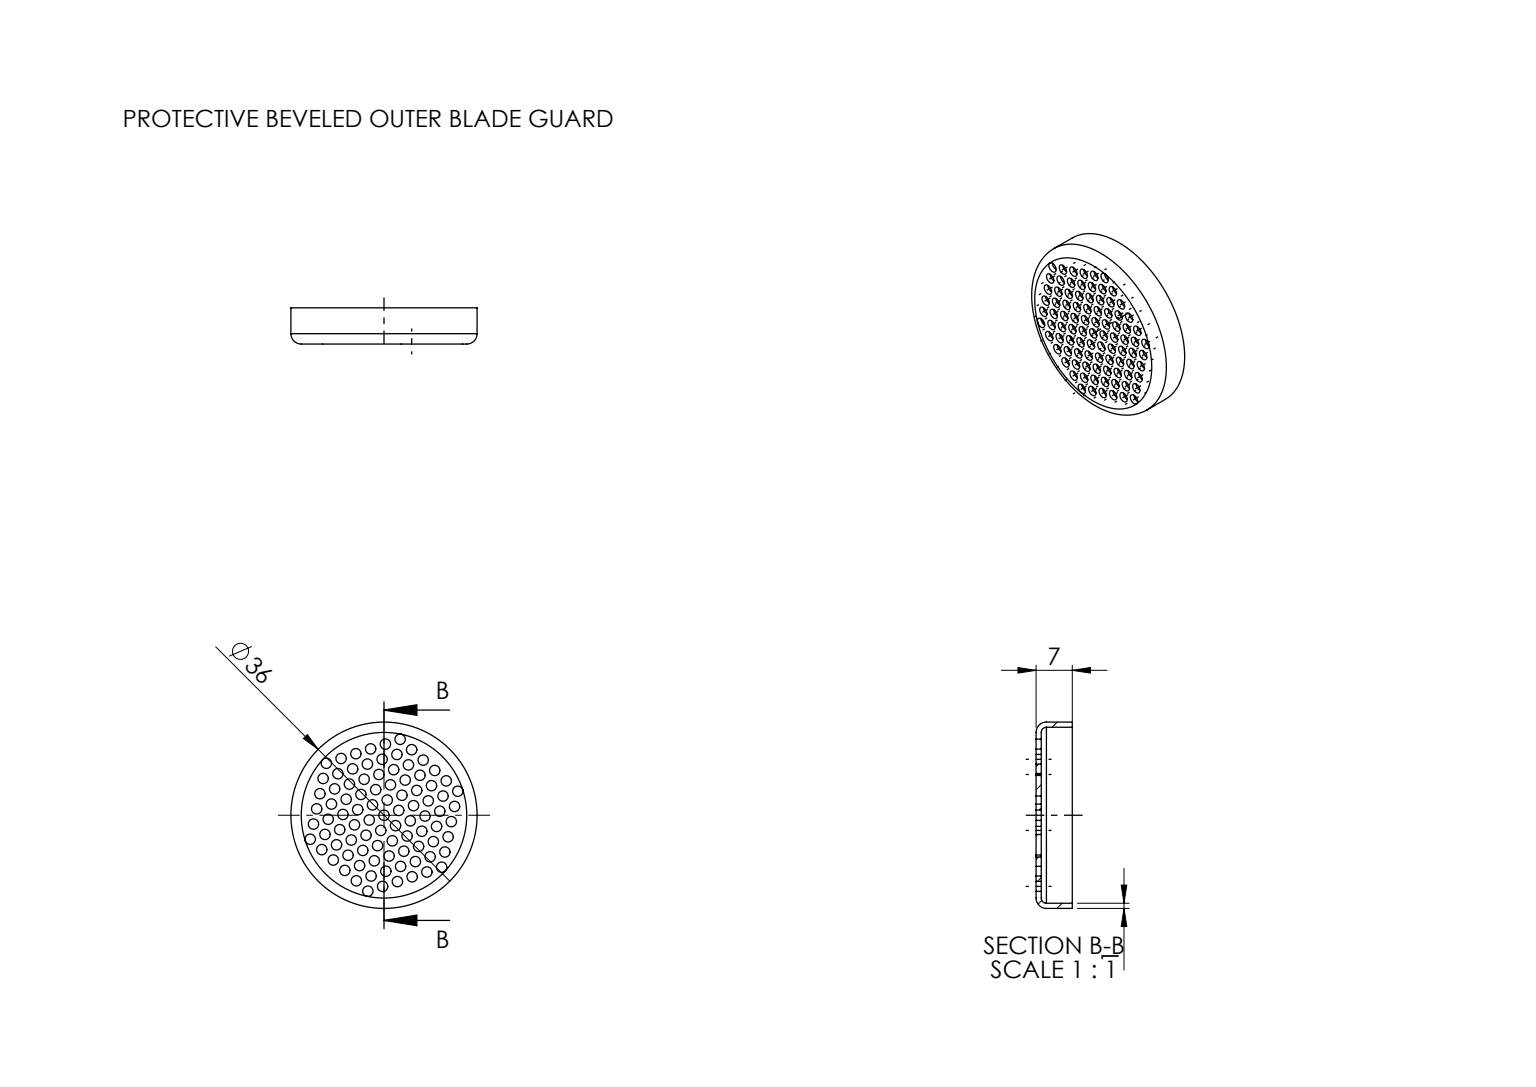
ISO-10303-21;
HEADER;
FILE_DESCRIPTION (('STEP AP214'),
    '1' );
FILE_NAME ('Protective Beveled Outer Blade Guard.step',
    '2026-10-04T08:29:30',
    ( '' ),
    ( '' ),
    'SwSTEP 2.0',
    'SolidWorks 2026',
    '' );
FILE_SCHEMA (( 'AUTOMOTIVE_DESIGN' ));
ENDSEC;

DATA;
#4=DIRECTION ( 'NONE',  ( 1.000000000000000000, 0.000000000000000000, 0.000000000000000000 ) ) ;
#5=CARTESIAN_POINT ( 'NONE',  ( 4.724371395536106633, 32.23037938972932892, 12.00000000000000000 ) ) ;
#7=VERTEX_POINT ( 'NONE', #23706 ) ;
#9=CYLINDRICAL_SURFACE ( 'NONE', #10255, 1.000000000000000000 ) ;
#10=DIRECTION ( 'NONE',  ( 1.000000000000000000, 0.000000000000000000, 0.000000000000000000 ) ) ;
#19=FACE_OUTER_BOUND ( 'NONE', #7772, .T. ) ;
#22=ORIENTED_EDGE ( 'NONE', *, *, #8423, .T. ) ;
#27=DIRECTION ( 'NONE',  ( 0.000000000000000000, 0.000000000000000000, 1.000000000000000000 ) ) ;
#33=CARTESIAN_POINT ( 'NONE',  ( -8.294006203984645609, 33.46401007850805343, 6.000000000000000000 ) ) ;
#34=ORIENTED_EDGE ( 'NONE', *, *, #3818, .T. ) ;
#39=CIRCLE ( 'NONE', #2001, 1.000000000000000000 ) ;
#40=DIRECTION ( 'NONE',  ( 1.000000000000000000, 0.000000000000000000, 0.000000000000000000 ) ) ;
#41=EDGE_LOOP ( 'NONE', ( #16818, #38380, #12394, #9835 ) ) ;
#54=DIRECTION ( 'NONE',  ( 0.000000000000000000, 0.000000000000000000, 1.000000000000000000 ) ) ;
#63=ORIENTED_EDGE ( 'NONE', *, *, #30537, .T. ) ;
#70=EDGE_CURVE ( 'NONE', #761, #15410, #872, .T. ) ;
#73=EDGE_CURVE ( 'NONE', #19744, #23095, #8006, .T. ) ;
#74=FACE_BOUND ( 'NONE', #6816, .T. ) ;
#78=DIRECTION ( 'NONE',  ( 0.000000000000000000, 0.000000000000000000, 1.000000000000000000 ) ) ;
#81=DIRECTION ( 'NONE',  ( 0.000000000000000000, 0.000000000000000000, 1.000000000000000000 ) ) ;
#83=ORIENTED_EDGE ( 'NONE', *, *, #31843, .F. ) ;
#90=ORIENTED_EDGE ( 'NONE', *, *, #14466, .T. ) ;
#91=DIRECTION ( 'NONE',  ( 1.000000000000000000, 0.000000000000000000, 0.000000000000000000 ) ) ;
#94=DIRECTION ( 'NONE',  ( 1.000000000000000000, 0.000000000000000000, 0.000000000000000000 ) ) ;
#105=CARTESIAN_POINT ( 'NONE',  ( 4.835130509701799362, 15.55077355964573904, 13.00000000000000178 ) ) ;
#107=DIRECTION ( 'NONE',  ( 1.000000000000000000, 0.000000000000000000, 0.000000000000000000 ) ) ;
#145=AXIS2_PLACEMENT_3D ( 'NONE', #32280, #11698, #11498 ) ;
#164=EDGE_CURVE ( 'NONE', #16334, #15391, #9293, .T. ) ;
#168=DIRECTION ( 'NONE',  ( 1.000000000000000000, 0.000000000000000000, 0.000000000000000000 ) ) ;
#169=EDGE_CURVE ( 'NONE', #13627, #24692, #9468, .T. ) ;
#175=DIRECTION ( 'NONE',  ( 1.000000000000000000, 0.000000000000000000, 0.000000000000000000 ) ) ;
#186=EDGE_CURVE ( 'NONE', #15751, #12988, #40137, .T. ) ;
#196=CIRCLE ( 'NONE', #16433, 1.000000000000000888 ) ;
#205=DIRECTION ( 'NONE',  ( 0.000000000000000000, 0.000000000000000000, 1.000000000000000000 ) ) ;
#206=DIRECTION ( 'NONE',  ( 0.000000000000000000, 0.000000000000000000, 1.000000000000000000 ) ) ;
#212=ORIENTED_EDGE ( 'NONE', *, *, #665, .T. ) ;
#223=ADVANCED_FACE ( 'NONE', ( #15359 ), #322, .F. ) ;
#230=DIRECTION ( 'NONE',  ( 0.000000000000000000, 0.000000000000000000, 1.000000000000000000 ) ) ;
#235=DIRECTION ( 'NONE',  ( 0.000000000000000000, 0.000000000000000000, 1.000000000000000000 ) ) ;
#237=EDGE_LOOP ( 'NONE', ( #9320, #17479 ) ) ;
#242=CARTESIAN_POINT ( 'NONE',  ( -7.559512017365658920, 19.71884705062586107, 13.00000000000000178 ) ) ;
#244=ORIENTED_EDGE ( 'NONE', *, *, #2667, .T. ) ;
#247=FACE_BOUND ( 'NONE', #237, .T. ) ;
#255=CARTESIAN_POINT ( 'NONE',  ( 5.100636323082810009, 29.29593658752792962, 6.000000000000000000 ) ) ;
#269=AXIS2_PLACEMENT_3D ( 'NONE', #36604, #30517, #27454 ) ;
#273=VECTOR ( 'NONE', #6219, 1000.000000000000000 ) ;
#274=FACE_BOUND ( 'NONE', #33600, .T. ) ;
#278=DIRECTION ( 'NONE',  ( 1.000000000000000000, 0.000000000000000000, 0.000000000000000000 ) ) ;
#292=ORIENTED_EDGE ( 'NONE', *, *, #22586, .T. ) ;
#304=DIRECTION ( 'NONE',  ( 0.000000000000000000, 0.000000000000000000, 1.000000000000000000 ) ) ;
#305=CARTESIAN_POINT ( 'NONE',  ( 9.541469607472739867, 17.40487552589537401, 13.00000000000000178 ) ) ;
#308=EDGE_LOOP ( 'NONE', ( #12738, #38655, #19382, #26352 ) ) ;
#313=ORIENTED_EDGE ( 'NONE', *, *, #4707, .F. ) ;
#314=CIRCLE ( 'NONE', #1622, 1.000000000000000888 ) ;
#317=CIRCLE ( 'NONE', #3523, 1.000000000000000000 ) ;
#318=EDGE_LOOP ( 'NONE', ( #14973, #38977, #20245, #19537 ) ) ;
#322=CYLINDRICAL_SURFACE ( 'NONE', #16452, 1.000000000000000000 ) ;
#325=CARTESIAN_POINT ( 'NONE',  ( -16.00000000000000000, 22.50000000000000711, 13.00000000000000178 ) ) ;
#327=CARTESIAN_POINT ( 'NONE',  ( 2.853166178176219425, 23.42705098312512746, 6.000000000000000000 ) ) ;
#329=DIRECTION ( 'NONE',  ( 0.000000000000000000, 0.000000000000000000, 1.000000000000000000 ) ) ;
#333=VERTEX_POINT ( 'NONE', #8869 ) ;
#337=EDGE_CURVE ( 'NONE', #7337, #4065, #33318, .T. ) ;
#342=VERTEX_POINT ( 'NONE', #31587 ) ;
#344=CARTESIAN_POINT ( 'NONE',  ( 1.247466774197339978, 28.36888560440311480, 12.00000000000000000 ) ) ;
#348=CIRCLE ( 'NONE', #38038, 1.000000000000000000 ) ;
#356=ORIENTED_EDGE ( 'NONE', *, *, #17824, .F. ) ;
#369=ORIENTED_EDGE ( 'NONE', *, *, #70, .F. ) ;
#370=EDGE_CURVE ( 'NONE', #7748, #33664, #16357, .T. ) ;
#372=CIRCLE ( 'NONE', #2976, 1.000000000000000000 ) ;
#376=FACE_OUTER_BOUND ( 'NONE', #28764, .T. ) ;
#382=CARTESIAN_POINT ( 'NONE',  ( -2.229437847141422679, 24.50739181907689712, 13.00000000000000178 ) ) ;
#389=CARTESIAN_POINT ( 'NONE',  ( 4.118671991557230072, 37.17221401100731981, 13.00000000000000178 ) ) ;
#404=CARTESIAN_POINT ( 'NONE',  ( -4.458872323573595864, 26.51478363815348160, 13.00000000000000178 ) ) ;
#405=AXIS2_PLACEMENT_3D ( 'NONE', #5623, #2190, #9079 ) ;
#406=VECTOR ( 'NONE', #32320, 1000.000000000000000 ) ;
#407=DIRECTION ( 'NONE',  ( 1.000000000000000000, 0.000000000000000000, 0.000000000000000000 ) ) ;
#418=ORIENTED_EDGE ( 'NONE', *, *, #17489, .F. ) ;
#420=DIRECTION ( 'NONE',  ( 0.000000000000000000, 0.000000000000000000, 1.000000000000000000 ) ) ;
#421=CARTESIAN_POINT ( 'NONE',  ( -7.330077540933487512, 17.71145523154927659, 6.000000000000000000 ) ) ;
#422=ADVANCED_FACE ( 'NONE', ( #9860 ), #3755, .F. ) ;
#426=CYLINDRICAL_SURFACE ( 'NONE', #11880, 1.000000000000000000 ) ;
#428=CARTESIAN_POINT ( 'NONE',  ( 4.100636323082810009, 29.29593658752792962, 12.00000000000000000 ) ) ;
#432=AXIS2_PLACEMENT_3D ( 'NONE', #3780, #28967, #7629 ) ;
#433=AXIS2_PLACEMENT_3D ( 'NONE', #15536, #27920, #20843 ) ;
#436=DIRECTION ( 'NONE',  ( 1.000000000000000000, 0.000000000000000000, 0.000000000000000000 ) ) ;
#443=FACE_OUTER_BOUND ( 'NONE', #7900, .T. ) ;
#453=DIRECTION ( 'NONE',  ( 1.000000000000000000, 0.000000000000000000, 0.000000000000000000 ) ) ;
#460=ORIENTED_EDGE ( 'NONE', *, *, #3040, .F. ) ;
#466=EDGE_CURVE ( 'NONE', #7227, #12151, #39815, .T. ) ;
#468=EDGE_CURVE ( 'NONE', #11093, #7792, #39183, .T. ) ;
#472=CYLINDRICAL_SURFACE ( 'NONE', #19490, 1.000000000000000888 ) ;
#473=FACE_BOUND ( 'NONE', #25651, .T. ) ;
#478=ADVANCED_FACE ( 'NONE', ( #13295 ), #25691, .F. ) ;
#488=VERTEX_POINT ( 'NONE', #16768 ) ;
#489=DIRECTION ( 'NONE',  ( 0.000000000000000000, 0.000000000000000000, 1.000000000000000000 ) ) ;
#495=DIRECTION ( 'NONE',  ( 0.000000000000000000, 0.000000000000000000, 1.000000000000000000 ) ) ;
#497=ORIENTED_EDGE ( 'NONE', *, *, #4457, .F. ) ;
#500=DIRECTION ( 'NONE',  ( 0.000000000000000000, 0.000000000000000000, 1.000000000000000000 ) ) ;
#502=ORIENTED_EDGE ( 'NONE', *, *, #14245, .T. ) ;
#507=ORIENTED_EDGE ( 'NONE', *, *, #21085, .T. ) ;
#516=ORIENTED_EDGE ( 'NONE', *, *, #20080, .F. ) ;
#525=DIRECTION ( 'NONE',  ( 1.000000000000000000, 0.000000000000000000, 0.000000000000000000 ) ) ;
#528=CARTESIAN_POINT ( 'NONE',  ( -6.688306800005769048, 28.52217545723006609, 12.00000000000000000 ) ) ;
#536=CYLINDRICAL_SURFACE ( 'NONE', #23712, 1.000000000000000888 ) ;
#539=ORIENTED_EDGE ( 'NONE', *, *, #1715, .F. ) ;
#548=ORIENTED_EDGE ( 'NONE', *, *, #9154, .F. ) ;
#555=AXIS2_PLACEMENT_3D ( 'NONE', #755, #4607, #4402 ) ;
#557=ORIENTED_EDGE ( 'NONE', *, *, #30997, .F. ) ;
#564=ORIENTED_EDGE ( 'NONE', *, *, #28279, .T. ) ;
#565=ORIENTED_EDGE ( 'NONE', *, *, #1592, .F. ) ;
#566=DIRECTION ( 'NONE',  ( 1.000000000000000000, 0.000000000000000000, 0.000000000000000000 ) ) ;
#567=DIRECTION ( 'NONE',  ( 0.000000000000000000, 0.000000000000000000, 1.000000000000000000 ) ) ;
#569=CYLINDRICAL_SURFACE ( 'NONE', #4551, 1.000000000000000000 ) ;
#575=EDGE_CURVE ( 'NONE', #17675, #5736, #23614, .T. ) ;
#577=LINE ( 'NONE', #40192, #36421 ) ;
#579=CARTESIAN_POINT ( 'NONE',  ( 4.100636323082810009, 29.29593658752792962, 12.00000000000000000 ) ) ;
#581=EDGE_LOOP ( 'NONE', ( #27282, #21112 ) ) ;
#600=VECTOR ( 'NONE', #21084, 1000.000000000000000 ) ;
#601=CIRCLE ( 'NONE', #23310, 1.000000000000000888 ) ;
#605=DIRECTION ( 'NONE',  ( 0.000000000000000000, 0.000000000000000000, 1.000000000000000000 ) ) ;
#607=CIRCLE ( 'NONE', #22659, 16.00000000000000000 ) ;
#609=ORIENTED_EDGE ( 'NONE', *, *, #7426, .F. ) ;
#618=EDGE_CURVE ( 'NONE', #36861, #8408, #24252, .T. ) ;
#622=DIRECTION ( 'NONE',  ( 0.000000000000000000, 0.000000000000000000, 1.000000000000000000 ) ) ;
#624=DIRECTION ( 'NONE',  ( 1.000000000000000000, 0.000000000000000000, 0.000000000000000000 ) ) ;
#625=CARTESIAN_POINT ( 'NONE',  ( 8.577540944421576441, 33.15743037285414374, 6.000000000000000000 ) ) ;
#632=VECTOR ( 'NONE', #12558, 1000.000000000000000 ) ;
#633=DIRECTION ( 'NONE',  ( 0.000000000000000000, 0.000000000000000000, 1.000000000000000000 ) ) ;
#634=VERTEX_POINT ( 'NONE', #17175 ) ;
#638=DIRECTION ( 'NONE',  ( 0.000000000000000000, 0.000000000000000000, 1.000000000000000000 ) ) ;
#641=ORIENTED_EDGE ( 'NONE', *, *, #9085, .F. ) ;
#644=FACE_BOUND ( 'NONE', #39612, .T. ) ;
#650=CARTESIAN_POINT ( 'NONE',  ( 5.064564986133971658, 13.54338174056915456, 6.000000000000000000 ) ) ;
#657=CYLINDRICAL_SURFACE ( 'NONE', #27165, 1.000000000000000888 ) ;
#664=CARTESIAN_POINT ( 'NONE',  ( 5.706335727061685681, 24.35410196624994583, 13.00000000000000178 ) ) ;
#665=EDGE_CURVE ( 'NONE', #36376, #19095, #908, .T. ) ;
#668=EDGE_CURVE ( 'NONE', #29140, #10198, #27105, .T. ) ;
#673=CARTESIAN_POINT ( 'NONE',  ( -0.01803903918367114056, 14.62372257652092422, 6.000000000000000000 ) ) ;
#682=CYLINDRICAL_SURFACE ( 'NONE', #22242, 1.000000000000000000 ) ;
#683=EDGE_CURVE ( 'NONE', #5931, #35634, #37212, .T. ) ;
#684=CIRCLE ( 'NONE', #18216, 1.000000000000000000 ) ;
#692=ORIENTED_EDGE ( 'NONE', *, *, #14157, .F. ) ;
#695=CARTESIAN_POINT ( 'NONE',  ( -3.458872323573595864, 26.51478363815348160, 13.00000000000000178 ) ) ;
#697=VERTEX_POINT ( 'NONE', #5170 ) ;
#699=CARTESIAN_POINT ( 'NONE',  ( 6.064564986133971658, 13.54338174056915456, 6.000000000000000000 ) ) ;
#708=VERTEX_POINT ( 'NONE', #2331 ) ;
#711=CARTESIAN_POINT ( 'NONE',  ( -3.118678732975735279, 7.827785988993307242, 13.00000000000000178 ) ) ;
#719=LINE ( 'NONE', #37295, #34101 ) ;
#720=ORIENTED_EDGE ( 'NONE', *, *, #23187, .T. ) ;
#730=AXIS2_PLACEMENT_3D ( 'NONE', #39640, #18124, #33167 ) ;
#732=DIRECTION ( 'NONE',  ( 1.000000000000000000, 0.000000000000000000, 0.000000000000000000 ) ) ;
#755=CARTESIAN_POINT ( 'NONE',  ( -14.26585111513660031, 17.86474508437623143, 13.00000000000000178 ) ) ;
#761=VERTEX_POINT ( 'NONE', #35848 ) ;
#775=DIRECTION ( 'NONE',  ( 0.000000000000000000, 0.000000000000000000, 1.000000000000000000 ) ) ;
#776=ORIENTED_EDGE ( 'NONE', *, *, #24265, .T. ) ;
#801=ADVANCED_FACE ( 'NONE', ( #34005 ), #24850, .F. ) ;
#808=AXIS2_PLACEMENT_3D ( 'NONE', #20811, #5557, #5361 ) ;
#810=SHAPE_DEFINITION_REPRESENTATION ( #13590, #33787 ) ;
#812=DIRECTION ( 'NONE',  ( 0.000000000000000000, 0.000000000000000000, 1.000000000000000000 ) ) ;
#820=DIRECTION ( 'NONE',  ( 0.000000000000000000, 0.000000000000000000, 1.000000000000000000 ) ) ;
#826=ORIENTED_EDGE ( 'NONE', *, *, #18908, .F. ) ;
#827=CIRCLE ( 'NONE', #29361, 1.000000000000000000 ) ;
#829=CARTESIAN_POINT ( 'NONE',  ( 8.293999462566144842, 11.53598992149257008, 12.00000000000000000 ) ) ;
#831=ORIENTED_EDGE ( 'NONE', *, *, #16332, .F. ) ;
#833=AXIS2_PLACEMENT_3D ( 'NONE', #38271, #31970, #16136 ) ;
#839=VERTEX_POINT ( 'NONE', #14916 ) ;
#843=AXIS2_PLACEMENT_3D ( 'NONE', #11726, #1991, #14371 ) ;
#844=FACE_BOUND ( 'NONE', #6698, .T. ) ;
#857=AXIS2_PLACEMENT_3D ( 'NONE', #18083, #5474, #30473 ) ;
#858=DIRECTION ( 'NONE',  ( 0.000000000000000000, 0.000000000000000000, 1.000000000000000000 ) ) ;
#867=EDGE_CURVE ( 'NONE', #37025, #33408, #28133, .T. ) ;
#869=ADVANCED_FACE ( 'NONE', ( #39494, #24256, #11671, #27502, #8821, #24652, #5564, #24058, #21208, #2722, #33618, #9020, #5768, #21014, #33423, #12264, #33812, #5960, #30362, #2529, #74, #27898, #21601, #27305, #30562, #37046, #18364, #30759, #15112, #39885, #12458, #12062, #2921, #9216, #15309, #30951, #3119, #15516, #34795, #25845, #35195, #3910, #6749, #25251, #38246, #22595, #6945, #10414, #9622, #31749, #22796, #38041, #9816, #28297, #13251, #25642, #37837, #3515, #7353, #22002, #19757, #32155, #34401, #28693, #13048, #25438, #4315, #28094, #28899, #473, #15912, #871, #31545, #274, #19352, #22392, #16310, #12659, #25051, #35004, #12856, #37646, #37445, #7153, #10210, #6552 ), #19551, .F. ) ;
#871=FACE_BOUND ( 'NONE', #16938, .T. ) ;
#872=CIRCLE ( 'NONE', #33967, 1.000000000000000000 ) ;
#880=VERTEX_POINT ( 'NONE', #4109 ) ;
#883=CARTESIAN_POINT ( 'NONE',  ( -2.229437847141422679, 24.50739181907689712, 12.00000000000000000 ) ) ;
#885=ORIENTED_EDGE ( 'NONE', *, *, #33735, .F. ) ;
#888=VERTEX_POINT ( 'NONE', #16516 ) ;
#890=CARTESIAN_POINT ( 'NONE',  ( -2.211402178667006169, 32.38366924255629442, 6.000000000000000000 ) ) ;
#893=CYLINDRICAL_SURFACE ( 'NONE', #39346, 1.000000000000000888 ) ;
#894=CIRCLE ( 'NONE', #2839, 1.000000000000000000 ) ;
#900=ORIENTED_EDGE ( 'NONE', *, *, #18324, .F. ) ;
#904=ORIENTED_EDGE ( 'NONE', *, *, #35439, .F. ) ;
#908=CIRCLE ( 'NONE', #24889, 1.000000000000000000 ) ;
#912=CIRCLE ( 'NONE', #27540, 1.000000000000000888 ) ;
#919=DIRECTION ( 'NONE',  ( 0.000000000000000000, 0.000000000000000000, 1.000000000000000000 ) ) ;
#921=EDGE_LOOP ( 'NONE', ( #7988, #20870 ) ) ;
#922=CARTESIAN_POINT ( 'NONE',  ( 5.724371395536106633, 32.23037938972932892, 13.00000000000000178 ) ) ;
#925=DIRECTION ( 'NONE',  ( 1.000000000000000000, 0.000000000000000000, 0.000000000000000000 ) ) ;
#956=VECTOR ( 'NONE', #36154, 1000.000000000000000 ) ;
#961=DIRECTION ( 'NONE',  ( 0.000000000000000000, 0.000000000000000000, 1.000000000000000000 ) ) ;
#972=ORIENTED_EDGE ( 'NONE', *, *, #34521, .F. ) ;
#974=CARTESIAN_POINT ( 'NONE',  ( -15.21736038221435727, 17.55712500267617315, 13.00000000000000178 ) ) ;
#976=STYLED_ITEM ( 'NONE', ( #32825 ), #34952 ) ;
#977=CARTESIAN_POINT ( 'NONE',  ( 13.03640989728592459, 29.14264673470096767, 13.00000000000000178 ) ) ;
#978=FACE_OUTER_BOUND ( 'NONE', #35617, .T. ) ;
#986=DIRECTION ( 'NONE',  ( 0.000000000000000000, 0.000000000000000000, 1.000000000000000000 ) ) ;
#991=LINE ( 'NONE', #7683, #5762 ) ;
#999=DIRECTION ( 'NONE',  ( 0.000000000000000000, 0.000000000000000000, 1.000000000000000000 ) ) ;
#1000=ORIENTED_EDGE ( 'NONE', *, *, #15480, .F. ) ;
#1008=ORIENTED_EDGE ( 'NONE', *, *, #2242, .F. ) ;
#1014=CIRCLE ( 'NONE', #6200, 1.000000000000000000 ) ;
#1017=PRODUCT_CONTEXT ( 'NONE', #21521, 'mechanical' ) ;
#1031=DIRECTION ( 'NONE',  ( 0.000000000000000000, 0.000000000000000000, 1.000000000000000000 ) ) ;
#1039=CIRCLE ( 'NONE', #14000, 1.000000000000000000 ) ;
#1042=AXIS2_PLACEMENT_3D ( 'NONE', #7873, #10730, #26571 ) ;
#1047=DIRECTION ( 'NONE',  ( 0.000000000000000000, 0.000000000000000000, 1.000000000000000000 ) ) ;
#1051=ORIENTED_EDGE ( 'NONE', *, *, #1452, .F. ) ;
#1053=CYLINDRICAL_SURFACE ( 'NONE', #33678, 1.000000000000000000 ) ;
#1054=CARTESIAN_POINT ( 'NONE',  ( -4.835137251120299240, 29.44922644035488446, 12.00000000000000000 ) ) ;
#1063=ORIENTED_EDGE ( 'NONE', *, *, #14261, .T. ) ;
#1066=CARTESIAN_POINT ( 'NONE',  ( -5.706342468480190000, 20.64589803375067945, 6.000000000000000000 ) ) ;
#1069=DIRECTION ( 'NONE',  ( 0.000000000000000000, 0.000000000000000000, 1.000000000000000000 ) ) ;
#1072=DIRECTION ( 'NONE',  ( 1.000000000000000000, 0.000000000000000000, 0.000000000000000000 ) ) ;
#1074=EDGE_CURVE ( 'NONE', #24243, #2749, #16921, .T. ) ;
#1076=ADVANCED_FACE ( 'NONE', ( #32767 ), #16717, .F. ) ;
#1079=ADVANCED_FACE ( 'NONE', ( #23613 ), #35403, .F. ) ;
#1081=CARTESIAN_POINT ( 'NONE',  ( 3.100636323082810009, 29.29593658752792962, 12.00000000000000000 ) ) ;
#1091=CARTESIAN_POINT ( 'NONE',  ( -3.211402178667006169, 32.38366924255629442, 13.00000000000000178 ) ) ;
#1103=ORIENTED_EDGE ( 'NONE', *, *, #25798, .F. ) ;
#1105=DIRECTION ( 'NONE',  ( 1.000000000000000000, 0.000000000000000000, 0.000000000000000000 ) ) ;
#1107=CARTESIAN_POINT ( 'NONE',  ( 0.3582258883630317636, 11.68927977431952137, 13.00000000000000178 ) ) ;
#1116=DIRECTION ( 'NONE',  ( 0.000000000000000000, 0.000000000000000000, 1.000000000000000000 ) ) ;
#1117=CYLINDRICAL_SURFACE ( 'NONE', #37924, 1.000000000000000000 ) ;
#1125=CARTESIAN_POINT ( 'NONE',  ( 0.9819609608163288872, 14.62372257652092422, 12.00000000000000000 ) ) ;
#1127=CIRCLE ( 'NONE', #32283, 1.000000000000000000 ) ;
#1149=ORIENTED_EDGE ( 'NONE', *, *, #8604, .F. ) ;
#1174=DIRECTION ( 'NONE',  ( 1.000000000000000000, 0.000000000000000000, 0.000000000000000000 ) ) ;
#1175=DIRECTION ( 'NONE',  ( 0.000000000000000000, 0.000000000000000000, 1.000000000000000000 ) ) ;
#1180=DIRECTION ( 'NONE',  ( 0.000000000000000000, 0.000000000000000000, 1.000000000000000000 ) ) ;
#1207=ORIENTED_EDGE ( 'NONE', *, *, #7249, .F. ) ;
#1213=EDGE_LOOP ( 'NONE', ( #29735, #21723 ) ) ;
#1216=AXIS2_PLACEMENT_3D ( 'NONE', #39023, #17309, #17711 ) ;
#1217=ORIENTED_EDGE ( 'NONE', *, *, #3052, .T. ) ;
#1220=CIRCLE ( 'NONE', #11606, 1.000000000000000000 ) ;
#1223=EDGE_CURVE ( 'NONE', #12698, #32913, #15840, .T. ) ;
#1226=EDGE_LOOP ( 'NONE', ( #7696, #31771 ) ) ;
#1228=DIRECTION ( 'NONE',  ( 0.000000000000000000, 0.000000000000000000, 1.000000000000000000 ) ) ;
#1229=FACE_OUTER_BOUND ( 'NONE', #33630, .T. ) ;
#1234=CARTESIAN_POINT ( 'NONE',  ( 1.494936919103933226, 34.23777120880591696, 6.000000000000000000 ) ) ;
#1240=ORIENTED_EDGE ( 'NONE', *, *, #8680, .T. ) ;
#1248=AXIS2_PLACEMENT_3D ( 'NONE', #664, #24648, #15512 ) ;
#1251=DIRECTION ( 'NONE',  ( 0.000000000000000000, 0.000000000000000000, 1.000000000000000000 ) ) ;
#1258=VERTEX_POINT ( 'NONE', #22299 ) ;
#1261=VERTEX_POINT ( 'NONE', #5321 ) ;
#1270=AXIS2_PLACEMENT_3D ( 'NONE', #37696, #19009, #9864 ) ;
#1275=DIRECTION ( 'NONE',  ( 0.000000000000000000, 0.000000000000000000, 1.000000000000000000 ) ) ;
#1287=ORIENTED_EDGE ( 'NONE', *, *, #18070, .T. ) ;
#1289=DIRECTION ( 'NONE',  ( 1.000000000000000000, 0.000000000000000000, 0.000000000000000000 ) ) ;
#1295=VECTOR ( 'NONE', #26003, 1000.000000000000000 ) ;
#1307=ORIENTED_EDGE ( 'NONE', *, *, #32309, .T. ) ;
#1310=ADVANCED_FACE ( 'NONE', ( #21162 ), #12761, .F. ) ;
#1313=EDGE_CURVE ( 'NONE', #6680, #2398, #15203, .T. ) ;
#1315=DIRECTION ( 'NONE',  ( 0.000000000000000000, 0.000000000000000000, 1.000000000000000000 ) ) ;
#1317=CARTESIAN_POINT ( 'NONE',  ( 5.458865582155095986, 18.48521636184714012, 12.00000000000000000 ) ) ;
#1324=EDGE_CURVE ( 'NONE', #26783, #13841, #26857, .T. ) ;
#1339=ORIENTED_EDGE ( 'NONE', *, *, #20945, .T. ) ;
#1350=CIRCLE ( 'NONE', #6519, 1.000000000000000888 ) ;
#1354=ORIENTED_EDGE ( 'NONE', *, *, #29827, .T. ) ;
#1356=ADVANCED_FACE ( 'NONE', ( #5514 ), #24009, .F. ) ;
#1358=EDGE_LOOP ( 'NONE', ( #33756, #22693 ) ) ;
#1361=AXIS2_PLACEMENT_3D ( 'NONE', #24804, #28254, #12412 ) ;
#1366=CARTESIAN_POINT ( 'NONE',  ( -18.00000000000000000, 22.50000000000000355, 6.000000000000000000 ) ) ;
#1367=LINE ( 'NONE', #10306, #8481 ) ;
#1376=EDGE_CURVE ( 'NONE', #18785, #40077, #26215, .T. ) ;
#1377=LINE ( 'NONE', #35710, #25357 ) ;
#1384=CARTESIAN_POINT ( 'NONE',  ( -4.118678732975735279, 7.827785988993307242, 6.000000000000000000 ) ) ;
#1396=CYLINDRICAL_SURFACE ( 'NONE', #2758, 1.000000000000000000 ) ;
#1409=ORIENTED_EDGE ( 'NONE', *, *, #22300, .F. ) ;
#1414=ORIENTED_EDGE ( 'NONE', *, *, #34847, .F. ) ;
#1419=CARTESIAN_POINT ( 'NONE',  ( 11.14716901145161643, 12.46304090461738667, 12.00000000000000000 ) ) ;
#1422=ORIENTED_EDGE ( 'NONE', *, *, #35439, .T. ) ;
#1423=LINE ( 'NONE', #23757, #26238 ) ;
#1425=EDGE_CURVE ( 'NONE', #29377, #5003, #4219, .T. ) ;
#1442=ORIENTED_EDGE ( 'NONE', *, *, #468, .T. ) ;
#1452=EDGE_CURVE ( 'NONE', #21094, #16360, #1581, .T. ) ;
#1453=DIRECTION ( 'NONE',  ( 0.000000000000000000, 0.000000000000000000, 1.000000000000000000 ) ) ;
#1454=CARTESIAN_POINT ( 'NONE',  ( 4.724371395536106633, 32.23037938972932892, 6.000000000000000000 ) ) ;
#1468=CARTESIAN_POINT ( 'NONE',  ( 16.00000000000000000, 22.50000000000000355, 12.00000000000000000 ) ) ;
#1472=CARTESIAN_POINT ( 'NONE',  ( 7.312035131040564906, 19.41226734497195849, 6.000000000000000000 ) ) ;
#1476=CIRCLE ( 'NONE', #24180, 1.000000000000000888 ) ;
#1493=DIRECTION ( 'NONE',  ( 1.000000000000000000, 0.000000000000000000, 0.000000000000000000 ) ) ;
#1495=DIRECTION ( 'NONE',  ( 0.000000000000000000, 0.000000000000000000, 1.000000000000000000 ) ) ;
#1504=ADVANCED_FACE ( 'NONE', ( #978 ), #10721, .F. ) ;
#1516=CARTESIAN_POINT ( 'NONE',  ( 0.8712018466506370462, 31.30332840660451765, 12.00000000000000000 ) ) ;
#1518=CARTESIAN_POINT ( 'NONE',  ( -7.688306800005769048, 28.52217545723006609, 12.00000000000000000 ) ) ;
#1519=CIRCLE ( 'NONE', #11910, 1.000000000000000000 ) ;
#1520=DIRECTION ( 'NONE',  ( 0.000000000000000000, 0.000000000000000000, 1.000000000000000000 ) ) ;
#1523=EDGE_CURVE ( 'NONE', #36376, #3606, #10317, .T. ) ;
#1525=CARTESIAN_POINT ( 'NONE',  ( -9.183247089818959097, 16.78440424842446532, 12.00000000000000000 ) ) ;
#1527=DIRECTION ( 'NONE',  ( 1.000000000000000000, 0.000000000000000000, 0.000000000000000000 ) ) ;
#1529=EDGE_CURVE ( 'NONE', #14246, #20723, #19724, .T. ) ;
#1531=CARTESIAN_POINT ( 'NONE',  ( 14.64210930126480115, 24.20081211342298744, 6.000000000000000000 ) ) ;
#1535=CIRCLE ( 'NONE', #24899, 1.000000000000000000 ) ;
#1553=VERTEX_POINT ( 'NONE', #25546 ) ;
#1555=CARTESIAN_POINT ( 'NONE',  ( 8.559505275947156377, 25.28115294937476065, 12.00000000000000000 ) ) ;
#1557=DIRECTION ( 'NONE',  ( 1.000000000000000000, 0.000000000000000000, 0.000000000000000000 ) ) ;
#1558=EDGE_LOOP ( 'NONE', ( #20598, #31967, #32905, #25702 ) ) ;
#1564=CARTESIAN_POINT ( 'NONE',  ( -8.577547685840080760, 11.84256962714647798, 6.000000000000000000 ) ) ;
#1573=CARTESIAN_POINT ( 'NONE',  ( 7.577540944421576441, 33.15743037285414374, 6.000000000000000000 ) ) ;
#1577=EDGE_CURVE ( 'NONE', #32176, #28480, #7460, .T. ) ;
#1581=LINE ( 'NONE', #23108, #4820 ) ;
#1582=CARTESIAN_POINT ( 'NONE',  ( -14.26585111513660031, 17.86474508437623143, 6.000000000000000000 ) ) ;
#1589=EDGE_CURVE ( 'NONE', #2436, #14685, #14573, .T. ) ;
#1590=DIRECTION ( 'NONE',  ( 0.000000000000000000, 0.000000000000000000, 1.000000000000000000 ) ) ;
#1592=EDGE_CURVE ( 'NONE', #35323, #33546, #6114, .T. ) ;
#1597=AXIS2_PLACEMENT_3D ( 'NONE', #38393, #1228, #29449 ) ;
#1602=CARTESIAN_POINT ( 'NONE',  ( -8.183247089818959097, 16.78440424842446532, 6.000000000000000000 ) ) ;
#1603=ORIENTED_EDGE ( 'NONE', *, *, #27527, .F. ) ;
#1607=ORIENTED_EDGE ( 'NONE', *, *, #31486, .F. ) ;
#1610=DIRECTION ( 'NONE',  ( 0.000000000000000000, 0.000000000000000000, 1.000000000000000000 ) ) ;
#1612=EDGE_LOOP ( 'NONE', ( #18659, #38492 ) ) ;
#1614=VERTEX_POINT ( 'NONE', #23318 ) ;
#1619=CARTESIAN_POINT ( 'NONE',  ( 6.330070799514983193, 27.28854476845134513, 13.00000000000000178 ) ) ;
#1621=DIRECTION ( 'NONE',  ( 0.000000000000000000, 0.000000000000000000, 1.000000000000000000 ) ) ;
#1622=AXIS2_PLACEMENT_3D ( 'NONE', #1740, #25900, #10676 ) ;
#1634=ORIENTED_EDGE ( 'NONE', *, *, #8604, .T. ) ;
#1640=CIRCLE ( 'NONE', #12654, 1.000000000000000000 ) ;
#1641=ORIENTED_EDGE ( 'NONE', *, *, #34748, .T. ) ;
#1646=VERTEX_POINT ( 'NONE', #32871 ) ;
#1647=ORIENTED_EDGE ( 'NONE', *, *, #28867, .T. ) ;
#1649=AXIS2_PLACEMENT_3D ( 'NONE', #3131, #12277, #15528 ) ;
#1650=CARTESIAN_POINT ( 'NONE',  ( 7.688300058587269170, 16.47782454277055564, 6.000000000000000000 ) ) ;
#1651=PLANE ( 'NONE',  #26970 ) ;
#1654=AXIS2_PLACEMENT_3D ( 'NONE', #13831, #38417, #10389 ) ;
#1665=EDGE_CURVE ( 'NONE', #12491, #1261, #14472, .T. ) ;
#1673=FACE_OUTER_BOUND ( 'NONE', #30728, .T. ) ;
#1675=CARTESIAN_POINT ( 'NONE',  ( 3.211395437248501850, 12.61633075744433796, 13.00000000000000178 ) ) ;
#1678=CIRCLE ( 'NONE', #6845, 1.000000000000000000 ) ;
#1685=DIRECTION ( 'NONE',  ( 0.000000000000000000, 0.000000000000000000, 1.000000000000000000 ) ) ;
#1690=VERTEX_POINT ( 'NONE', #18029 ) ;
#1694=DIRECTION ( 'NONE',  ( 0.000000000000000000, 0.000000000000000000, 1.000000000000000000 ) ) ;
#1708=ORIENTED_EDGE ( 'NONE', *, *, #26546, .T. ) ;
#1710=DIRECTION ( 'NONE',  ( 0.000000000000000000, 0.000000000000000000, 1.000000000000000000 ) ) ;
#1714=ORIENTED_EDGE ( 'NONE', *, *, #9208, .T. ) ;
#1715=EDGE_CURVE ( 'NONE', #40077, #18785, #11904, .T. ) ;
#1727=EDGE_CURVE ( 'NONE', #14625, #5931, #1784, .T. ) ;
#1731=DIRECTION ( 'NONE',  ( 0.000000000000000000, 0.000000000000000000, 1.000000000000000000 ) ) ;
#1735=DIRECTION ( 'NONE',  ( 0.000000000000000000, 0.000000000000000000, 1.000000000000000000 ) ) ;
#1740=CARTESIAN_POINT ( 'NONE',  ( 8.559505275947156377, 25.28115294937476065, 12.00000000000000000 ) ) ;
#1741=ORIENTED_EDGE ( 'NONE', *, *, #23042, .T. ) ;
#1750=ORIENTED_EDGE ( 'NONE', *, *, #3369, .F. ) ;
#1758=ORIENTED_EDGE ( 'NONE', *, *, #12792, .T. ) ;
#1762=DIRECTION ( 'NONE',  ( 1.000000000000000000, 0.000000000000000000, 0.000000000000000000 ) ) ;
#1768=EDGE_CURVE ( 'NONE', #8057, #24946, #11230, .T. ) ;
#1772=CIRCLE ( 'NONE', #4980, 1.000000000000000888 ) ;
#1775=DIRECTION ( 'NONE',  ( 1.000000000000000000, 0.000000000000000000, 0.000000000000000000 ) ) ;
#1776=AXIS2_PLACEMENT_3D ( 'NONE', #39774, #14803, #20706 ) ;
#1777=CIRCLE ( 'NONE', #28349, 1.000000000000000888 ) ;
#1781=CARTESIAN_POINT ( 'NONE',  ( 6.953805871968278929, 30.22298757065274444, 13.00000000000000178 ) ) ;
#1784=LINE ( 'NONE', #30215, #4083 ) ;
#1785=CARTESIAN_POINT ( 'NONE',  ( 5.348106467989403257, 35.16482219193073178, 12.00000000000000000 ) ) ;
#1798=CIRCLE ( 'NONE', #30361, 1.000000000000000000 ) ;
#1808=EDGE_LOOP ( 'NONE', ( #37828, #25664 ) ) ;
#1815=EDGE_LOOP ( 'NONE', ( #20216, #34 ) ) ;
#1821=ORIENTED_EDGE ( 'NONE', *, *, #14362, .F. ) ;
#1825=EDGE_CURVE ( 'NONE', #3811, #17784, #36546, .T. ) ;
#1826=CIRCLE ( 'NONE', #36844, 1.000000000000000000 ) ;
#1827=CARTESIAN_POINT ( 'NONE',  ( 0.7344908159097338629, 8.754836972118123839, 13.00000000000000178 ) ) ;
#1828=CARTESIAN_POINT ( 'NONE',  ( 1.853166178176219203, 23.42705098312512746, 13.00000000000000178 ) ) ;
#1833=ORIENTED_EDGE ( 'NONE', *, *, #7795, .F. ) ;
#1839=AXIS2_PLACEMENT_3D ( 'NONE', #33935, #205, #34531 ) ;
#1841=VERTEX_POINT ( 'NONE', #18819 ) ;
#1857=FACE_BOUND ( 'NONE', #16912, .T. ) ;
#1864=DIRECTION ( 'NONE',  ( 1.000000000000000000, 0.000000000000000000, 0.000000000000000000 ) ) ;
#1871=DIRECTION ( 'NONE',  ( 0.000000000000000000, 0.000000000000000000, 1.000000000000000000 ) ) ;
#1881=DIRECTION ( 'NONE',  ( 1.000000000000000000, 0.000000000000000000, 0.000000000000000000 ) ) ;
#1889=EDGE_CURVE ( 'NONE', #33038, #25337, #3370, .T. ) ;
#1892=AXIS2_PLACEMENT_3D ( 'NONE', #20958, #2671, #33765 ) ;
#1894=CARTESIAN_POINT ( 'NONE',  ( -9.183247089818959097, 16.78440424842446532, 6.000000000000000000 ) ) ;
#1900=DIRECTION ( 'NONE',  ( 0.000000000000000000, 0.000000000000000000, 1.000000000000000000 ) ) ;
#1902=EDGE_LOOP ( 'NONE', ( #18747, #37802, #33933, #21876 ) ) ;
#1916=DIRECTION ( 'NONE',  ( 0.000000000000000000, 0.000000000000000000, 1.000000000000000000 ) ) ;
#1927=AXIS2_PLACEMENT_3D ( 'NONE', #24798, #2870, #6697 ) ;
#1931=CARTESIAN_POINT ( 'NONE',  ( 0.2655024426717602637, 36.24516302788250499, 13.00000000000000178 ) ) ;
#1933=DIRECTION ( 'NONE',  ( 0.000000000000000000, 0.000000000000000000, 1.000000000000000000 ) ) ;
#1937=LINE ( 'NONE', #39095, #9264 ) ;
#1938=CARTESIAN_POINT ( 'NONE',  ( 9.293999462566146619, 11.53598992149257008, 6.000000000000000000 ) ) ;
#1940=ADVANCED_FACE ( 'NONE', ( #3569 ), #9076, .F. ) ;
#1943=DIRECTION ( 'NONE',  ( 0.000000000000000000, 0.000000000000000000, 1.000000000000000000 ) ) ;
#1944=EDGE_CURVE ( 'NONE', #30326, #6441, #36712, .T. ) ;
#1959=CYLINDRICAL_SURFACE ( 'NONE', #39979, 1.000000000000000000 ) ;
#1981=CARTESIAN_POINT ( 'NONE',  ( 4.724371395536106633, 32.23037938972932892, 6.000000000000000000 ) ) ;
#1983=AXIS2_PLACEMENT_3D ( 'NONE', #5219, #17631, #8670 ) ;
#1988=CARTESIAN_POINT ( 'NONE',  ( 3.211395437248501850, 12.61633075744433796, 6.000000000000000000 ) ) ;
#1991=DIRECTION ( 'NONE',  ( 0.000000000000000000, 0.000000000000000000, 1.000000000000000000 ) ) ;
#2001=AXIS2_PLACEMENT_3D ( 'NONE', #13298, #25694, #10874 ) ;
#2006=DIRECTION ( 'NONE',  ( 1.000000000000000000, 0.000000000000000000, 0.000000000000000000 ) ) ;
#2011=CARTESIAN_POINT ( 'NONE',  ( 3.853166178176219425, 23.42705098312512746, 6.000000000000000000 ) ) ;
#2013=AXIS2_PLACEMENT_3D ( 'NONE', #25802, #19709, #38198 ) ;
#2016=DIRECTION ( 'NONE',  ( 1.000000000000000000, 0.000000000000000000, 0.000000000000000000 ) ) ;
#2026=ORIENTED_EDGE ( 'NONE', *, *, #23863, .F. ) ;
#2030=CARTESIAN_POINT ( 'NONE',  ( 4.458865582155095986, 18.48521636184714012, 12.00000000000000000 ) ) ;
#2033=VERTEX_POINT ( 'NONE', #13103 ) ;
#2034=LINE ( 'NONE', #14414, #10664 ) ;
#2035=CARTESIAN_POINT ( 'NONE',  ( 1.358225888363031819, 11.68927977431952137, 12.00000000000000000 ) ) ;
#2036=VECTOR ( 'NONE', #34902, 1000.000000000000000 ) ;
#2037=CARTESIAN_POINT ( 'NONE',  ( -2.476907992048017260, 18.63850621467409496, 12.00000000000000000 ) ) ;
#2048=AXIS2_PLACEMENT_3D ( 'NONE', #20521, #26604, #7914 ) ;
#2051=AXIS2_PLACEMENT_3D ( 'NONE', #11019, #19958, #38239 ) ;
#2055=ORIENTED_EDGE ( 'NONE', *, *, #14868, .F. ) ;
#2060=ORIENTED_EDGE ( 'NONE', *, *, #13963, .T. ) ;
#2063=LINE ( 'NONE', #39421, #12227 ) ;
#2064=AXIS2_PLACEMENT_3D ( 'NONE', #10796, #29875, #26226 ) ;
#2066=ORIENTED_EDGE ( 'NONE', *, *, #19550, .F. ) ;
#2072=VERTEX_POINT ( 'NONE', #25493 ) ;
#2076=CARTESIAN_POINT ( 'NONE',  ( 5.953805871968278929, 30.22298757065274444, 13.00000000000000178 ) ) ;
#2082=CARTESIAN_POINT ( 'NONE',  ( 8.806975420853749625, 31.15003855377755571, 12.00000000000000000 ) ) ;
#2107=ORIENTED_EDGE ( 'NONE', *, *, #6049, .T. ) ;
#2121=VERTEX_POINT ( 'NONE', #38498 ) ;
#2125=DIRECTION ( 'NONE',  ( 1.000000000000000000, 0.000000000000000000, 0.000000000000000000 ) ) ;
#2128=DIRECTION ( 'NONE',  ( 1.000000000000000000, 0.000000000000000000, 0.000000000000000000 ) ) ;
#2137=EDGE_CURVE ( 'NONE', #24274, #12134, #28093, .T. ) ;
#2144=AXIS2_PLACEMENT_3D ( 'NONE', #27850, #9570, #15863 ) ;
#2145=DIRECTION ( 'NONE',  ( 0.000000000000000000, 0.000000000000000000, 1.000000000000000000 ) ) ;
#2151=DIRECTION ( 'NONE',  ( 1.000000000000000000, 0.000000000000000000, 0.000000000000000000 ) ) ;
#2175=MECHANICAL_DESIGN_GEOMETRIC_PRESENTATION_REPRESENTATION('',(#39801),#30067);
#2178=AXIS2_PLACEMENT_3D ( 'NONE', #34148, #25386, #25790 ) ;
#2190=DIRECTION ( 'NONE',  ( 0.000000000000000000, 0.000000000000000000, 1.000000000000000000 ) ) ;
#2191=ORIENTED_EDGE ( 'NONE', *, *, #28729, .T. ) ;
#2193=DIRECTION ( 'NONE',  ( -0.000000000000000000, -0.000000000000000000, -1.000000000000000000 ) ) ;
#2194=AXIS2_PLACEMENT_3D ( 'NONE', #5367, #11469, #14716 ) ;
#2196=EDGE_CURVE ( 'NONE', #33602, #21186, #32001, .T. ) ;
#2198=DIRECTION ( 'NONE',  ( 1.000000000000000000, 0.000000000000000000, 0.000000000000000000 ) ) ;
#2203=EDGE_CURVE ( 'NONE', #3338, #23748, #25511, .T. ) ;
#2214=ORIENTED_EDGE ( 'NONE', *, *, #1589, .T. ) ;
#2216=CARTESIAN_POINT ( 'NONE',  ( 0.3762615568374529929, 19.56555719779890978, 12.00000000000000000 ) ) ;
#2219=EDGE_CURVE ( 'NONE', #3881, #28480, #37836, .T. ) ;
#2220=EDGE_LOOP ( 'NONE', ( #38643, #904, #30878, #30669 ) ) ;
#2224=ORIENTED_EDGE ( 'NONE', *, *, #668, .F. ) ;
#2225=CARTESIAN_POINT ( 'NONE',  ( 11.03640989728592281, 29.14264673470096767, 13.00000000000000178 ) ) ;
#2242=EDGE_CURVE ( 'NONE', #634, #15741, #10881, .T. ) ;
#2244=CARTESIAN_POINT ( 'NONE',  ( -0.2474735156158440752, 16.63111439559750693, 13.00000000000000178 ) ) ;
#2271=EDGE_CURVE ( 'NONE', #14129, #36946, #30720, .T. ) ;
#2287=CYLINDRICAL_SURFACE ( 'NONE', #25446, 1.000000000000000000 ) ;
#2289=ORIENTED_EDGE ( 'NONE', *, *, #33735, .T. ) ;
#2313=LINE ( 'NONE', #29934, #33589 ) ;
#2322=VECTOR ( 'NONE', #1694, 1000.000000000000000 ) ;
#2325=CIRCLE ( 'NONE', #27599, 1.000000000000000000 ) ;
#2329=DIRECTION ( 'NONE',  ( 1.000000000000000000, 0.000000000000000000, 0.000000000000000000 ) ) ;
#2331=CARTESIAN_POINT ( 'NONE',  ( 6.440829913680675034, 10.60893893836775348, 12.00000000000000000 ) ) ;
#2339=DIRECTION ( 'NONE',  ( 0.000000000000000000, 0.000000000000000000, 1.000000000000000000 ) ) ;
#2345=EDGE_CURVE ( 'NONE', #7792, #11093, #26828, .T. ) ;
#2347=DIRECTION ( 'NONE',  ( 0.000000000000000000, 0.000000000000000000, 1.000000000000000000 ) ) ;
#2364=VECTOR ( 'NONE', #30625, 1000.000000000000000 ) ;
#2365=DIRECTION ( 'NONE',  ( 0.000000000000000000, 0.000000000000000000, 1.000000000000000000 ) ) ;
#2366=DIRECTION ( 'NONE',  ( 1.000000000000000000, 0.000000000000000000, 0.000000000000000000 ) ) ;
#2367=CARTESIAN_POINT ( 'NONE',  ( -11.39464589777670867, 26.66807349098043289, 13.00000000000000178 ) ) ;
#2378=LINE ( 'NONE', #36106, #16885 ) ;
#2384=DIRECTION ( 'NONE',  ( 1.000000000000000000, 0.000000000000000000, 0.000000000000000000 ) ) ;
#2390=VERTEX_POINT ( 'NONE', #12272 ) ;
#2392=DIRECTION ( 'NONE',  ( 1.000000000000000000, 0.000000000000000000, 0.000000000000000000 ) ) ;
#2395=EDGE_CURVE ( 'NONE', #16360, #21859, #32017, .T. ) ;
#2398=VERTEX_POINT ( 'NONE', #40095 ) ;
#2407=ORIENTED_EDGE ( 'NONE', *, *, #25596, .F. ) ;
#2408=AXIS2_PLACEMENT_3D ( 'NONE', #8042, #29380, #32027 ) ;
#2411=VERTEX_POINT ( 'NONE', #36857 ) ;
#2418=EDGE_CURVE ( 'NONE', #38453, #6898, #12465, .T. ) ;
#2419=VERTEX_POINT ( 'NONE', #22008 ) ;
#2421=FACE_OUTER_BOUND ( 'NONE', #4819, .T. ) ;
#2422=EDGE_LOOP ( 'NONE', ( #33879, #4411 ) ) ;
#2425=EDGE_CURVE ( 'NONE', #21186, #24692, #4710, .T. ) ;
#2429=CARTESIAN_POINT ( 'NONE',  ( 2.835130509701798918, 15.55077355964573904, 12.00000000000000000 ) ) ;
#2436=VERTEX_POINT ( 'NONE', #34013 ) ;
#2442=EDGE_CURVE ( 'NONE', #7574, #1553, #9426, .T. ) ;
#2443=AXIS2_PLACEMENT_3D ( 'NONE', #1981, #39536, #36496 ) ;
#2447=CIRCLE ( 'NONE', #3107, 1.000000000000000000 ) ;
#2462=AXIS2_PLACEMENT_3D ( 'NONE', #20972, #17935, #36411 ) ;
#2478=DIRECTION ( 'NONE',  ( 1.000000000000000000, 0.000000000000000000, 0.000000000000000000 ) ) ;
#2483=CARTESIAN_POINT ( 'NONE',  ( -1.247473515615844075, 16.63111439559750693, 12.00000000000000000 ) ) ;
#2494=VECTOR ( 'NONE', #31133, 1000.000000000000000 ) ;
#2498=ORIENTED_EDGE ( 'NONE', *, *, #169, .F. ) ;
#2500=VERTEX_POINT ( 'NONE', #25057 ) ;
#2501=CIRCLE ( 'NONE', #5737, 16.99999999999999645 ) ;
#2515=VERTEX_POINT ( 'NONE', #15316 ) ;
#2520=ORIENTED_EDGE ( 'NONE', *, *, #18562, .T. ) ;
#2524=AXIS2_PLACEMENT_3D ( 'NONE', #26370, #19881, #32270 ) ;
#2529=FACE_BOUND ( 'NONE', #10441, .T. ) ;
#2531=ORIENTED_EDGE ( 'NONE', *, *, #35614, .T. ) ;
#2552=AXIS2_PLACEMENT_3D ( 'NONE', #23619, #25500, #20173 ) ;
#2566=ORIENTED_EDGE ( 'NONE', *, *, #29697, .T. ) ;
#2577=CIRCLE ( 'NONE', #20095, 1.000000000000000000 ) ;
#2583=CARTESIAN_POINT ( 'NONE',  ( -12.03641663870442713, 15.85735326529964873, 6.000000000000000000 ) ) ;
#2584=AXIS2_PLACEMENT_3D ( 'NONE', #13351, #31841, #28794 ) ;
#2589=DIRECTION ( 'NONE',  ( 1.000000000000000000, 0.000000000000000000, 0.000000000000000000 ) ) ;
#2590=VERTEX_POINT ( 'NONE', #1081 ) ;
#2611=CARTESIAN_POINT ( 'NONE',  ( 16.00000000000000000, 22.50000000000000355, 11.00000000000000178 ) ) ;
#2616=EDGE_CURVE ( 'NONE', #27843, #32176, #35849, .T. ) ;
#2617=CARTESIAN_POINT ( 'NONE',  ( 3.835130509701798918, 15.55077355964573904, 13.00000000000000178 ) ) ;
#2622=AXIS2_PLACEMENT_3D ( 'NONE', #36150, #26599, #21108 ) ;
#2623=CARTESIAN_POINT ( 'NONE',  ( -3.229437847141423124, 24.50739181907689712, 6.000000000000000000 ) ) ;
#2625=DIRECTION ( 'NONE',  ( 1.000000000000000000, 0.000000000000000000, 0.000000000000000000 ) ) ;
#2634=DIRECTION ( 'NONE',  ( 0.000000000000000000, 0.000000000000000000, 1.000000000000000000 ) ) ;
#2636=CARTESIAN_POINT ( 'NONE',  ( 0.9999966292907466192, 22.50000000000031264, 12.00000000000000000 ) ) ;
#2637=CIRCLE ( 'NONE', #14959, 1.000000000000000888 ) ;
#2646=ORIENTED_EDGE ( 'NONE', *, *, #22480, .F. ) ;
#2648=CARTESIAN_POINT ( 'NONE',  ( -4.476907992048016816, 18.63850621467409496, 13.00000000000000178 ) ) ;
#2649=LINE ( 'NONE', #27428, #36051 ) ;
#2650=AXIS2_PLACEMENT_3D ( 'NONE', #7659, #38135, #7855 ) ;
#2651=LINE ( 'NONE', #9145, #3989 ) ;
#2655=DIRECTION ( 'NONE',  ( 0.000000000000000000, 0.000000000000000000, 1.000000000000000000 ) ) ;
#2667=EDGE_CURVE ( 'NONE', #12151, #36438, #3713, .T. ) ;
#2669=EDGE_CURVE ( 'NONE', #5543, #37261, #7269, .T. ) ;
#2671=DIRECTION ( 'NONE',  ( 0.000000000000000000, 0.000000000000000000, 1.000000000000000000 ) ) ;
#2673=CARTESIAN_POINT ( 'NONE',  ( 2.587660364795204782, 9.681887955242936883, 6.000000000000000000 ) ) ;
#2676=AXIS2_PLACEMENT_3D ( 'NONE', #12215, #24607, #37199 ) ;
#2681=DIRECTION ( 'NONE',  ( 0.000000000000000000, 0.000000000000000000, 1.000000000000000000 ) ) ;
#2690=DIRECTION ( 'NONE',  ( 1.000000000000000000, 0.000000000000000000, 0.000000000000000000 ) ) ;
#2691=ORIENTED_EDGE ( 'NONE', *, *, #5546, .F. ) ;
#2702=ORIENTED_EDGE ( 'NONE', *, *, #39692, .F. ) ;
#2706=ORIENTED_EDGE ( 'NONE', *, *, #17533, .T. ) ;
#2713=ORIENTED_EDGE ( 'NONE', *, *, #6496, .T. ) ;
#2716=DIRECTION ( 'NONE',  ( 1.000000000000000000, 0.000000000000000000, 0.000000000000000000 ) ) ;
#2717=EDGE_CURVE ( 'NONE', #18344, #2814, #20286, .T. ) ;
#2722=FACE_BOUND ( 'NONE', #10922, .T. ) ;
#2724=ORIENTED_EDGE ( 'NONE', *, *, #8963, .T. ) ;
#2729=CARTESIAN_POINT ( 'NONE',  ( 8.293999462566144842, 11.53598992149257008, 13.00000000000000178 ) ) ;
#2739=FACE_OUTER_BOUND ( 'NONE', #19124, .T. ) ;
#2740=ORIENTED_EDGE ( 'NONE', *, *, #36853, .F. ) ;
#2749=VERTEX_POINT ( 'NONE', #22600 ) ;
#2752=CIRCLE ( 'NONE', #18953, 1.000000000000000888 ) ;
#2753=DIRECTION ( 'NONE',  ( 1.000000000000000000, 0.000000000000000000, 0.000000000000000000 ) ) ;
#2758=AXIS2_PLACEMENT_3D ( 'NONE', #19676, #24085, #17608 ) ;
#2762=DIRECTION ( 'NONE',  ( 0.000000000000000000, 0.000000000000000000, 1.000000000000000000 ) ) ;
#2764=ORIENTED_EDGE ( 'NONE', *, *, #14758, .F. ) ;
#2766=LINE ( 'NONE', #36500, #39833 ) ;
#2769=DIRECTION ( 'NONE',  ( 0.000000000000000000, 0.000000000000000000, 1.000000000000000000 ) ) ;
#2787=CARTESIAN_POINT ( 'NONE',  ( -12.77091082532341382, 29.60251629318183575, 12.00000000000000000 ) ) ;
#2791=DIRECTION ( 'NONE',  ( 0.000000000000000000, 0.000000000000000000, 1.000000000000000000 ) ) ;
#2792=CARTESIAN_POINT ( 'NONE',  ( -6.440836655099179353, 34.39106106163288246, 6.000000000000000000 ) ) ;
#2806=CIRCLE ( 'NONE', #15759, 1.000000000000000888 ) ;
#2811=ADVANCED_FACE ( 'NONE', ( #8382 ), #2287, .F. ) ;
#2814=VERTEX_POINT ( 'NONE', #23216 ) ;
#2815=CARTESIAN_POINT ( 'NONE',  ( 11.14716901145161643, 12.46304090461738667, 12.00000000000000000 ) ) ;
#2818=AXIS2_PLACEMENT_3D ( 'NONE', #2729, #5776, #24659 ) ;
#2821=EDGE_CURVE ( 'NONE', #25235, #1258, #39735, .T. ) ;
#2823=DIRECTION ( 'NONE',  ( 0.000000000000000000, 0.000000000000000000, 1.000000000000000000 ) ) ;
#2836=DIRECTION ( 'NONE',  ( 0.000000000000000000, 0.000000000000000000, 1.000000000000000000 ) ) ;
#2839=AXIS2_PLACEMENT_3D ( 'NONE', #10969, #20310, #38790 ) ;
#2846=ORIENTED_EDGE ( 'NONE', *, *, #35816, .T. ) ;
#2849=DIRECTION ( 'NONE',  ( 0.000000000000000000, 0.000000000000000000, 1.000000000000000000 ) ) ;
#2863=ORIENTED_EDGE ( 'NONE', *, *, #8963, .F. ) ;
#2870=DIRECTION ( 'NONE',  ( 0.000000000000000000, 0.000000000000000000, 1.000000000000000000 ) ) ;
#2883=ORIENTED_EDGE ( 'NONE', *, *, #22924, .T. ) ;
#2893=EDGE_CURVE ( 'NONE', #22834, #5201, #5972, .T. ) ;
#2912=EDGE_CURVE ( 'NONE', #32554, #20514, #8595, .T. ) ;
#2914=CARTESIAN_POINT ( 'NONE',  ( -5.724378136954611840, 12.76962061027129458, 12.00000000000000000 ) ) ;
#2915=FACE_OUTER_BOUND ( 'NONE', #9754, .T. ) ;
#2918=AXIS2_PLACEMENT_3D ( 'NONE', #40147, #30817, #12322 ) ;
#2921=FACE_BOUND ( 'NONE', #19584, .T. ) ;
#2925=DIRECTION ( 'NONE',  ( 0.000000000000000000, 0.000000000000000000, 1.000000000000000000 ) ) ;
#2933=DIRECTION ( 'NONE',  ( 0.000000000000000000, 0.000000000000000000, 1.000000000000000000 ) ) ;
#2945=VECTOR ( 'NONE', #32735, 1000.000000000000000 ) ;
#2950=VERTEX_POINT ( 'NONE', #24014 ) ;
#2959=AXIS2_PLACEMENT_3D ( 'NONE', #10460, #1731, #32201 ) ;
#2960=AXIS2_PLACEMENT_3D ( 'NONE', #9346, #21726, #34132 ) ;
#2965=EDGE_CURVE ( 'NONE', #21746, #3779, #21550, .T. ) ;
#2975=DIRECTION ( 'NONE',  ( 0.000000000000000000, 0.000000000000000000, 1.000000000000000000 ) ) ;
#2976=AXIS2_PLACEMENT_3D ( 'NONE', #883, #25654, #10221 ) ;
#2977=LINE ( 'NONE', #12318, #18656 ) ;
#2983=ORIENTED_EDGE ( 'NONE', *, *, #7165, .F. ) ;
#2987=LINE ( 'NONE', #21665, #4283 ) ;
#2988=VECTOR ( 'NONE', #5876, 1000.000000000000000 ) ;
#3001=CARTESIAN_POINT ( 'NONE',  ( -18.00000000000000000, 22.50000000000000355, 13.00000000000000178 ) ) ;
#3003=ORIENTED_EDGE ( 'NONE', *, *, #7870, .T. ) ;
#3006=ORIENTED_EDGE ( 'NONE', *, *, #32881, .T. ) ;
#3013=AXIS2_PLACEMENT_3D ( 'NONE', #19573, #3337, #15932 ) ;
#3040=EDGE_CURVE ( 'NONE', #33978, #6629, #20971, .T. ) ;
#3042=ORIENTED_EDGE ( 'NONE', *, *, #18589, .T. ) ;
#3044=DIRECTION ( 'NONE',  ( 1.000000000000000000, 0.000000000000000000, 0.000000000000000000 ) ) ;
#3052=EDGE_CURVE ( 'NONE', #17743, #37305, #11845, .T. ) ;
#3056=ORIENTED_EDGE ( 'NONE', *, *, #6591, .T. ) ;
#3065=CARTESIAN_POINT ( 'NONE',  ( 2.476901250629512941, 26.36149378532653031, 13.00000000000000178 ) ) ;
#3067=LINE ( 'NONE', #6306, #19643 ) ;
#3091=FACE_BOUND ( 'NONE', #37232, .T. ) ;
#3093=VECTOR ( 'NONE', #2365, 1000.000000000000000 ) ;
#3098=ORIENTED_EDGE ( 'NONE', *, *, #3139, .F. ) ;
#3102=AXIS2_PLACEMENT_3D ( 'NONE', #15352, #6002, #15953 ) ;
#3103=EDGE_LOOP ( 'NONE', ( #12291, #25656, #14279, #8995 ) ) ;
#3107=AXIS2_PLACEMENT_3D ( 'NONE', #35785, #1453, #25282 ) ;
#3110=ORIENTED_EDGE ( 'NONE', *, *, #19798, .F. ) ;
#3119=FACE_BOUND ( 'NONE', #12939, .T. ) ;
#3123=CARTESIAN_POINT ( 'NONE',  ( -0.8712085880691411433, 13.69667159339610762, 6.000000000000000000 ) ) ;
#3131=CARTESIAN_POINT ( 'NONE',  ( -7.577547685840081648, 11.84256962714647798, 6.000000000000000000 ) ) ;
#3134=CARTESIAN_POINT ( 'NONE',  ( 1.853166178176219203, 23.42705098312512746, 12.00000000000000000 ) ) ;
#3139=EDGE_CURVE ( 'NONE', #19314, #19744, #37007, .T. ) ;
#3152=CARTESIAN_POINT ( 'NONE',  ( -5.082607396026893376, 23.58034083595207875, 12.00000000000000000 ) ) ;
#3167=DIRECTION ( 'NONE',  ( 1.000000000000000000, 0.000000000000000000, 0.000000000000000000 ) ) ;
#3173=CARTESIAN_POINT ( 'NONE',  ( -1.853172919594719970, 21.57294901687549427, 6.000000000000000000 ) ) ;
#3180=LINE ( 'NONE', #31015, #19762 ) ;
#3182=ORIENTED_EDGE ( 'NONE', *, *, #14027, .F. ) ;
#3185=CARTESIAN_POINT ( 'NONE',  ( -7.294006203984644721, 33.46401007850805343, 6.000000000000000000 ) ) ;
#3188=CARTESIAN_POINT ( 'NONE',  ( -6.953812613386785912, 14.77701242934787906, 13.00000000000000178 ) ) ;
#3220=DIRECTION ( 'NONE',  ( 0.000000000000000000, 0.000000000000000000, 1.000000000000000000 ) ) ;
#3225=ADVANCED_BREP_SHAPE_REPRESENTATION ( '', ( #34952, #24238 ), #27483 ) ;
#3245=EDGE_LOOP ( 'NONE', ( #18238, #565, #19994, #26314 ) ) ;
#3246=CIRCLE ( 'NONE', #34393, 1.000000000000000888 ) ;
#3255=EDGE_LOOP ( 'NONE', ( #22229, #30777, #5734, #23474 ) ) ;
#3257=DIRECTION ( 'NONE',  ( 1.000000000000000000, 0.000000000000000000, 0.000000000000000000 ) ) ;
#3268=EDGE_CURVE ( 'NONE', #14685, #23635, #12540, .T. ) ;
#3269=DIRECTION ( 'NONE',  ( 1.000000000000000000, 0.000000000000000000, 0.000000000000000000 ) ) ;
#3272=DIRECTION ( 'NONE',  ( 0.000000000000000000, 0.000000000000000000, 1.000000000000000000 ) ) ;
#3276=DIRECTION ( 'NONE',  ( 0.000000000000000000, 0.000000000000000000, 1.000000000000000000 ) ) ;
#3278=ORIENTED_EDGE ( 'NONE', *, *, #32069, .T. ) ;
#3283=AXIS2_PLACEMENT_3D ( 'NONE', #15758, #28149, #25101 ) ;
#3284=CARTESIAN_POINT ( 'NONE',  ( -3.853172919594720192, 21.57294901687549427, 13.00000000000000178 ) ) ;
#3285=ORIENTED_EDGE ( 'NONE', *, *, #8355, .T. ) ;
#3286=ORIENTED_EDGE ( 'NONE', *, *, #35387, .F. ) ;
#3289=FACE_BOUND ( 'NONE', #32379, .T. ) ;
#3296=CARTESIAN_POINT ( 'NONE',  ( 6.330070799514983193, 27.28854476845134513, 6.000000000000000000 ) ) ;
#3297=CARTESIAN_POINT ( 'NONE',  ( -0.6237384431625470071, 19.56555719779890978, 13.00000000000000178 ) ) ;
#3299=VECTOR ( 'NONE', #34752, 1000.000000000000000 ) ;
#3302=EDGE_LOOP ( 'NONE', ( #37285, #21030, #2107, #38367 ) ) ;
#3306=ORIENTED_EDGE ( 'NONE', *, *, #37334, .T. ) ;
#3319=CYLINDRICAL_SURFACE ( 'NONE', #23539, 1.000000000000000000 ) ;
#3320=EDGE_CURVE ( 'NONE', #16453, #32987, #8581, .T. ) ;
#3326=ORIENTED_EDGE ( 'NONE', *, *, #2667, .F. ) ;
#3337=DIRECTION ( 'NONE',  ( 0.000000000000000000, 0.000000000000000000, 1.000000000000000000 ) ) ;
#3338=VERTEX_POINT ( 'NONE', #39488 ) ;
#3343=ORIENTED_EDGE ( 'NONE', *, *, #21458, .T. ) ;
#3355=AXIS2_PLACEMENT_3D ( 'NONE', #20751, #26629, #32334 ) ;
#3363=CARTESIAN_POINT ( 'NONE',  ( -1.871208588069141143, 13.69667159339610762, 12.00000000000000000 ) ) ;
#3365=CARTESIAN_POINT ( 'NONE',  ( -7.330077540933487512, 17.71145523154927659, 12.00000000000000000 ) ) ;
#3366=DIRECTION ( 'NONE',  ( 0.000000000000000000, 0.000000000000000000, 1.000000000000000000 ) ) ;
#3369=EDGE_CURVE ( 'NONE', #35589, #19392, #32362, .T. ) ;
#3370=LINE ( 'NONE', #28153, #21600 ) ;
#3376=CARTESIAN_POINT ( 'NONE',  ( -0.7344975573282397363, 36.24516302788250499, 12.00000000000000000 ) ) ;
#3383=ORIENTED_EDGE ( 'NONE', *, *, #17215, .T. ) ;
#3384=CARTESIAN_POINT ( 'NONE',  ( 3.724371395536106188, 32.23037938972932892, 12.00000000000000000 ) ) ;
#3393=ORIENTED_EDGE ( 'NONE', *, *, #31603, .T. ) ;
#3397=VECTOR ( 'NONE', #19157, 1000.000000000000000 ) ;
#3400=CARTESIAN_POINT ( 'NONE',  ( 9.559505275947156377, 25.28115294937476065, 12.00000000000000000 ) ) ;
#3419=DIRECTION ( 'NONE',  ( 1.000000000000000000, 0.000000000000000000, 0.000000000000000000 ) ) ;
#3439=ORIENTED_EDGE ( 'NONE', *, *, #18782, .F. ) ;
#3443=DIRECTION ( 'NONE',  ( 1.000000000000000000, 0.000000000000000000, 0.000000000000000000 ) ) ;
#3445=AXIS2_PLACEMENT_3D ( 'NONE', #16456, #420, #37988 ) ;
#3446=DIRECTION ( 'NONE',  ( 0.000000000000000000, 0.000000000000000000, 1.000000000000000000 ) ) ;
#3453=DIRECTION ( 'NONE',  ( 1.000000000000000000, 0.000000000000000000, 0.000000000000000000 ) ) ;
#3455=VERTEX_POINT ( 'NONE', #25431 ) ;
#3458=EDGE_LOOP ( 'NONE', ( #36985, #9159, #21688, #29766 ) ) ;
#3466=ORIENTED_EDGE ( 'NONE', *, *, #25058, .F. ) ;
#3470=CARTESIAN_POINT ( 'NONE',  ( 1.853166178176219203, 23.42705098312512746, 6.000000000000000000 ) ) ;
#3474=AXIS2_PLACEMENT_3D ( 'NONE', #37342, #34893, #9717 ) ;
#3480=AXIS2_PLACEMENT_3D ( 'NONE', #37247, #6163, #18566 ) ;
#3488=FACE_BOUND ( 'NONE', #33804, .T. ) ;
#3489=CIRCLE ( 'NONE', #12567, 1.000000000000000000 ) ;
#3493=DIRECTION ( 'NONE',  ( 0.000000000000000000, 0.000000000000000000, 1.000000000000000000 ) ) ;
#3497=DIRECTION ( 'NONE',  ( 1.000000000000000000, 0.000000000000000000, 0.000000000000000000 ) ) ;
#3498=ADVANCED_FACE ( 'NONE', ( #28088 ), #12850, .F. ) ;
#3503=CIRCLE ( 'NONE', #4813, 1.000000000000000888 ) ;
#3506=EDGE_LOOP ( 'NONE', ( #34875, #4502, #3644, #36933 ) ) ;
#3515=FACE_BOUND ( 'NONE', #19319, .T. ) ;
#3522=ORIENTED_EDGE ( 'NONE', *, *, #9208, .F. ) ;
#3523=AXIS2_PLACEMENT_3D ( 'NONE', #30511, #31105, #18515 ) ;
#3526=CARTESIAN_POINT ( 'NONE',  ( 7.577540944421576441, 33.15743037285414374, 6.000000000000000000 ) ) ;
#3528=ORIENTED_EDGE ( 'NONE', *, *, #32151, .T. ) ;
#3529=CYLINDRICAL_SURFACE ( 'NONE', #15126, 1.000000000000000000 ) ;
#3534=LINE ( 'NONE', #12876, #36110 ) ;
#3544=DIRECTION ( 'NONE',  ( 0.000000000000000000, 0.000000000000000000, 1.000000000000000000 ) ) ;
#3545=CARTESIAN_POINT ( 'NONE',  ( 5.706335727061685681, 24.35410196624994583, 6.000000000000000000 ) ) ;
#3558=ORIENTED_EDGE ( 'NONE', *, *, #17104, .T. ) ;
#3563=CARTESIAN_POINT ( 'NONE',  ( -6.577547685840081648, 11.84256962714647798, 13.00000000000000178 ) ) ;
#3567=DIRECTION ( 'NONE',  ( 0.000000000000000000, 0.000000000000000000, 1.000000000000000000 ) ) ;
#3568=DIRECTION ( 'NONE',  ( 1.000000000000000000, 0.000000000000000000, 0.000000000000000000 ) ) ;
#3569=FACE_OUTER_BOUND ( 'NONE', #12983, .T. ) ;
#3571=CIRCLE ( 'NONE', #23681, 1.000000000000000000 ) ;
#3574=ORIENTED_EDGE ( 'NONE', *, *, #36374, .F. ) ;
#3582=ORIENTED_EDGE ( 'NONE', *, *, #16560, .F. ) ;
#3588=CIRCLE ( 'NONE', #30223, 1.000000000000000000 ) ;
#3592=ORIENTED_EDGE ( 'NONE', *, *, #38567, .F. ) ;
#3596=ORIENTED_EDGE ( 'NONE', *, *, #6124, .F. ) ;
#3606=VERTEX_POINT ( 'NONE', #28486 ) ;
#3608=DIRECTION ( 'NONE',  ( 1.000000000000000000, 0.000000000000000000, 0.000000000000000000 ) ) ;
#3610=CARTESIAN_POINT ( 'NONE',  ( 12.14716901145161643, 12.46304090461738667, 12.00000000000000000 ) ) ;
#3619=CARTESIAN_POINT ( 'NONE',  ( 9.541469607472739867, 17.40487552589537401, 13.00000000000000178 ) ) ;
#3636=DIRECTION ( 'NONE',  ( 1.000000000000000000, 0.000000000000000000, 0.000000000000000000 ) ) ;
#3637=ORIENTED_EDGE ( 'NONE', *, *, #8355, .F. ) ;
#3639=AXIS2_PLACEMENT_3D ( 'NONE', #25018, #13422, #37808 ) ;
#3644=ORIENTED_EDGE ( 'NONE', *, *, #7479, .T. ) ;
#3650=EDGE_LOOP ( 'NONE', ( #30966, #12947, #37821, #18333 ) ) ;
#3668=LINE ( 'NONE', #21750, #3299 ) ;
#3669=ADVANCED_FACE ( 'NONE', ( #28891 ), #14255, .F. ) ;
#3673=VERTEX_POINT ( 'NONE', #38440 ) ;
#3680=CARTESIAN_POINT ( 'NONE',  ( 6.688300058587269170, 16.47782454277055564, 6.000000000000000000 ) ) ;
#3684=CARTESIAN_POINT ( 'NONE',  ( -3.100643064501314328, 15.70406341247269211, 12.00000000000000000 ) ) ;
#3686=FACE_BOUND ( 'NONE', #15604, .T. ) ;
#3690=ORIENTED_EDGE ( 'NONE', *, *, #16352, .F. ) ;
#3694=DIRECTION ( 'NONE',  ( 0.000000000000000000, 0.000000000000000000, 1.000000000000000000 ) ) ;
#3703=ORIENTED_EDGE ( 'NONE', *, *, #1825, .T. ) ;
#3709=CARTESIAN_POINT ( 'NONE',  ( 0.000000000000000000, 22.50000000000000355, 12.00000000000000000 ) ) ;
#3713=LINE ( 'NONE', #673, #3397 ) ;
#3715=CIRCLE ( 'NONE', #40028, 1.000000000000000000 ) ;
#3720=CARTESIAN_POINT ( 'NONE',  ( -14.64211604268330902, 20.79918788657763429, 6.000000000000000000 ) ) ;
#3723=CARTESIAN_POINT ( 'NONE',  ( -0.2474735156158440752, 16.63111439559750693, 12.00000000000000000 ) ) ;
#3724=ORIENTED_EDGE ( 'NONE', *, *, #3369, .T. ) ;
#3729=FACE_OUTER_BOUND ( 'NONE', #38613, .T. ) ;
#3730=AXIS2_PLACEMENT_3D ( 'NONE', #3545, #34433, #11005 ) ;
#3734=CARTESIAN_POINT ( 'NONE',  ( -7.935776944912362296, 22.65328985282726393, 12.00000000000000000 ) ) ;
#3736=VERTEX_POINT ( 'NONE', #36002 ) ;
#3739=FACE_OUTER_BOUND ( 'NONE', #16500, .T. ) ;
#3740=CARTESIAN_POINT ( 'NONE',  ( -13.64211604268330724, 20.79918788657763429, 12.00000000000000000 ) ) ;
#3745=ORIENTED_EDGE ( 'NONE', *, *, #30869, .T. ) ;
#3753=CIRCLE ( 'NONE', #1839, 1.000000000000000000 ) ;
#3755=CYLINDRICAL_SURFACE ( 'NONE', #35944, 1.000000000000000888 ) ;
#3758=EDGE_CURVE ( 'NONE', #35978, #17743, #14367, .T. ) ;
#3759=ORIENTED_EDGE ( 'NONE', *, *, #15975, .T. ) ;
#3761=CARTESIAN_POINT ( 'NONE',  ( -5.724378136954611840, 12.76962061027129458, 13.00000000000000178 ) ) ;
#3764=DIRECTION ( 'NONE',  ( 0.000000000000000000, 0.000000000000000000, 1.000000000000000000 ) ) ;
#3765=CARTESIAN_POINT ( 'NONE',  ( 9.806975420853749625, 31.15003855377755571, 12.00000000000000000 ) ) ;
#3768=ORIENTED_EDGE ( 'NONE', *, *, #11787, .T. ) ;
#3779=VERTEX_POINT ( 'NONE', #1468 ) ;
#3780=CARTESIAN_POINT ( 'NONE',  ( 7.312035131040564906, 19.41226734497195849, 13.00000000000000178 ) ) ;
#3789=DIRECTION ( 'NONE',  ( -0.000000000000000000, -0.000000000000000000, -1.000000000000000000 ) ) ;
#3800=EDGE_CURVE ( 'NONE', #11948, #35485, #26012, .T. ) ;
#3805=ORIENTED_EDGE ( 'NONE', *, *, #28700, .T. ) ;
#3811=VERTEX_POINT ( 'NONE', #35798 ) ;
#3813=DIRECTION ( 'NONE',  ( 1.000000000000000000, 0.000000000000000000, 0.000000000000000000 ) ) ;
#3816=LINE ( 'NONE', #10930, #2036 ) ;
#3818=EDGE_CURVE ( 'NONE', #25818, #342, #29272, .T. ) ;
#3822=ORIENTED_EDGE ( 'NONE', *, *, #10861, .F. ) ;
#3831=DIRECTION ( 'NONE',  ( 1.000000000000000000, 0.000000000000000000, 0.000000000000000000 ) ) ;
#3841=CIRCLE ( 'NONE', #29781, 1.000000000000000000 ) ;
#3842=CARTESIAN_POINT ( 'NONE',  ( 5.440829913680675034, 10.60893893836775348, 12.00000000000000000 ) ) ;
#3851=ORIENTED_EDGE ( 'NONE', *, *, #18911, .T. ) ;
#3856=VERTEX_POINT ( 'NONE', #17919 ) ;
#3859=CARTESIAN_POINT ( 'NONE',  ( 0.6056960332696259552, 17.55816537872232530, 12.00000000000000000 ) ) ;
#3874=CIRCLE ( 'NONE', #15565, 1.000000000000000888 ) ;
#3875=CARTESIAN_POINT ( 'NONE',  ( -9.917741276437942233, 30.52956727630665057, 13.00000000000000178 ) ) ;
#3881=VERTEX_POINT ( 'NONE', #2076 ) ;
#3885=FACE_BOUND ( 'NONE', #13805, .T. ) ;
#3887=DIRECTION ( 'NONE',  ( 1.000000000000000000, 0.000000000000000000, 0.000000000000000000 ) ) ;
#3897=ADVANCED_FACE ( 'NONE', ( #14861 ), #21152, .F. ) ;
#3907=FACE_OUTER_BOUND ( 'NONE', #11561, .T. ) ;
#3910=FACE_BOUND ( 'NONE', #38784, .T. ) ;
#3942=ORIENTED_EDGE ( 'NONE', *, *, #9008, .T. ) ;
#3958=LINE ( 'NONE', #3173, #22390 ) ;
#3963=CARTESIAN_POINT ( 'NONE',  ( 9.806975420853749625, 31.15003855377755571, 13.00000000000000178 ) ) ;
#3966=DIRECTION ( 'NONE',  ( 1.000000000000000000, 0.000000000000000000, 0.000000000000000000 ) ) ;
#3968=CIRCLE ( 'NONE', #4647, 1.000000000000000000 ) ;
#3989=VECTOR ( 'NONE', #39816, 1000.000000000000000 ) ;
#3991=ORIENTED_EDGE ( 'NONE', *, *, #4938, .T. ) ;
#4003=DIRECTION ( 'NONE',  ( 0.000000000000000000, 0.000000000000000000, 1.000000000000000000 ) ) ;
#4005=DIRECTION ( 'NONE',  ( 0.000000000000000000, 0.000000000000000000, 1.000000000000000000 ) ) ;
#4009=DIRECTION ( 'NONE',  ( 0.000000000000000000, 0.000000000000000000, 1.000000000000000000 ) ) ;
#4019=CARTESIAN_POINT ( 'NONE',  ( 3.118671991557230516, 37.17221401100731981, 12.00000000000000000 ) ) ;
#4031=CARTESIAN_POINT ( 'NONE',  ( -6.330077540933487512, 17.71145523154927659, 12.00000000000000000 ) ) ;
#4038=CARTESIAN_POINT ( 'NONE',  ( 9.788939752379329562, 23.27376113029817617, 12.00000000000000000 ) ) ;
#4046=ORIENTED_EDGE ( 'NONE', *, *, #26108, .T. ) ;
#4059=CARTESIAN_POINT ( 'NONE',  ( -1.358232629781535916, 33.31072022568110924, 12.00000000000000000 ) ) ;
#4063=AXIS2_PLACEMENT_3D ( 'NONE', #33026, #24260, #20823 ) ;
#4065=VERTEX_POINT ( 'NONE', #6300 ) ;
#4068=EDGE_CURVE ( 'NONE', #21075, #29599, #23449, .T. ) ;
#4078=CYLINDRICAL_SURFACE ( 'NONE', #35400, 1.000000000000000000 ) ;
#4083=VECTOR ( 'NONE', #14776, 1000.000000000000000 ) ;
#4092=ORIENTED_EDGE ( 'NONE', *, *, #20964, .T. ) ;
#4094=ADVANCED_FACE ( 'NONE', ( #19 ), #9163, .F. ) ;
#4109=CARTESIAN_POINT ( 'NONE',  ( -3.326590493086956091, 6.849639119454676184, 13.00000000000000178 ) ) ;
#4126=ORIENTED_EDGE ( 'NONE', *, *, #23455, .T. ) ;
#4132=VERTEX_POINT ( 'NONE', #12999 ) ;
#4151=EDGE_CURVE ( 'NONE', #33408, #33800, #28245, .T. ) ;
#4153=CIRCLE ( 'NONE', #4063, 1.000000000000000888 ) ;
#4155=CIRCLE ( 'NONE', #11319, 1.000000000000000000 ) ;
#4166=CARTESIAN_POINT ( 'NONE',  ( 3.118671991557230516, 37.17221401100731981, 12.00000000000000000 ) ) ;
#4172=AXIS2_PLACEMENT_3D ( 'NONE', #25748, #13358, #13966 ) ;
#4177=EDGE_LOOP ( 'NONE', ( #17371, #16830, #29515, #18095 ) ) ;
#4182=CARTESIAN_POINT ( 'NONE',  ( -4.348113209407908464, 9.835177808069893501, 6.000000000000000000 ) ) ;
#4185=AXIS2_PLACEMENT_3D ( 'NONE', #829, #13617, #19116 ) ;
#4197=EDGE_CURVE ( 'NONE', #21746, #4655, #32473, .T. ) ;
#4200=ORIENTED_EDGE ( 'NONE', *, *, #8165, .T. ) ;
#4203=DIRECTION ( 'NONE',  ( 1.000000000000000000, 0.000000000000000000, 0.000000000000000000 ) ) ;
#4207=ORIENTED_EDGE ( 'NONE', *, *, #35998, .F. ) ;
#4217=( GEOMETRIC_REPRESENTATION_CONTEXT ( 3 ) GLOBAL_UNCERTAINTY_ASSIGNED_CONTEXT ( ( #35587 ) ) GLOBAL_UNIT_ASSIGNED_CONTEXT ( ( #35664, #19821, #20224 ) ) REPRESENTATION_CONTEXT ( 'NONE', 'WORKASPACE' ) );
#4219=LINE ( 'NONE', #29001, #24282 ) ;
#4220=DIRECTION ( 'NONE',  ( 0.000000000000000000, 0.000000000000000000, 1.000000000000000000 ) ) ;
#4230=CARTESIAN_POINT ( 'NONE',  ( -5.706342468480190000, 20.64589803375067945, 12.00000000000000000 ) ) ;
#4233=DIRECTION ( 'NONE',  ( 0.000000000000000000, 0.000000000000000000, 1.000000000000000000 ) ) ;
#4244=DIRECTION ( 'NONE',  ( 1.000000000000000000, 0.000000000000000000, 0.000000000000000000 ) ) ;
#4254=AXIS2_PLACEMENT_3D ( 'NONE', #38085, #28741, #23458 ) ;
#4263=ORIENTED_EDGE ( 'NONE', *, *, #24570, .F. ) ;
#4265=CARTESIAN_POINT ( 'NONE',  ( 9.541469607472739867, 17.40487552589537401, 12.00000000000000000 ) ) ;
#4266=CYLINDRICAL_SURFACE ( 'NONE', #34444, 1.000000000000000888 ) ;
#4269=ORIENTED_EDGE ( 'NONE', *, *, #29165, .T. ) ;
#4271=CARTESIAN_POINT ( 'NONE',  ( 6.082600654608392610, 21.41965916404854298, 12.00000000000000000 ) ) ;
#4279=CIRCLE ( 'NONE', #26998, 1.000000000000000000 ) ;
#4283=VECTOR ( 'NONE', #18036, 1000.000000000000000 ) ;
#4284=DIRECTION ( 'NONE',  ( 1.000000000000000000, 0.000000000000000000, 0.000000000000000000 ) ) ;
#4292=DIRECTION ( 'NONE',  ( 0.000000000000000000, 0.000000000000000000, 1.000000000000000000 ) ) ;
#4293=EDGE_LOOP ( 'NONE', ( #26428, #20714, #33713, #2407 ) ) ;
#4295=LINE ( 'NONE', #35176, #38851 ) ;
#4296=CARTESIAN_POINT ( 'NONE',  ( -0.9819677022348329842, 30.37627742347970283, 6.000000000000000000 ) ) ;
#4302=CARTESIAN_POINT ( 'NONE',  ( 3.724371395536106188, 32.23037938972932892, 6.000000000000000000 ) ) ;
#4315=FACE_BOUND ( 'NONE', #17062, .T. ) ;
#4320=ADVANCED_FACE ( 'NONE', ( #23357 ), #7906, .F. ) ;
#4328=VERTEX_POINT ( 'NONE', #1828 ) ;
#4330=DIRECTION ( 'NONE',  ( 0.000000000000000000, 0.000000000000000000, 1.000000000000000000 ) ) ;
#4335=CARTESIAN_POINT ( 'NONE',  ( 4.211395437248501850, 12.61633075744433796, 13.00000000000000178 ) ) ;
#4341=CARTESIAN_POINT ( 'NONE',  ( 0.9819609608163288872, 14.62372257652092422, 6.000000000000000000 ) ) ;
#4351=EDGE_LOOP ( 'NONE', ( #33099, #8110 ) ) ;
#4352=EDGE_CURVE ( 'NONE', #32176, #27843, #9842, .T. ) ;
#4354=FACE_OUTER_BOUND ( 'NONE', #13393, .T. ) ;
#4355=CARTESIAN_POINT ( 'NONE',  ( 8.293999462566144842, 11.53598992149257008, 13.00000000000000178 ) ) ;
#4360=DIRECTION ( 'NONE',  ( 1.000000000000000000, 0.000000000000000000, 0.000000000000000000 ) ) ;
#4362=EDGE_LOOP ( 'NONE', ( #29197, #32537 ) ) ;
#4374=CARTESIAN_POINT ( 'NONE',  ( -0.3582326297815359162, 33.31072022568110924, 6.000000000000000000 ) ) ;
#4378=CARTESIAN_POINT ( 'NONE',  ( 13.01837422881150452, 21.26636931122159169, 6.000000000000000000 ) ) ;
#4382=ORIENTED_EDGE ( 'NONE', *, *, #18265, .F. ) ;
#4396=EDGE_LOOP ( 'NONE', ( #24911, #28883, #14746, #4899 ) ) ;
#4401=ORIENTED_EDGE ( 'NONE', *, *, #29148, .F. ) ;
#4402=DIRECTION ( 'NONE',  ( 1.000000000000000000, 0.000000000000000000, 0.000000000000000000 ) ) ;
#4406=DIRECTION ( 'NONE',  ( 1.000000000000000000, 0.000000000000000000, 0.000000000000000000 ) ) ;
#4411=ORIENTED_EDGE ( 'NONE', *, *, #30649, .F. ) ;
#4413=CARTESIAN_POINT ( 'NONE',  ( 0.6237317017440463518, 25.43444280220171194, 6.000000000000000000 ) ) ;
#4419=CARTESIAN_POINT ( 'NONE',  ( 5.100636323082810009, 29.29593658752792962, 12.00000000000000000 ) ) ;
#4420=DIRECTION ( 'NONE',  ( 0.000000000000000000, 0.000000000000000000, 1.000000000000000000 ) ) ;
#4428=CARTESIAN_POINT ( 'NONE',  ( -2.247473515615844075, 16.63111439559750693, 12.00000000000000000 ) ) ;
#4434=CIRCLE ( 'NONE', #14819, 1.000000000000000000 ) ;
#4436=FACE_OUTER_BOUND ( 'NONE', #39055, .T. ) ;
#4437=EDGE_CURVE ( 'NONE', #2950, #7051, #18916, .T. ) ;
#4457=EDGE_CURVE ( 'NONE', #16497, #3811, #18067, .T. ) ;
#4464=DIRECTION ( 'NONE',  ( 0.000000000000000000, 0.000000000000000000, 1.000000000000000000 ) ) ;
#4468=ORIENTED_EDGE ( 'NONE', *, *, #1727, .F. ) ;
#4469=CARTESIAN_POINT ( 'NONE',  ( 0.000000000000000000, 0.000000000000000000, 0.000000000000000000 ) ) ;
#4471=CYLINDRICAL_SURFACE ( 'NONE', #17630, 1.000000000000000888 ) ;
#4472=DIRECTION ( 'NONE',  ( 1.000000000000000000, 0.000000000000000000, 0.000000000000000000 ) ) ;
#4476=CARTESIAN_POINT ( 'NONE',  ( -2.853172919594720192, 21.57294901687549427, 13.00000000000000178 ) ) ;
#4480=CARTESIAN_POINT ( 'NONE',  ( 14.01837422881150452, 21.26636931122159169, 13.00000000000000178 ) ) ;
#4482=CIRCLE ( 'NONE', #37576, 18.00000000000000000 ) ;
#4483=ORIENTED_EDGE ( 'NONE', *, *, #38781, .T. ) ;
#4497=ORIENTED_EDGE ( 'NONE', *, *, #22300, .T. ) ;
#4499=CYLINDRICAL_SURFACE ( 'NONE', #3730, 1.000000000000000000 ) ;
#4501=DIRECTION ( 'NONE',  ( 0.000000000000000000, 0.000000000000000000, 1.000000000000000000 ) ) ;
#4502=ORIENTED_EDGE ( 'NONE', *, *, #11668, .F. ) ;
#4505=ORIENTED_EDGE ( 'NONE', *, *, #6887, .F. ) ;
#4516=AXIS2_PLACEMENT_3D ( 'NONE', #1125, #13506, #10671 ) ;
#4519=EDGE_CURVE ( 'NONE', #17087, #11673, #12416, .T. ) ;
#4531=EDGE_CURVE ( 'NONE', #23343, #14560, #22073, .T. ) ;
#4540=CYLINDRICAL_SURFACE ( 'NONE', #17875, 1.000000000000000888 ) ;
#4549=FACE_OUTER_BOUND ( 'NONE', #16582, .T. ) ;
#4551=AXIS2_PLACEMENT_3D ( 'NONE', #19648, #29201, #38136 ) ;
#4569=ORIENTED_EDGE ( 'NONE', *, *, #39478, .T. ) ;
#4573=AXIS2_PLACEMENT_3D ( 'NONE', #14961, #34448, #12115 ) ;
#4575=CARTESIAN_POINT ( 'NONE',  ( -8.294006203984645609, 33.46401007850805343, 13.00000000000000178 ) ) ;
#4580=FACE_OUTER_BOUND ( 'NONE', #34181, .T. ) ;
#4583=EDGE_CURVE ( 'NONE', #8501, #27275, #27005, .T. ) ;
#4597=ORIENTED_EDGE ( 'NONE', *, *, #32250, .F. ) ;
#4606=ORIENTED_EDGE ( 'NONE', *, *, #7349, .T. ) ;
#4607=DIRECTION ( 'NONE',  ( 0.000000000000000000, 0.000000000000000000, 1.000000000000000000 ) ) ;
#4608=CARTESIAN_POINT ( 'NONE',  ( 0.6237317017440463518, 25.43444280220171194, 12.00000000000000000 ) ) ;
#4611=FACE_OUTER_BOUND ( 'NONE', #29914, .T. ) ;
#4619=DIRECTION ( 'NONE',  ( 0.000000000000000000, 0.000000000000000000, 1.000000000000000000 ) ) ;
#4626=CARTESIAN_POINT ( 'NONE',  ( 14.26584437371809777, 27.13525491562438319, 13.00000000000000178 ) ) ;
#4634=CARTESIAN_POINT ( 'NONE',  ( 0.000000000000000000, 22.50000000000000355, 12.00000000000000000 ) ) ;
#4637=CARTESIAN_POINT ( 'NONE',  ( 4.476901250629513385, 26.36149378532653031, 13.00000000000000178 ) ) ;
#4647=AXIS2_PLACEMENT_3D ( 'NONE', #20118, #29450, #10365 ) ;
#4655=VERTEX_POINT ( 'NONE', #3610 ) ;
#4658=ORIENTED_EDGE ( 'NONE', *, *, #24570, .T. ) ;
#4662=AXIS2_PLACEMENT_3D ( 'NONE', #32076, #3446, #4244 ) ;
#4668=CARTESIAN_POINT ( 'NONE',  ( -8.577547685840080760, 11.84256962714647798, 13.00000000000000178 ) ) ;
#4677=DIRECTION ( 'NONE',  ( 0.000000000000000000, 0.000000000000000000, 1.000000000000000000 ) ) ;
#4690=EDGE_LOOP ( 'NONE', ( #3098, #25683, #14065, #31716 ) ) ;
#4694=FACE_BOUND ( 'NONE', #9684, .T. ) ;
#4707=EDGE_CURVE ( 'NONE', #17253, #39380, #30611, .T. ) ;
#4708=ORIENTED_EDGE ( 'NONE', *, *, #6811, .F. ) ;
#4710=CIRCLE ( 'NONE', #32611, 1.000000000000000000 ) ;
#4722=VECTOR ( 'NONE', #20399, 1000.000000000000000 ) ;
#4736=VERTEX_POINT ( 'NONE', #12557 ) ;
#4741=CARTESIAN_POINT ( 'NONE',  ( -10.16521142134453548, 24.66068167190384841, 12.00000000000000000 ) ) ;
#4745=ORIENTED_EDGE ( 'NONE', *, *, #17376, .F. ) ;
#4752=DIRECTION ( 'NONE',  ( 0.000000000000000000, 0.000000000000000000, 1.000000000000000000 ) ) ;
#4753=AXIS2_PLACEMENT_3D ( 'NONE', #31957, #37853, #1289 ) ;
#4754=DIRECTION ( 'NONE',  ( 1.000000000000000000, 0.000000000000000000, 0.000000000000000000 ) ) ;
#4755=EDGE_LOOP ( 'NONE', ( #6573, #6456 ) ) ;
#4764=CARTESIAN_POINT ( 'NONE',  ( 10.78893975237932956, 23.27376113029817617, 12.00000000000000000 ) ) ;
#4766=AXIS2_PLACEMENT_3D ( 'NONE', #20680, #38550, #14372 ) ;
#4775=DIRECTION ( 'NONE',  ( 1.000000000000000000, 0.000000000000000000, 0.000000000000000000 ) ) ;
#4779=CIRCLE ( 'NONE', #9970, 1.000000000000000888 ) ;
#4788=ORIENTED_EDGE ( 'NONE', *, *, #11668, .T. ) ;
#4798=VERTEX_POINT ( 'NONE', #10107 ) ;
#4802=ADVANCED_FACE ( 'NONE', ( #7451 ), #38744, .F. ) ;
#4810=CARTESIAN_POINT ( 'NONE',  ( 0.9819609608163288872, 14.62372257652092422, 13.00000000000000178 ) ) ;
#4813=AXIS2_PLACEMENT_3D ( 'NONE', #22690, #16609, #20467 ) ;
#4815=ORIENTED_EDGE ( 'NONE', *, *, #39284, .F. ) ;
#4819=EDGE_LOOP ( 'NONE', ( #12199, #8147, #21082, #23738 ) ) ;
#4820=VECTOR ( 'NONE', #22495, 1000.000000000000000 ) ;
#4822=FACE_OUTER_BOUND ( 'NONE', #32447, .T. ) ;
#4823=CARTESIAN_POINT ( 'NONE',  ( 3.587660364795204782, 9.681887955242936883, 13.00000000000000178 ) ) ;
#4829=VERTEX_POINT ( 'NONE', #35499 ) ;
#4834=CARTESIAN_POINT ( 'NONE',  ( -1.623738443162547007, 19.56555719779890978, 13.00000000000000178 ) ) ;
#4848=ORIENTED_EDGE ( 'NONE', *, *, #29746, .T. ) ;
#4856=CYLINDRICAL_SURFACE ( 'NONE', #9602, 1.000000000000000000 ) ;
#4863=CIRCLE ( 'NONE', #9418, 1.000000000000000000 ) ;
#4865=ORIENTED_EDGE ( 'NONE', *, *, #2893, .T. ) ;
#4871=VERTEX_POINT ( 'NONE', #28994 ) ;
#4872=DIRECTION ( 'NONE',  ( 1.000000000000000000, 0.000000000000000000, 0.000000000000000000 ) ) ;
#4879=ADVANCED_FACE ( 'NONE', ( #38338 ), #26142, .F. ) ;
#4880=CIRCLE ( 'NONE', #10713, 16.00000000000000000 ) ;
#4881=ORIENTED_EDGE ( 'NONE', *, *, #4352, .T. ) ;
#4886=EDGE_CURVE ( 'NONE', #17473, #5105, #1367, .T. ) ;
#4889=EDGE_LOOP ( 'NONE', ( #28303, #36699 ) ) ;
#4893=FACE_BOUND ( 'NONE', #36289, .T. ) ;
#4898=CARTESIAN_POINT ( 'NONE',  ( 18.00000000000000000, 22.50000000000000711, 11.00000000000000178 ) ) ;
#4899=ORIENTED_EDGE ( 'NONE', *, *, #18324, .T. ) ;
#4904=ORIENTED_EDGE ( 'NONE', *, *, #19699, .T. ) ;
#4910=ORIENTED_EDGE ( 'NONE', *, *, #3818, .F. ) ;
#4916=EDGE_CURVE ( 'NONE', #21094, #3673, #31186, .T. ) ;
#4918=DIRECTION ( 'NONE',  ( 1.000000000000000000, 0.000000000000000000, 0.000000000000000000 ) ) ;
#4919=EDGE_LOOP ( 'NONE', ( #19898, #39272, #17299, #35275 ) ) ;
#4920=DIRECTION ( 'NONE',  ( 0.000000000000000000, 0.000000000000000000, 1.000000000000000000 ) ) ;
#4927=CIRCLE ( 'NONE', #1042, 1.000000000000000888 ) ;
#4929=CARTESIAN_POINT ( 'NONE',  ( -12.64211604268330724, 20.79918788657763429, 12.00000000000000000 ) ) ;
#4932=EDGE_LOOP ( 'NONE', ( #4910, #36188, #32120, #16272 ) ) ;
#4938=EDGE_CURVE ( 'NONE', #888, #39039, #9781, .T. ) ;
#4943=ORIENTED_EDGE ( 'NONE', *, *, #27945, .T. ) ;
#4947=DIRECTION ( 'NONE',  ( 0.000000000000000000, 0.000000000000000000, 1.000000000000000000 ) ) ;
#4953=ORIENTED_EDGE ( 'NONE', *, *, #11067, .T. ) ;
#4957=VECTOR ( 'NONE', #32535, 1000.000000000000000 ) ;
#4968=DIRECTION ( 'NONE',  ( 1.000000000000000000, 0.000000000000000000, 0.000000000000000000 ) ) ;
#4974=DIRECTION ( 'NONE',  ( 0.000000000000000000, 0.000000000000000000, 1.000000000000000000 ) ) ;
#4977=CARTESIAN_POINT ( 'NONE',  ( 7.064564986133971658, 13.54338174056915456, 12.00000000000000000 ) ) ;
#4980=AXIS2_PLACEMENT_3D ( 'NONE', #33745, #33543, #3044 ) ;
#4982=ORIENTED_EDGE ( 'NONE', *, *, #11891, .T. ) ;
#4988=VERTEX_POINT ( 'NONE', #15513 ) ;
#4992=DIRECTION ( 'NONE',  ( 0.000000000000000000, 0.000000000000000000, 1.000000000000000000 ) ) ;
#5003=VERTEX_POINT ( 'NONE', #27304 ) ;
#5014=DIRECTION ( 'NONE',  ( 0.000000000000000000, 0.000000000000000000, 1.000000000000000000 ) ) ;
#5015=CIRCLE ( 'NONE', #27714, 1.000000000000000000 ) ;
#5019=EDGE_CURVE ( 'NONE', #7705, #26791, #27896, .T. ) ;
#5039=CIRCLE ( 'NONE', #22538, 1.000000000000000888 ) ;
#5046=VERTEX_POINT ( 'NONE', #27693 ) ;
#5050=CIRCLE ( 'NONE', #18021, 16.00000000000000000 ) ;
#5055=VERTEX_POINT ( 'NONE', #24450 ) ;
#5063=CARTESIAN_POINT ( 'NONE',  ( -4.100643064501314328, 15.70406341247269211, 13.00000000000000178 ) ) ;
#5068=CYLINDRICAL_SURFACE ( 'NONE', #19444, 1.000000000000000888 ) ;
#5069=VERTEX_POINT ( 'NONE', #34002 ) ;
#5070=FILL_AREA_STYLE ('',( #39790 ) ) ;
#5079=EDGE_LOOP ( 'NONE', ( #2646, #28638, #28377, #14455 ) ) ;
#5092=ORIENTED_EDGE ( 'NONE', *, *, #9815, .F. ) ;
#5096=AXIS2_PLACEMENT_3D ( 'NONE', #7676, #13160, #38352 ) ;
#5099=ORIENTED_EDGE ( 'NONE', *, *, #31891, .T. ) ;
#5105=VERTEX_POINT ( 'NONE', #39493 ) ;
#5107=DIRECTION ( 'NONE',  ( 1.000000000000000000, 0.000000000000000000, 0.000000000000000000 ) ) ;
#5112=ORIENTED_EDGE ( 'NONE', *, *, #16329, .T. ) ;
#5116=ADVANCED_FACE ( 'NONE', ( #32660 ), #11070, .F. ) ;
#5118=CARTESIAN_POINT ( 'NONE',  ( -3.370709253380788084E-06, 22.50000000000031264, 12.00000000000000000 ) ) ;
#5124=CIRCLE ( 'NONE', #38212, 18.00000000000000000 ) ;
#5129=AXIS2_PLACEMENT_3D ( 'NONE', #32355, #20369, #4918 ) ;
#5130=DIRECTION ( 'NONE',  ( 1.000000000000000000, 0.000000000000000000, 0.000000000000000000 ) ) ;
#5134=EDGE_LOOP ( 'NONE', ( #35801, #2702 ) ) ;
#5139=ORIENTED_EDGE ( 'NONE', *, *, #27671, .T. ) ;
#5141=ORIENTED_EDGE ( 'NONE', *, *, #35796, .F. ) ;
#5143=CARTESIAN_POINT ( 'NONE',  ( -5.458872323573595864, 26.51478363815348160, 6.000000000000000000 ) ) ;
#5153=DIRECTION ( 'NONE',  ( 1.000000000000000000, 0.000000000000000000, 0.000000000000000000 ) ) ;
#5154=CARTESIAN_POINT ( 'NONE',  ( -5.348113209407908464, 9.835177808069893501, 6.000000000000000000 ) ) ;
#5155=ORIENTED_EDGE ( 'NONE', *, *, #14362, .T. ) ;
#5160=EDGE_LOOP ( 'NONE', ( #5092, #21096, #24093, #4982, #16138, #5494, #19649, #5139, #40159, #8031, #4200, #33238, #35762, #16784, #28868, #23622, #29969, #24635, #35062, #27667, #22322, #3745, #9855, #31781, #18261, #292 ) ) ;
#5170=CARTESIAN_POINT ( 'NONE',  ( -4.706342468480190000, 20.64589803375067945, 12.00000000000000000 ) ) ;
#5172=ORIENTED_EDGE ( 'NONE', *, *, #30341, .T. ) ;
#5185=CARTESIAN_POINT ( 'NONE',  ( 0.8712018466506370462, 31.30332840660451765, 6.000000000000000000 ) ) ;
#5187=EDGE_LOOP ( 'NONE', ( #17458, #27885, #1714, #16908 ) ) ;
#5192=DIRECTION ( 'NONE',  ( 0.000000000000000000, 0.000000000000000000, 1.000000000000000000 ) ) ;
#5196=ADVANCED_FACE ( 'NONE', ( #9618 ), #472, .F. ) ;
#5199=FACE_OUTER_BOUND ( 'NONE', #13457, .T. ) ;
#5201=VERTEX_POINT ( 'NONE', #28296 ) ;
#5203=DIRECTION ( 'NONE',  ( 1.000000000000000000, 0.000000000000000000, 0.000000000000000000 ) ) ;
#5204=DIRECTION ( 'NONE',  ( 0.000000000000000000, -1.000000000000000000, 0.000000000000000000 ) ) ;
#5209=CARTESIAN_POINT ( 'NONE',  ( -13.01838097023000707, 23.73363068877903359, 12.00000000000000000 ) ) ;
#5215=ADVANCED_FACE ( 'NONE', ( #3907 ), #15704, .F. ) ;
#5219=CARTESIAN_POINT ( 'NONE',  ( 14.26584437371809777, 27.13525491562438319, 12.00000000000000000 ) ) ;
#5237=CARTESIAN_POINT ( 'NONE',  ( 12.64210930126479937, 24.20081211342298744, 13.00000000000000178 ) ) ;
#5250=ORIENTED_EDGE ( 'NONE', *, *, #21062, .T. ) ;
#5257=EDGE_LOOP ( 'NONE', ( #14272, #17943, #32119, #19918 ) ) ;
#5266=CARTESIAN_POINT ( 'NONE',  ( 9.806975420853749625, 31.15003855377755571, 6.000000000000000000 ) ) ;
#5271=CIRCLE ( 'NONE', #12401, 1.000000000000000888 ) ;
#5275=EDGE_LOOP ( 'NONE', ( #11952, #31131, #17080, #33165 ) ) ;
#5289=ORIENTED_EDGE ( 'NONE', *, *, #12815, .F. ) ;
#5290=VERTEX_POINT ( 'NONE', #9814 ) ;
#5298=ADVANCED_FACE ( 'NONE', ( #34200 ), #16107, .F. ) ;
#5303=ORIENTED_EDGE ( 'NONE', *, *, #36682, .F. ) ;
#5321=CARTESIAN_POINT ( 'NONE',  ( 8.183240348400453001, 28.21559575157615996, 13.00000000000000178 ) ) ;
#5326=CARTESIAN_POINT ( 'NONE',  ( -11.41268156625113406, 18.79179606750104981, 12.00000000000000000 ) ) ;
#5328=EDGE_LOOP ( 'NONE', ( #8807, #2289, #6785, #39254 ) ) ;
#5330=EDGE_LOOP ( 'NONE', ( #14409, #26437 ) ) ;
#5344=ORIENTED_EDGE ( 'NONE', *, *, #34521, .T. ) ;
#5347=AXIS2_PLACEMENT_3D ( 'NONE', #14063, #39450, #5130 ) ;
#5361=DIRECTION ( 'NONE',  ( 1.000000000000000000, 0.000000000000000000, 0.000000000000000000 ) ) ;
#5362=DIRECTION ( 'NONE',  ( 0.000000000000000000, 0.000000000000000000, 1.000000000000000000 ) ) ;
#5367=CARTESIAN_POINT ( 'NONE',  ( -7.935776944912362296, 22.65328985282726393, 13.00000000000000178 ) ) ;
#5372=PLANE ( 'NONE',  #37636 ) ;
#5374=CARTESIAN_POINT ( 'NONE',  ( -6.688306800005769048, 28.52217545723006609, 13.00000000000000178 ) ) ;
#5377=AXIS2_PLACEMENT_3D ( 'NONE', #38600, #32106, #4872 ) ;
#5382=CIRCLE ( 'NONE', #6050, 16.00000000000000000 ) ;
#5389=CYLINDRICAL_SURFACE ( 'NONE', #23133, 1.000000000000000000 ) ;
#5402=CARTESIAN_POINT ( 'NONE',  ( -3.100643064501314328, 15.70406341247269211, 13.00000000000000178 ) ) ;
#5415=ORIENTED_EDGE ( 'NONE', *, *, #16560, .T. ) ;
#5417=CYLINDRICAL_SURFACE ( 'NONE', #15195, 1.000000000000000000 ) ;
#5418=ADVANCED_FACE ( 'NONE', ( #29303 ), #14057, .F. ) ;
#5421=CIRCLE ( 'NONE', #17795, 1.000000000000000000 ) ;
#5422=DIRECTION ( 'NONE',  ( 1.000000000000000000, 0.000000000000000000, 0.000000000000000000 ) ) ;
#5423=CARTESIAN_POINT ( 'NONE',  ( -8.559512017365658920, 19.71884705062586107, 12.00000000000000000 ) ) ;
#5428=CARTESIAN_POINT ( 'NONE',  ( 11.14716901145161643, 12.46304090461738667, 6.000000000000000000 ) ) ;
#5430=DIRECTION ( 'NONE',  ( 0.000000000000000000, 0.000000000000000000, 1.000000000000000000 ) ) ;
#5464=AXIS2_PLACEMENT_3D ( 'NONE', #29508, #1685, #11031 ) ;
#5466=ORIENTED_EDGE ( 'NONE', *, *, #8665, .T. ) ;
#5474=DIRECTION ( 'NONE',  ( 0.000000000000000000, 0.000000000000000000, 1.000000000000000000 ) ) ;
#5477=CARTESIAN_POINT ( 'NONE',  ( -6.688306800005769048, 28.52217545723006609, 13.00000000000000178 ) ) ;
#5482=DIRECTION ( 'NONE',  ( 0.000000000000000000, 0.000000000000000000, 1.000000000000000000 ) ) ;
#5490=EDGE_LOOP ( 'NONE', ( #692, #39856, #14190, #25497 ) ) ;
#5493=CARTESIAN_POINT ( 'NONE',  ( -0.01803903918367114056, 14.62372257652092422, 12.00000000000000000 ) ) ;
#5494=ORIENTED_EDGE ( 'NONE', *, *, #8705, .F. ) ;
#5495=CIRCLE ( 'NONE', #23004, 1.000000000000000888 ) ;
#5498=EDGE_LOOP ( 'NONE', ( #30727, #32701 ) ) ;
#5502=VERTEX_POINT ( 'NONE', #23408 ) ;
#5507=DIRECTION ( 'NONE',  ( 1.000000000000000000, 0.000000000000000000, 0.000000000000000000 ) ) ;
#5509=EDGE_CURVE ( 'NONE', #26584, #21822, #39643, .T. ) ;
#5511=DIRECTION ( 'NONE',  ( 0.000000000000000000, 0.000000000000000000, 1.000000000000000000 ) ) ;
#5514=FACE_OUTER_BOUND ( 'NONE', #31260, .T. ) ;
#5517=EDGE_CURVE ( 'NONE', #839, #22834, #26450, .T. ) ;
#5519=DIRECTION ( 'NONE',  ( 1.000000000000000000, 0.000000000000000000, 0.000000000000000000 ) ) ;
#5525=ORIENTED_EDGE ( 'NONE', *, *, #337, .F. ) ;
#5528=AXIS2_PLACEMENT_3D ( 'NONE', #40011, #33544, #33140 ) ;
#5532=ORIENTED_EDGE ( 'NONE', *, *, #1324, .T. ) ;
#5543=VERTEX_POINT ( 'NONE', #2082 ) ;
#5546=EDGE_CURVE ( 'NONE', #18400, #8408, #39042, .T. ) ;
#5547=CARTESIAN_POINT ( 'NONE',  ( 5.688300058587269170, 16.47782454277055564, 13.00000000000000178 ) ) ;
#5554=EDGE_LOOP ( 'NONE', ( #31328, #31703, #12353, #38632 ) ) ;
#5557=DIRECTION ( 'NONE',  ( 0.000000000000000000, 0.000000000000000000, 1.000000000000000000 ) ) ;
#5558=DIRECTION ( 'NONE',  ( 0.000000000000000000, 0.000000000000000000, 1.000000000000000000 ) ) ;
#5559=CIRCLE ( 'NONE', #8137, 1.000000000000000888 ) ;
#5564=FACE_BOUND ( 'NONE', #35416, .T. ) ;
#5581=ORIENTED_EDGE ( 'NONE', *, *, #7870, .F. ) ;
#5584=FACE_OUTER_BOUND ( 'NONE', #27287, .T. ) ;
#5586=CARTESIAN_POINT ( 'NONE',  ( -10.14717575287011542, 32.53695909538323860, 6.000000000000000000 ) ) ;
#5615=VECTOR ( 'NONE', #40109, 1000.000000000000000 ) ;
#5619=FACE_OUTER_BOUND ( 'NONE', #39417, .T. ) ;
#5623=CARTESIAN_POINT ( 'NONE',  ( 3.835130509701798918, 15.55077355964573904, 12.00000000000000000 ) ) ;
#5627=CARTESIAN_POINT ( 'NONE',  ( 4.706335727061685681, 24.35410196624994583, 13.00000000000000178 ) ) ;
#5640=ADVANCED_FACE ( 'NONE', ( #27651 ), #23806, .F. ) ;
#5644=AXIS2_PLACEMENT_3D ( 'NONE', #19369, #35213, #19168 ) ;
#5654=DIRECTION ( 'NONE',  ( 0.000000000000000000, 0.000000000000000000, 1.000000000000000000 ) ) ;
#5657=CARTESIAN_POINT ( 'NONE',  ( -16.00000000000000000, 22.50000000000000711, 11.00000000000000178 ) ) ;
#5663=CARTESIAN_POINT ( 'NONE',  ( -1.871208588069141143, 13.69667159339610762, 13.00000000000000178 ) ) ;
#5671=ADVANCED_FACE ( 'NONE', ( #33369 ), #27451, .F. ) ;
#5684=VERTEX_POINT ( 'NONE', #39837 ) ;
#5687=ADVANCED_FACE ( 'NONE', ( #24403 ), #15640, .F. ) ;
#5700=EDGE_LOOP ( 'NONE', ( #3466, #9802 ) ) ;
#5703=CIRCLE ( 'NONE', #28404, 1.000000000000000000 ) ;
#5715=DIRECTION ( 'NONE',  ( 0.000000000000000000, 0.000000000000000000, 1.000000000000000000 ) ) ;
#5716=DIRECTION ( 'NONE',  ( 0.000000000000000000, 0.000000000000000000, 1.000000000000000000 ) ) ;
#5722=CARTESIAN_POINT ( 'NONE',  ( 0.000000000000000000, 22.50000000000000355, 12.00000000000000000 ) ) ;
#5723=DIRECTION ( 'NONE',  ( 0.000000000000000000, 0.000000000000000000, 1.000000000000000000 ) ) ;
#5724=ORIENTED_EDGE ( 'NONE', *, *, #22456, .F. ) ;
#5734=ORIENTED_EDGE ( 'NONE', *, *, #34833, .T. ) ;
#5736=VERTEX_POINT ( 'NONE', #8769 ) ;
#5737=AXIS2_PLACEMENT_3D ( 'NONE', #6256, #24349, #36748 ) ;
#5752=ORIENTED_EDGE ( 'NONE', *, *, #10882, .F. ) ;
#5759=ADVANCED_FACE ( 'NONE', ( #15262 ), #33566, .F. ) ;
#5760=DIRECTION ( 'NONE',  ( -0.000000000000000000, -0.000000000000000000, -1.000000000000000000 ) ) ;
#5762=VECTOR ( 'NONE', #32063, 1000.000000000000000 ) ;
#5768=FACE_BOUND ( 'NONE', #19749, .T. ) ;
#5773=EDGE_CURVE ( 'NONE', #39686, #4328, #28648, .T. ) ;
#5776=DIRECTION ( 'NONE',  ( 0.000000000000000000, 0.000000000000000000, 1.000000000000000000 ) ) ;
#5779=ORIENTED_EDGE ( 'NONE', *, *, #15719, .F. ) ;
#5785=CARTESIAN_POINT ( 'NONE',  ( 1.871201846650637046, 31.30332840660451765, 6.000000000000000000 ) ) ;
#5791=AXIS2_PLACEMENT_3D ( 'NONE', #1894, #14271, #34861 ) ;
#5803=AXIS2_PLACEMENT_3D ( 'NONE', #18712, #24603, #22341 ) ;
#5804=ORIENTED_EDGE ( 'NONE', *, *, #16052, .F. ) ;
#5810=EDGE_CURVE ( 'NONE', #23095, #19744, #7857, .T. ) ;
#5813=ORIENTED_EDGE ( 'NONE', *, *, #35971, .F. ) ;
#5815=VECTOR ( 'NONE', #36658, 1000.000000000000000 ) ;
#5822=ADVANCED_FACE ( 'NONE', ( #31699 ), #25394, .F. ) ;
#5830=ORIENTED_EDGE ( 'NONE', *, *, #27631, .T. ) ;
#5833=CARTESIAN_POINT ( 'NONE',  ( 7.293999462566144842, 11.53598992149257008, 12.00000000000000000 ) ) ;
#5857=ORIENTED_EDGE ( 'NONE', *, *, #32366, .T. ) ;
#5858=DIRECTION ( 'NONE',  ( 0.000000000000000000, 0.000000000000000000, 1.000000000000000000 ) ) ;
#5861=DIRECTION ( 'NONE',  ( 1.000000000000000000, 0.000000000000000000, 0.000000000000000000 ) ) ;
#5862=AXIS2_PLACEMENT_3D ( 'NONE', #21011, #18564, #36843 ) ;
#5874=ORIENTED_EDGE ( 'NONE', *, *, #36728, .F. ) ;
#5876=DIRECTION ( 'NONE',  ( 0.000000000000000000, 0.000000000000000000, 1.000000000000000000 ) ) ;
#5879=VECTOR ( 'NONE', #27, 1000.000000000000000 ) ;
#5888=CARTESIAN_POINT ( 'NONE',  ( -10.78894649379783388, 21.72623886970244911, 6.000000000000000000 ) ) ;
#5910=CARTESIAN_POINT ( 'NONE',  ( -6.577547685840081648, 11.84256962714647798, 6.000000000000000000 ) ) ;
#5914=EDGE_CURVE ( 'NONE', #17958, #9757, #13691, .T. ) ;
#5916=EDGE_CURVE ( 'NONE', #29319, #2590, #24103, .T. ) ;
#5920=AXIS2_PLACEMENT_3D ( 'NONE', #28643, #6104, #30899 ) ;
#5924=DIRECTION ( 'NONE',  ( 1.000000000000000000, 0.000000000000000000, 0.000000000000000000 ) ) ;
#5930=CARTESIAN_POINT ( 'NONE',  ( -12.41268156625113406, 18.79179606750104981, 6.000000000000000000 ) ) ;
#5931=VERTEX_POINT ( 'NONE', #34550 ) ;
#5937=ORIENTED_EDGE ( 'NONE', *, *, #33881, .F. ) ;
#5940=DIRECTION ( 'NONE',  ( 0.000000000000000000, 0.000000000000000000, 1.000000000000000000 ) ) ;
#5960=FACE_BOUND ( 'NONE', #38459, .T. ) ;
#5972=CIRCLE ( 'NONE', #16358, 1.000000000000000888 ) ;
#5977=DIRECTION ( 'NONE',  ( 1.000000000000000000, 0.000000000000000000, 0.000000000000000000 ) ) ;
#5990=AXIS2_PLACEMENT_3D ( 'NONE', #38978, #23342, #19893 ) ;
#5991=CARTESIAN_POINT ( 'NONE',  ( 10.54146960747273987, 17.40487552589537401, 13.00000000000000178 ) ) ;
#5993=EDGE_LOOP ( 'NONE', ( #18579, #29785 ) ) ;
#6002=DIRECTION ( 'NONE',  ( 0.000000000000000000, 0.000000000000000000, 1.000000000000000000 ) ) ;
#6007=AXIS2_PLACEMENT_3D ( 'NONE', #33427, #27309, #30366 ) ;
#6008=CARTESIAN_POINT ( 'NONE',  ( -9.559512017365660697, 19.71884705062586107, 6.000000000000000000 ) ) ;
#6024=EDGE_CURVE ( 'NONE', #22329, #33038, #19546, .T. ) ;
#6027=EDGE_CURVE ( 'NONE', #14918, #32909, #20868, .T. ) ;
#6032=DIRECTION ( 'NONE',  ( 1.000000000000000000, 0.000000000000000000, 0.000000000000000000 ) ) ;
#6034=AXIS2_PLACEMENT_3D ( 'NONE', #31011, #34260, #30813 ) ;
#6049=EDGE_CURVE ( 'NONE', #6207, #28039, #3968, .T. ) ;
#6050=AXIS2_PLACEMENT_3D ( 'NONE', #6566, #34218, #37063 ) ;
#6057=ORIENTED_EDGE ( 'NONE', *, *, #26265, .F. ) ;
#6064=DIRECTION ( 'NONE',  ( 0.000000000000000000, 0.000000000000000000, 1.000000000000000000 ) ) ;
#6066=CARTESIAN_POINT ( 'NONE',  ( -6.706342468480190000, 20.64589803375067945, 12.00000000000000000 ) ) ;
#6074=PRODUCT_DEFINITION_FORMATION_WITH_SPECIFIED_SOURCE ( 'ANY', '', #13249, .NOT_KNOWN. ) ;
#6087=DIRECTION ( 'NONE',  ( 1.000000000000000000, 0.000000000000000000, 0.000000000000000000 ) ) ;
#6094=EDGE_CURVE ( 'NONE', #19619, #37255, #31242, .T. ) ;
#6101=ORIENTED_EDGE ( 'NONE', *, *, #14599, .T. ) ;
#6104=DIRECTION ( 'NONE',  ( 0.000000000000000000, 0.000000000000000000, 1.000000000000000000 ) ) ;
#6106=CIRCLE ( 'NONE', #28817, 1.000000000000000000 ) ;
#6108=ORIENTED_EDGE ( 'NONE', *, *, #8165, .F. ) ;
#6114=CIRCLE ( 'NONE', #6687, 1.000000000000000888 ) ;
#6118=FACE_OUTER_BOUND ( 'NONE', #22718, .T. ) ;
#6124=EDGE_CURVE ( 'NONE', #13841, #26783, #37069, .T. ) ;
#6132=FACE_BOUND ( 'NONE', #19679, .T. ) ;
#6133=AXIS2_PLACEMENT_3D ( 'NONE', #20317, #22950, #20520 ) ;
#6143=ADVANCED_FACE ( 'NONE', ( #1229 ), #10975, .F. ) ;
#6144=VERTEX_POINT ( 'NONE', #4059 ) ;
#6145=EDGE_CURVE ( 'NONE', #33348, #17668, #11118, .T. ) ;
#6154=DIRECTION ( 'NONE',  ( 0.000000000000000000, 0.000000000000000000, 1.000000000000000000 ) ) ;
#6155=VECTOR ( 'NONE', #18873, 1000.000000000000000 ) ;
#6156=CARTESIAN_POINT ( 'NONE',  ( 4.706335727061685681, 24.35410196624994583, 12.00000000000000000 ) ) ;
#6161=ADVANCED_FACE ( 'NONE', ( #35553 ), #4471, .F. ) ;
#6163=DIRECTION ( 'NONE',  ( 0.000000000000000000, 0.000000000000000000, 1.000000000000000000 ) ) ;
#6166=ORIENTED_EDGE ( 'NONE', *, *, #22769, .F. ) ;
#6168=DIRECTION ( 'NONE',  ( 0.000000000000000000, 0.000000000000000000, 1.000000000000000000 ) ) ;
#6173=ORIENTED_EDGE ( 'NONE', *, *, #6760, .F. ) ;
#6176=LINE ( 'NONE', #40101, #39919 ) ;
#6180=ORIENTED_EDGE ( 'NONE', *, *, #33279, .F. ) ;
#6184=CARTESIAN_POINT ( 'NONE',  ( -13.26585111513660031, 17.86474508437623143, 6.000000000000000000 ) ) ;
#6191=ORIENTED_EDGE ( 'NONE', *, *, #19850, .T. ) ;
#6193=LINE ( 'NONE', #18599, #12831 ) ;
#6200=AXIS2_PLACEMENT_3D ( 'NONE', #21066, #36504, #18221 ) ;
#6204=ORIENTED_EDGE ( 'NONE', *, *, #5914, .F. ) ;
#6207=VERTEX_POINT ( 'NONE', #33118 ) ;
#6208=DIRECTION ( 'NONE',  ( 0.000000000000000000, 0.000000000000000000, 1.000000000000000000 ) ) ;
#6209=APPLICATION_CONTEXT ( 'automotive_design' ) ;
#6211=CARTESIAN_POINT ( 'NONE',  ( -9.541476348891238857, 27.59512447410525127, 13.00000000000000178 ) ) ;
#6219=DIRECTION ( 'NONE',  ( 0.000000000000000000, 0.000000000000000000, 1.000000000000000000 ) ) ;
#6226=CIRCLE ( 'NONE', #20510, 1.000000000000000888 ) ;
#6228=AXIS2_PLACEMENT_3D ( 'NONE', #11133, #32477, #23521 ) ;
#6234=LINE ( 'NONE', #27968, #16615 ) ;
#6247=CARTESIAN_POINT ( 'NONE',  ( 7.917734535019441466, 14.47043272369397116, 12.00000000000000000 ) ) ;
#6249=CARTESIAN_POINT ( 'NONE',  ( 0.000000000000000000, 22.50000000000000355, 6.000000000000000000 ) ) ;
#6254=CIRCLE ( 'NONE', #14708, 1.000000000000000000 ) ;
#6256=CARTESIAN_POINT ( 'NONE',  ( 0.000000000000000000, 22.50000000000000355, 11.00000000000000178 ) ) ;
#6257=VERTEX_POINT ( 'NONE', #2035 ) ;
#6270=ORIENTED_EDGE ( 'NONE', *, *, #12514, .F. ) ;
#6272=LINE ( 'NONE', #27413, #2988 ) ;
#6275=DIRECTION ( 'NONE',  ( 0.000000000000000000, 0.000000000000000000, 1.000000000000000000 ) ) ;
#6282=ORIENTED_EDGE ( 'NONE', *, *, #22434, .F. ) ;
#6291=ORIENTED_EDGE ( 'NONE', *, *, #1589, .F. ) ;
#6293=FACE_OUTER_BOUND ( 'NONE', #25742, .T. ) ;
#6294=ORIENTED_EDGE ( 'NONE', *, *, #7647, .F. ) ;
#6300=CARTESIAN_POINT ( 'NONE',  ( -10.54147634889124063, 27.59512447410525127, 13.00000000000000178 ) ) ;
#6305=ORIENTED_EDGE ( 'NONE', *, *, #38945, .F. ) ;
#6306=CARTESIAN_POINT ( 'NONE',  ( -2.247473515615844075, 16.63111439559750693, 6.000000000000000000 ) ) ;
#6314=EDGE_CURVE ( 'NONE', #5046, #33648, #34492, .T. ) ;
#6326=FACE_BOUND ( 'NONE', #8981, .T. ) ;
#6333=VERTEX_POINT ( 'NONE', #23961 ) ;
#6351=CARTESIAN_POINT ( 'NONE',  ( -10.16521142134453548, 24.66068167190384841, 6.000000000000000000 ) ) ;
#6353=CIRCLE ( 'NONE', #10933, 1.000000000000000888 ) ;
#6355=DIRECTION ( 'NONE',  ( 0.000000000000000000, 0.000000000000000000, 1.000000000000000000 ) ) ;
#6358=FACE_OUTER_BOUND ( 'NONE', #3103, .T. ) ;
#6361=AXIS2_PLACEMENT_3D ( 'NONE', #16965, #23454, #19805 ) ;
#6366=EDGE_LOOP ( 'NONE', ( #15007, #2713 ) ) ;
#6373=EDGE_LOOP ( 'NONE', ( #21439, #39227 ) ) ;
#6378=ORIENTED_EDGE ( 'NONE', *, *, #2425, .F. ) ;
#6387=CARTESIAN_POINT ( 'NONE',  ( 2.229431105722923245, 20.49260818092372460, 13.00000000000000178 ) ) ;
#6391=VECTOR ( 'NONE', #16705, 1000.000000000000000 ) ;
#6393=AXIS2_PLACEMENT_3D ( 'NONE', #19333, #35383, #7541 ) ;
#6396=VERTEX_POINT ( 'NONE', #2429 ) ;
#6399=DIRECTION ( 'NONE',  ( 1.000000000000000000, 0.000000000000000000, 0.000000000000000000 ) ) ;
#6402=CARTESIAN_POINT ( 'NONE',  ( -11.77091082532341204, 29.60251629318183575, 6.000000000000000000 ) ) ;
#6412=FACE_OUTER_BOUND ( 'NONE', #12569, .T. ) ;
#6414=CIRCLE ( 'NONE', #34330, 1.000000000000000000 ) ;
#6418=ORIENTED_EDGE ( 'NONE', *, *, #11517, .F. ) ;
#6420=DIRECTION ( 'NONE',  ( 0.000000000000000000, 0.000000000000000000, 1.000000000000000000 ) ) ;
#6436=LINE ( 'NONE', #9703, #36160 ) ;
#6441=VERTEX_POINT ( 'NONE', #18666 ) ;
#6453=CARTESIAN_POINT ( 'NONE',  ( -2.494943660522439099, 10.76222879119470832, 13.00000000000000178 ) ) ;
#6456=ORIENTED_EDGE ( 'NONE', *, *, #9882, .T. ) ;
#6460=DIRECTION ( 'NONE',  ( 1.000000000000000000, 0.000000000000000000, 0.000000000000000000 ) ) ;
#6472=DIRECTION ( 'NONE',  ( 0.000000000000000000, 0.000000000000000000, 1.000000000000000000 ) ) ;
#6482=CYLINDRICAL_SURFACE ( 'NONE', #22483, 1.000000000000000000 ) ;
#6483=DIRECTION ( 'NONE',  ( 0.000000000000000000, 0.000000000000000000, 1.000000000000000000 ) ) ;
#6485=VERTEX_POINT ( 'NONE', #12957 ) ;
#6496=EDGE_CURVE ( 'NONE', #25213, #17512, #15666, .T. ) ;
#6504=DIRECTION ( 'NONE',  ( 1.000000000000000000, 0.000000000000000000, 0.000000000000000000 ) ) ;
#6506=DIRECTION ( 'NONE',  ( 1.000000000000000000, 0.000000000000000000, 0.000000000000000000 ) ) ;
#6512=CARTESIAN_POINT ( 'NONE',  ( -4.100643064501314328, 15.70406341247269211, 12.00000000000000000 ) ) ;
#6513=ORIENTED_EDGE ( 'NONE', *, *, #10295, .T. ) ;
#6519=AXIS2_PLACEMENT_3D ( 'NONE', #1525, #26307, #6998 ) ;
#6526=FACE_BOUND ( 'NONE', #20907, .T. ) ;
#6533=CYLINDRICAL_SURFACE ( 'NONE', #37520, 1.000000000000000000 ) ;
#6551=CARTESIAN_POINT ( 'NONE',  ( 10.78893975237932956, 23.27376113029817617, 6.000000000000000000 ) ) ;
#6552=FACE_OUTER_BOUND ( 'NONE', #5160, .T. ) ;
#6555=CYLINDRICAL_SURFACE ( 'NONE', #9904, 1.000000000000000000 ) ;
#6557=DIRECTION ( 'NONE',  ( 0.000000000000000000, 0.000000000000000000, 1.000000000000000000 ) ) ;
#6566=CARTESIAN_POINT ( 'NONE',  ( 0.000000000000000000, 22.50000000000000355, 12.00000000000000000 ) ) ;
#6569=DIRECTION ( 'NONE',  ( 1.000000000000000000, 0.000000000000000000, 0.000000000000000000 ) ) ;
#6573=ORIENTED_EDGE ( 'NONE', *, *, #17735, .T. ) ;
#6582=DIRECTION ( 'NONE',  ( 1.000000000000000000, 0.000000000000000000, 0.000000000000000000 ) ) ;
#6583=CARTESIAN_POINT ( 'NONE',  ( -12.01838097023000529, 23.73363068877903359, 13.00000000000000178 ) ) ;
#6591=EDGE_CURVE ( 'NONE', #8118, #10191, #28016, .T. ) ;
#6593=CYLINDRICAL_SURFACE ( 'NONE', #3102, 1.000000000000000000 ) ;
#6595=DIRECTION ( 'NONE',  ( 0.000000000000000000, 0.000000000000000000, 1.000000000000000000 ) ) ;
#6596=CARTESIAN_POINT ( 'NONE',  ( 12.03640989728592459, 29.14264673470096767, 12.00000000000000000 ) ) ;
#6600=CYLINDRICAL_SURFACE ( 'NONE', #1270, 1.000000000000000888 ) ;
#6603=EDGE_CURVE ( 'NONE', #342, #22756, #9324, .T. ) ;
#6604=DIRECTION ( 'NONE',  ( 1.000000000000000000, 0.000000000000000000, 0.000000000000000000 ) ) ;
#6607=EDGE_LOOP ( 'NONE', ( #27878, #30510 ) ) ;
#6610=CYLINDRICAL_SURFACE ( 'NONE', #29603, 1.000000000000000888 ) ;
#6629=VERTEX_POINT ( 'NONE', #37552 ) ;
#6632=VECTOR ( 'NONE', #40044, 1000.000000000000000 ) ;
#6649=ORIENTED_EDGE ( 'NONE', *, *, #11291, .T. ) ;
#6653=CARTESIAN_POINT ( 'NONE',  ( 6.440829913680675034, 10.60893893836775348, 6.000000000000000000 ) ) ;
#6680=VERTEX_POINT ( 'NONE', #4823 ) ;
#6684=VERTEX_POINT ( 'NONE', #17227 ) ;
#6687=AXIS2_PLACEMENT_3D ( 'NONE', #30011, #35908, #11528 ) ;
#6696=CIRCLE ( 'NONE', #35243, 1.000000000000000000 ) ;
#6697=DIRECTION ( 'NONE',  ( 1.000000000000000000, 0.000000000000000000, 0.000000000000000000 ) ) ;
#6698=EDGE_LOOP ( 'NONE', ( #641, #11607 ) ) ;
#6715=DIRECTION ( 'NONE',  ( 0.000000000000000000, 0.000000000000000000, 1.000000000000000000 ) ) ;
#6717=ORIENTED_EDGE ( 'NONE', *, *, #30221, .T. ) ;
#6720=FACE_BOUND ( 'NONE', #22288, .T. ) ;
#6731=ORIENTED_EDGE ( 'NONE', *, *, #20895, .F. ) ;
#6739=ORIENTED_EDGE ( 'NONE', *, *, #14132, .F. ) ;
#6743=CARTESIAN_POINT ( 'NONE',  ( 8.559505275947156377, 25.28115294937476065, 6.000000000000000000 ) ) ;
#6746=EDGE_CURVE ( 'NONE', #32554, #32493, #7054, .T. ) ;
#6749=FACE_BOUND ( 'NONE', #21386, .T. ) ;
#6760=EDGE_CURVE ( 'NONE', #39486, #14121, #11103, .T. ) ;
#6763=ORIENTED_EDGE ( 'NONE', *, *, #19306, .T. ) ;
#6764=DIRECTION ( 'NONE',  ( 1.000000000000000000, 0.000000000000000000, 0.000000000000000000 ) ) ;
#6765=ORIENTED_EDGE ( 'NONE', *, *, #11156, .F. ) ;
#6770=ORIENTED_EDGE ( 'NONE', *, *, #17421, .T. ) ;
#6778=CYLINDRICAL_SURFACE ( 'NONE', #34814, 18.00000000000000000 ) ;
#6785=ORIENTED_EDGE ( 'NONE', *, *, #8064, .F. ) ;
#6786=AXIS2_PLACEMENT_3D ( 'NONE', #21074, #36910, #14577 ) ;
#6790=CIRCLE ( 'NONE', #7464, 1.000000000000000000 ) ;
#6801=CARTESIAN_POINT ( 'NONE',  ( -1.623738443162547007, 19.56555719779890978, 12.00000000000000000 ) ) ;
#6811=EDGE_CURVE ( 'NONE', #14009, #7, #10416, .T. ) ;
#6816=EDGE_LOOP ( 'NONE', ( #18602, #26748 ) ) ;
#6818=LINE ( 'NONE', #4182, #9483 ) ;
#6833=VERTEX_POINT ( 'NONE', #28799 ) ;
#6834=FACE_OUTER_BOUND ( 'NONE', #3650, .T. ) ;
#6845=AXIS2_PLACEMENT_3D ( 'NONE', #18228, #27760, #11531 ) ;
#6846=CIRCLE ( 'NONE', #12717, 1.000000000000000888 ) ;
#6882=AXIS2_PLACEMENT_3D ( 'NONE', #18084, #12175, #27215 ) ;
#6884=ORIENTED_EDGE ( 'NONE', *, *, #15345, .T. ) ;
#6887=EDGE_CURVE ( 'NONE', #6898, #7015, #30560, .T. ) ;
#6888=ORIENTED_EDGE ( 'NONE', *, *, #20284, .F. ) ;
#6898=VERTEX_POINT ( 'NONE', #29806 ) ;
#6901=DIRECTION ( 'NONE',  ( 0.000000000000000000, 0.000000000000000000, 1.000000000000000000 ) ) ;
#6912=EDGE_LOOP ( 'NONE', ( #36040, #6765 ) ) ;
#6918=VERTEX_POINT ( 'NONE', #36505 ) ;
#6921=FACE_BOUND ( 'NONE', #18921, .T. ) ;
#6924=ORIENTED_EDGE ( 'NONE', *, *, #19107, .F. ) ;
#6926=LINE ( 'NONE', #650, #18727 ) ;
#6927=CARTESIAN_POINT ( 'NONE',  ( -12.03641663870442713, 15.85735326529964873, 13.00000000000000178 ) ) ;
#6935=LINE ( 'NONE', #34784, #26533 ) ;
#6938=ORIENTED_EDGE ( 'NONE', *, *, #34399, .F. ) ;
#6945=FACE_BOUND ( 'NONE', #37491, .T. ) ;
#6962=CIRCLE ( 'NONE', #25801, 1.000000000000000000 ) ;
#6971=DIRECTION ( 'NONE',  ( 0.000000000000000000, 0.000000000000000000, 1.000000000000000000 ) ) ;
#6975=CARTESIAN_POINT ( 'NONE',  ( 9.183240348400453001, 28.21559575157615996, 13.00000000000000178 ) ) ;
#6977=FACE_OUTER_BOUND ( 'NONE', #20264, .T. ) ;
#6986=AXIS2_PLACEMENT_3D ( 'NONE', #35586, #25423, #7134 ) ;
#6987=AXIS2_PLACEMENT_3D ( 'NONE', #24039, #1710, #5153 ) ;
#6998=DIRECTION ( 'NONE',  ( 1.000000000000000000, 0.000000000000000000, 0.000000000000000000 ) ) ;
#7007=ORIENTED_EDGE ( 'NONE', *, *, #17824, .T. ) ;
#7015=VERTEX_POINT ( 'NONE', #19202 ) ;
#7022=AXIS2_PLACEMENT_3D ( 'NONE', #1454, #34777, #10193 ) ;
#7026=ADVANCED_FACE ( 'NONE', ( #30810 ), #26657, .T. ) ;
#7033=ORIENTED_EDGE ( 'NONE', *, *, #15425, .T. ) ;
#7035=VECTOR ( 'NONE', #23941, 1000.000000000000000 ) ;
#7037=ORIENTED_EDGE ( 'NONE', *, *, #39171, .T. ) ;
#7046=DIRECTION ( 'NONE',  ( 1.000000000000000000, 0.000000000000000000, 0.000000000000000000 ) ) ;
#7051=VERTEX_POINT ( 'NONE', #325 ) ;
#7053=DIRECTION ( 'NONE',  ( 1.000000000000000000, 0.000000000000000000, 0.000000000000000000 ) ) ;
#7054=LINE ( 'NONE', #19867, #11735 ) ;
#7055=AXIS2_PLACEMENT_3D ( 'NONE', #21154, #27447, #11419 ) ;
#7056=CARTESIAN_POINT ( 'NONE',  ( -9.541476348891238857, 27.59512447410525127, 13.00000000000000178 ) ) ;
#7070=CARTESIAN_POINT ( 'NONE',  ( -9.559512017365660697, 19.71884705062586107, 13.00000000000000178 ) ) ;
#7077=EDGE_LOOP ( 'NONE', ( #13585, #2214, #19534, #37744 ) ) ;
#7079=CIRCLE ( 'NONE', #14225, 1.000000000000000000 ) ;
#7081=ORIENTED_EDGE ( 'NONE', *, *, #28529, .F. ) ;
#7086=VECTOR ( 'NONE', #28247, 1000.000000000000000 ) ;
#7088=ORIENTED_EDGE ( 'NONE', *, *, #35796, .T. ) ;
#7093=ORIENTED_EDGE ( 'NONE', *, *, #24528, .T. ) ;
#7107=FACE_OUTER_BOUND ( 'NONE', #7236, .T. ) ;
#7110=ORIENTED_EDGE ( 'NONE', *, *, #15720, .T. ) ;
#7124=ORIENTED_EDGE ( 'NONE', *, *, #38945, .T. ) ;
#7127=FACE_BOUND ( 'NONE', #36877, .T. ) ;
#7131=ORIENTED_EDGE ( 'NONE', *, *, #14106, .F. ) ;
#7133=CYLINDRICAL_SURFACE ( 'NONE', #6393, 1.000000000000000888 ) ;
#7134=DIRECTION ( 'NONE',  ( 1.000000000000000000, 0.000000000000000000, 0.000000000000000000 ) ) ;
#7138=VERTEX_POINT ( 'NONE', #31200 ) ;
#7146=EDGE_CURVE ( 'NONE', #22293, #2500, #36384, .T. ) ;
#7153=FACE_BOUND ( 'NONE', #8767, .T. ) ;
#7165=EDGE_CURVE ( 'NONE', #33185, #15751, #1350, .T. ) ;
#7171=CIRCLE ( 'NONE', #12375, 1.000000000000000000 ) ;
#7177=VERTEX_POINT ( 'NONE', #922 ) ;
#7180=CARTESIAN_POINT ( 'NONE',  ( 4.440829913680675034, 10.60893893836775348, 13.00000000000000178 ) ) ;
#7182=ORIENTED_EDGE ( 'NONE', *, *, #1715, .T. ) ;
#7186=ORIENTED_EDGE ( 'NONE', *, *, #20126, .F. ) ;
#7189=AXIS2_PLACEMENT_3D ( 'NONE', #31106, #6901, #6504 ) ;
#7195=CARTESIAN_POINT ( 'NONE',  ( -11.78894649379783388, 21.72623886970244911, 6.000000000000000000 ) ) ;
#7199=DIRECTION ( 'NONE',  ( 0.000000000000000000, 0.000000000000000000, 1.000000000000000000 ) ) ;
#7201=ORIENTED_EDGE ( 'NONE', *, *, #39775, .T. ) ;
#7202=CARTESIAN_POINT ( 'NONE',  ( -15.21690460405485545, 17.55572914666943873, 13.00000000000000178 ) ) ;
#7213=AXIS2_PLACEMENT_3D ( 'NONE', #39035, #19544, #32758 ) ;
#7217=ORIENTED_EDGE ( 'NONE', *, *, #11891, .F. ) ;
#7227=VERTEX_POINT ( 'NONE', #7610 ) ;
#7236=EDGE_LOOP ( 'NONE', ( #16542, #15933, #4092, #21485 ) ) ;
#7238=CYLINDRICAL_SURFACE ( 'NONE', #37519, 1.000000000000000000 ) ;
#7243=ORIENTED_EDGE ( 'NONE', *, *, #17076, .T. ) ;
#7244=ORIENTED_EDGE ( 'NONE', *, *, #17376, .T. ) ;
#7245=DIRECTION ( 'NONE',  ( 0.000000000000000000, 0.000000000000000000, 1.000000000000000000 ) ) ;
#7249=EDGE_CURVE ( 'NONE', #5684, #8671, #39, .T. ) ;
#7254=CARTESIAN_POINT ( 'NONE',  ( 15.26584437371809955, 27.13525491562438319, 12.00000000000000000 ) ) ;
#7264=CARTESIAN_POINT ( 'NONE',  ( -5.688306800005769048, 28.52217545723006609, 12.00000000000000000 ) ) ;
#7267=DIRECTION ( 'NONE',  ( 1.000000000000000000, 0.000000000000000000, 0.000000000000000000 ) ) ;
#7269=CIRCLE ( 'NONE', #18342, 1.000000000000000888 ) ;
#7274=CARTESIAN_POINT ( 'NONE',  ( -8.541476348891238857, 27.59512447410525127, 12.00000000000000000 ) ) ;
#7276=ADVANCED_FACE ( 'NONE', ( #19811 ), #16565, .F. ) ;
#7288=VERTEX_POINT ( 'NONE', #32413 ) ;
#7296=ADVANCED_FACE ( 'NONE', ( #37888 ), #32203, .F. ) ;
#7298=DIRECTION ( 'NONE',  ( 1.000000000000000000, 0.000000000000000000, 0.000000000000000000 ) ) ;
#7299=VERTEX_POINT ( 'NONE', #7202 ) ;
#7302=DIRECTION ( 'NONE',  ( 0.000000000000000000, 0.000000000000000000, 1.000000000000000000 ) ) ;
#7323=ORIENTED_EDGE ( 'NONE', *, *, #24649, .T. ) ;
#7328=CLOSED_SHELL ( 'NONE', ( #19512, #35712, #7860, #18283, #28751, #11651, #1310, #25290, #1079, #15623, #36935, #18090, #13256, #7398, #25434, #31870, #20211, #9544, #25177, #4879, #12888, #15772, #39894, #23536, #33531, #29852, #37914, #15502, #24443, #31344, #22430, #33732, #18357, #11268, #11600, #26388, #30001, #478, #36148, #6161, #19178, #10551, #34248, #28379, #21835, #19847, #32038, #22611, #21751, #26766, #4094, #13648, #5418, #26301, #16496, #37401, #16950, #16511, #13368, #8135, #30419, #9249, #27582, #35968, #801, #31741, #5215, #1076, #36303, #1356, #33494, #10879, #14546, #32951, #31359, #39927, #18457, #37809, #3897, #21256, #10858, #32666, #15987, #5640, #36239, #8876, #1504, #20165, #7296, #13105, #21528, #5687, #17074, #7026, #11290, #34196, #22166, #20157, #25646, #26236, #869, #5116, #223, #21390, #13800, #11134, #5298, #16025, #19956, #39534, #30417, #4320, #39578, #28223, #23407, #2811, #31013, #27140, #12111, #29754, #9750, #11034, #21692, #26493, #28637, #16872, #4802, #1940, #422, #33508, #35487, #7661, #10982, #5671, #5196, #23925, #32650, #11515, #33947, #36202, #37947, #26793, #26249, #19685, #27347, #26024, #39931, #6143, #40052, #29600, #36976, #7276, #35150, #17988, #17775, #32970, #12949, #33900, #31509, #19760, #39190, #24242, #8570, #7540, #18446, #5759, #20587, #15397, #24998, #24564, #3669, #16278, #31390, #28427, #27730, #39681, #3498, #24883, #39326, #27494, #22686, #11616, #34724, #5822, #23094, #20561, #31941, #39430, #14104, #16831, #31441, #27902, #14359 ) ) ;
#7337=VERTEX_POINT ( 'NONE', #7815 ) ;
#7349=EDGE_CURVE ( 'NONE', #4871, #36787, #4153, .T. ) ;
#7351=DIRECTION ( 'NONE',  ( 0.000000000000000000, 0.000000000000000000, 1.000000000000000000 ) ) ;
#7352=EDGE_CURVE ( 'NONE', #37261, #16796, #1937, .T. ) ;
#7353=FACE_BOUND ( 'NONE', #6366, .T. ) ;
#7367=ORIENTED_EDGE ( 'NONE', *, *, #27650, .F. ) ;
#7385=DIRECTION ( 'NONE',  ( 1.000000000000000000, 0.000000000000000000, 0.000000000000000000 ) ) ;
#7398=ADVANCED_FACE ( 'NONE', ( #26909 ), #14920, .F. ) ;
#7404=CARTESIAN_POINT ( 'NONE',  ( 12.03640989728592459, 29.14264673470096767, 6.000000000000000000 ) ) ;
#7418=EDGE_LOOP ( 'NONE', ( #1240, #40007 ) ) ;
#7426=EDGE_CURVE ( 'NONE', #24952, #36412, #20294, .T. ) ;
#7427=CIRCLE ( 'NONE', #12622, 1.000000000000000000 ) ;
#7431=ORIENTED_EDGE ( 'NONE', *, *, #25689, .T. ) ;
#7436=COLOUR_RGB ( '', 0.40784314, 0.44705882, 0.49803922) ;
#7440=VECTOR ( 'NONE', #35756, 1000.000000000000000 ) ;
#7450=FACE_OUTER_BOUND ( 'NONE', #37234, .T. ) ;
#7451=FACE_OUTER_BOUND ( 'NONE', #8880, .T. ) ;
#7460=LINE ( 'NONE', #11125, #30109 ) ;
#7464=AXIS2_PLACEMENT_3D ( 'NONE', #35097, #26753, #1174 ) ;
#7479=EDGE_CURVE ( 'NONE', #488, #12698, #36657, .T. ) ;
#7481=CARTESIAN_POINT ( 'NONE',  ( -5.330077540933487512, 17.71145523154927659, 12.00000000000000000 ) ) ;
#7483=EDGE_LOOP ( 'NONE', ( #14879, #33556, #36634, #2764 ) ) ;
#7495=ORIENTED_EDGE ( 'NONE', *, *, #31835, .T. ) ;
#7502=DIRECTION ( 'NONE',  ( 1.000000000000000000, 0.000000000000000000, 0.000000000000000000 ) ) ;
#7506=ORIENTED_EDGE ( 'NONE', *, *, #34223, .F. ) ;
#7508=DIRECTION ( 'NONE',  ( 1.000000000000000000, 0.000000000000000000, 0.000000000000000000 ) ) ;
#7509=EDGE_CURVE ( 'NONE', #29377, #32505, #16492, .T. ) ;
#7514=CARTESIAN_POINT ( 'NONE',  ( 13.01837422881150452, 21.26636931122159169, 12.00000000000000000 ) ) ;
#7534=DIRECTION ( 'NONE',  ( 0.000000000000000000, 0.000000000000000000, 1.000000000000000000 ) ) ;
#7537=ORIENTED_EDGE ( 'NONE', *, *, #25894, .T. ) ;
#7540=ADVANCED_FACE ( 'NONE', ( #8427 ), #3319, .F. ) ;
#7541=DIRECTION ( 'NONE',  ( 1.000000000000000000, 0.000000000000000000, 0.000000000000000000 ) ) ;
#7556=AXIS2_PLACEMENT_3D ( 'NONE', #35268, #23071, #32432 ) ;
#7557=DIRECTION ( 'NONE',  ( 0.000000000000000000, 0.000000000000000000, 1.000000000000000000 ) ) ;
#7559=EDGE_CURVE ( 'NONE', #24946, #8057, #28715, .T. ) ;
#7562=CARTESIAN_POINT ( 'NONE',  ( 5.706335727061685681, 24.35410196624994583, 6.000000000000000000 ) ) ;
#7572=CYLINDRICAL_SURFACE ( 'NONE', #12054, 1.000000000000000888 ) ;
#7574=VERTEX_POINT ( 'NONE', #27506 ) ;
#7583=AXIS2_PLACEMENT_3D ( 'NONE', #4031, #23126, #13378 ) ;
#7589=ORIENTED_EDGE ( 'NONE', *, *, #23139, .T. ) ;
#7596=AXIS2_PLACEMENT_3D ( 'NONE', #20269, #29606, #27162 ) ;
#7604=AXIS2_PLACEMENT_3D ( 'NONE', #11658, #24040, #8601 ) ;
#7609=EDGE_LOOP ( 'NONE', ( #16733, #3805 ) ) ;
#7610=CARTESIAN_POINT ( 'NONE',  ( 1.981960960816328887, 14.62372257652092422, 12.00000000000000000 ) ) ;
#7611=DIRECTION ( 'NONE',  ( 0.000000000000000000, 0.000000000000000000, 1.000000000000000000 ) ) ;
#7613=VECTOR ( 'NONE', #36894, 1000.000000000000000 ) ;
#7618=DIRECTION ( 'NONE',  ( 0.000000000000000000, 0.000000000000000000, 1.000000000000000000 ) ) ;
#7629=DIRECTION ( 'NONE',  ( 1.000000000000000000, 0.000000000000000000, 0.000000000000000000 ) ) ;
#7631=EDGE_CURVE ( 'NONE', #31950, #26852, #15519, .T. ) ;
#7637=EDGE_CURVE ( 'NONE', #7051, #32832, #11216, .T. ) ;
#7641=CARTESIAN_POINT ( 'NONE',  ( 6.577540944421576441, 33.15743037285414374, 13.00000000000000178 ) ) ;
#7646=CIRCLE ( 'NONE', #20008, 1.000000000000000000 ) ;
#7647=EDGE_CURVE ( 'NONE', #14056, #33800, #29391, .T. ) ;
#7649=ORIENTED_EDGE ( 'NONE', *, *, #7637, .T. ) ;
#7653=CARTESIAN_POINT ( 'NONE',  ( -4.440836655099179353, 34.39106106163288246, 12.00000000000000000 ) ) ;
#7657=ORIENTED_EDGE ( 'NONE', *, *, #36728, .T. ) ;
#7659=CARTESIAN_POINT ( 'NONE',  ( -5.440836655099179353, 34.39106106163288246, 6.000000000000000000 ) ) ;
#7661=ADVANCED_FACE ( 'NONE', ( #6358 ), #6555, .F. ) ;
#7668=DIRECTION ( 'NONE',  ( 0.000000000000000000, 0.000000000000000000, 1.000000000000000000 ) ) ;
#7669=DIRECTION ( 'NONE',  ( 1.000000000000000000, 0.000000000000000000, 0.000000000000000000 ) ) ;
#7674=ORIENTED_EDGE ( 'NONE', *, *, #28279, .F. ) ;
#7676=CARTESIAN_POINT ( 'NONE',  ( 7.577540944421576441, 33.15743037285414374, 12.00000000000000000 ) ) ;
#7681=VECTOR ( 'NONE', #5858, 1000.000000000000000 ) ;
#7683=CARTESIAN_POINT ( 'NONE',  ( -10.77091082532341204, 29.60251629318183575, 6.000000000000000000 ) ) ;
#7696=ORIENTED_EDGE ( 'NONE', *, *, #35695, .F. ) ;
#7697=CARTESIAN_POINT ( 'NONE',  ( -2.835137251120299684, 29.44922644035488446, 6.000000000000000000 ) ) ;
#7704=AXIS2_PLACEMENT_3D ( 'NONE', #11733, #18035, #23520 ) ;
#7705=VERTEX_POINT ( 'NONE', #24854 ) ;
#7708=AXIS2_PLACEMENT_3D ( 'NONE', #21598, #16106, #28490 ) ;
#7715=DIRECTION ( 'NONE',  ( 0.000000000000000000, 0.000000000000000000, 1.000000000000000000 ) ) ;
#7716=EDGE_CURVE ( 'NONE', #4829, #12491, #37250, .T. ) ;
#7721=DIRECTION ( 'NONE',  ( 1.000000000000000000, 0.000000000000000000, 0.000000000000000000 ) ) ;
#7722=DIRECTION ( 'NONE',  ( 0.000000000000000000, 0.000000000000000000, 1.000000000000000000 ) ) ;
#7727=ORIENTED_EDGE ( 'NONE', *, *, #9833, .T. ) ;
#7737=FACE_BOUND ( 'NONE', #6607, .T. ) ;
#7745=ORIENTED_EDGE ( 'NONE', *, *, #39800, .T. ) ;
#7748=VERTEX_POINT ( 'NONE', #38202 ) ;
#7772=EDGE_LOOP ( 'NONE', ( #30220, #7431, #10147, #1607 ) ) ;
#7774=ORIENTED_EDGE ( 'NONE', *, *, #35230, .F. ) ;
#7781=ORIENTED_EDGE ( 'NONE', *, *, #683, .F. ) ;
#7792=VERTEX_POINT ( 'NONE', #26208 ) ;
#7795=EDGE_CURVE ( 'NONE', #8150, #26803, #22883, .T. ) ;
#7807=AXIS2_PLACEMENT_3D ( 'NONE', #35347, #37989, #16867 ) ;
#7810=CYLINDRICAL_SURFACE ( 'NONE', #15599, 1.000000000000000000 ) ;
#7815=CARTESIAN_POINT ( 'NONE',  ( -8.541476348891238857, 27.59512447410525127, 13.00000000000000178 ) ) ;
#7816=DIRECTION ( 'NONE',  ( 0.000000000000000000, 0.000000000000000000, 1.000000000000000000 ) ) ;
#7825=CARTESIAN_POINT ( 'NONE',  ( 4.706335727061685681, 24.35410196624994583, 6.000000000000000000 ) ) ;
#7827=ORIENTED_EDGE ( 'NONE', *, *, #11316, .T. ) ;
#7831=DIRECTION ( 'NONE',  ( 1.000000000000000000, 0.000000000000000000, 0.000000000000000000 ) ) ;
#7840=DIRECTION ( 'NONE',  ( 0.000000000000000000, 0.000000000000000000, 1.000000000000000000 ) ) ;
#7841=DIRECTION ( 'NONE',  ( 1.000000000000000000, 0.000000000000000000, 0.000000000000000000 ) ) ;
#7843=DIRECTION ( 'NONE',  ( 0.000000000000000000, 0.000000000000000000, 1.000000000000000000 ) ) ;
#7844=ORIENTED_EDGE ( 'NONE', *, *, #19715, .T. ) ;
#7853=EDGE_LOOP ( 'NONE', ( #885, #1750, #30592, #3439 ) ) ;
#7854=CYLINDRICAL_SURFACE ( 'NONE', #35316, 1.000000000000000000 ) ;
#7855=DIRECTION ( 'NONE',  ( 1.000000000000000000, 0.000000000000000000, 0.000000000000000000 ) ) ;
#7857=CIRCLE ( 'NONE', #7189, 1.000000000000000888 ) ;
#7859=ORIENTED_EDGE ( 'NONE', *, *, #25017, .T. ) ;
#7860=ADVANCED_FACE ( 'NONE', ( #19919 ), #17486, .F. ) ;
#7862=DIRECTION ( 'NONE',  ( 1.000000000000000000, 0.000000000000000000, 0.000000000000000000 ) ) ;
#7865=DIRECTION ( 'NONE',  ( 1.000000000000000000, 0.000000000000000000, 0.000000000000000000 ) ) ;
#7870=EDGE_CURVE ( 'NONE', #2515, #7748, #33323, .T. ) ;
#7873=CARTESIAN_POINT ( 'NONE',  ( -11.41268156625113406, 18.79179606750104981, 13.00000000000000178 ) ) ;
#7887=EDGE_CURVE ( 'NONE', #19767, #36141, #31353, .T. ) ;
#7889=EDGE_CURVE ( 'NONE', #6833, #25338, #17081, .T. ) ;
#7891=CARTESIAN_POINT ( 'NONE',  ( 12.41267482483262796, 26.20820393249957192, 12.00000000000000000 ) ) ;
#7896=EDGE_LOOP ( 'NONE', ( #17922, #37279, #31913, #19416 ) ) ;
#7900=EDGE_LOOP ( 'NONE', ( #17195, #29897, #25908, #22234 ) ) ;
#7902=AXIS2_PLACEMENT_3D ( 'NONE', #3842, #9747, #38171 ) ;
#7906=CYLINDRICAL_SURFACE ( 'NONE', #26043, 1.000000000000000000 ) ;
#7914=DIRECTION ( 'NONE',  ( 1.000000000000000000, 0.000000000000000000, 0.000000000000000000 ) ) ;
#7915=DIRECTION ( 'NONE',  ( 0.000000000000000000, 0.000000000000000000, 1.000000000000000000 ) ) ;
#7932=LINE ( 'NONE', #1650, #2945 ) ;
#7933=FACE_BOUND ( 'NONE', #30692, .T. ) ;
#7939=DIRECTION ( 'NONE',  ( 1.000000000000000000, 0.000000000000000000, 0.000000000000000000 ) ) ;
#7943=ORIENTED_EDGE ( 'NONE', *, *, #17665, .F. ) ;
#7945=DIRECTION ( 'NONE',  ( 1.000000000000000000, 0.000000000000000000, 0.000000000000000000 ) ) ;
#7955=CARTESIAN_POINT ( 'NONE',  ( -12.39464589777671044, 26.66807349098043289, 6.000000000000000000 ) ) ;
#7956=EDGE_LOOP ( 'NONE', ( #19320, #23627, #10427, #10080 ) ) ;
#7966=DIRECTION ( 'NONE',  ( 0.000000000000000000, 0.000000000000000000, 1.000000000000000000 ) ) ;
#7967=VERTEX_POINT ( 'NONE', #23369 ) ;
#7983=ORIENTED_EDGE ( 'NONE', *, *, #13870, .T. ) ;
#7988=ORIENTED_EDGE ( 'NONE', *, *, #6094, .F. ) ;
#7992=CIRCLE ( 'NONE', #35225, 1.000000000000000000 ) ;
#7998=EDGE_CURVE ( 'NONE', #30397, #6485, #1519, .T. ) ;
#8006=CIRCLE ( 'NONE', #35916, 1.000000000000000888 ) ;
#8007=DIRECTION ( 'NONE',  ( 0.000000000000000000, 0.000000000000000000, 1.000000000000000000 ) ) ;
#8011=CARTESIAN_POINT ( 'NONE',  ( -6.312041872459064784, 25.58773265502866678, 12.00000000000000000 ) ) ;
#8014=CARTESIAN_POINT ( 'NONE',  ( -1.229437847141422901, 24.50739181907689712, 6.000000000000000000 ) ) ;
#8021=CARTESIAN_POINT ( 'NONE',  ( -0.2655091840902661926, 8.754836972118123839, 12.00000000000000000 ) ) ;
#8022=VERTEX_POINT ( 'NONE', #15021 ) ;
#8029=EDGE_LOOP ( 'NONE', ( #38816, #17314, #3759, #12872 ) ) ;
#8031=ORIENTED_EDGE ( 'NONE', *, *, #11316, .F. ) ;
#8039=ORIENTED_EDGE ( 'NONE', *, *, #15345, .F. ) ;
#8042=CARTESIAN_POINT ( 'NONE',  ( -6.688306800005769048, 28.52217545723006609, 6.000000000000000000 ) ) ;
#8043=DIRECTION ( 'NONE',  ( 1.000000000000000000, 0.000000000000000000, 0.000000000000000000 ) ) ;
#8044=EDGE_LOOP ( 'NONE', ( #23833, #10354 ) ) ;
#8055=CYLINDRICAL_SURFACE ( 'NONE', #2443, 1.000000000000000000 ) ;
#8057=VERTEX_POINT ( 'NONE', #21121 ) ;
#8060=DIRECTION ( 'NONE',  ( 0.000000000000000000, 0.000000000000000000, 1.000000000000000000 ) ) ;
#8063=CARTESIAN_POINT ( 'NONE',  ( -11.14717575287011542, 32.53695909538323860, 6.000000000000000000 ) ) ;
#8064=EDGE_CURVE ( 'NONE', #25619, #20347, #23566, .T. ) ;
#8069=DIRECTION ( 'NONE',  ( 0.000000000000000000, 0.000000000000000000, 1.000000000000000000 ) ) ;
#8070=AXIS2_PLACEMENT_3D ( 'NONE', #14221, #17694, #17491 ) ;
#8073=EDGE_LOOP ( 'NONE', ( #3596, #35127 ) ) ;
#8082=AXIS2_PLACEMENT_3D ( 'NONE', #19806, #13293, #35042 ) ;
#8087=CARTESIAN_POINT ( 'NONE',  ( 9.541469607472739867, 17.40487552589537401, 6.000000000000000000 ) ) ;
#8090=VERTEX_POINT ( 'NONE', #27214 ) ;
#8091=EDGE_CURVE ( 'NONE', #28113, #12049, #25482, .T. ) ;
#8096=ORIENTED_EDGE ( 'NONE', *, *, #24041, .F. ) ;
#8098=VERTEX_POINT ( 'NONE', #39337 ) ;
#8102=DIRECTION ( 'NONE',  ( 0.000000000000000000, 0.000000000000000000, 1.000000000000000000 ) ) ;
#8110=ORIENTED_EDGE ( 'NONE', *, *, #30287, .F. ) ;
#8112=CARTESIAN_POINT ( 'NONE',  ( -13.39464589777671044, 26.66807349098043289, 6.000000000000000000 ) ) ;
#8113=DIRECTION ( 'NONE',  ( 0.000000000000000000, 0.000000000000000000, 1.000000000000000000 ) ) ;
#8118=VERTEX_POINT ( 'NONE', #33063 ) ;
#8135=ADVANCED_FACE ( 'NONE', ( #4611 ), #14557, .F. ) ;
#8136=DIRECTION ( 'NONE',  ( 0.000000000000000000, 0.000000000000000000, 1.000000000000000000 ) ) ;
#8137=AXIS2_PLACEMENT_3D ( 'NONE', #30809, #9862, #19006 ) ;
#8140=CARTESIAN_POINT ( 'NONE',  ( -8.559512017365658920, 19.71884705062586107, 12.00000000000000000 ) ) ;
#8143=EDGE_CURVE ( 'NONE', #1258, #25235, #6696, .T. ) ;
#8147=ORIENTED_EDGE ( 'NONE', *, *, #36682, .T. ) ;
#8150=VERTEX_POINT ( 'NONE', #7653 ) ;
#8154=ORIENTED_EDGE ( 'NONE', *, *, #1889, .F. ) ;
#8165=EDGE_CURVE ( 'NONE', #33425, #3338, #17113, .T. ) ;
#8168=VECTOR ( 'NONE', #31025, 1000.000000000000000 ) ;
#8171=AXIS2_PLACEMENT_3D ( 'NONE', #18871, #10324, #31262 ) ;
#8175=CARTESIAN_POINT ( 'NONE',  ( 1.623731701744046241, 25.43444280220171194, 13.00000000000000178 ) ) ;
#8176=EDGE_LOOP ( 'NONE', ( #17345, #7124 ) ) ;
#8181=CARTESIAN_POINT ( 'NONE',  ( -3.458872323573595864, 26.51478363815348160, 6.000000000000000000 ) ) ;
#8183=EDGE_LOOP ( 'NONE', ( #26587, #4815, #12559, #31094 ) ) ;
#8190=DIRECTION ( 'NONE',  ( 0.000000000000000000, 0.000000000000000000, 1.000000000000000000 ) ) ;
#8191=EDGE_LOOP ( 'NONE', ( #4468, #34993, #2724, #28577 ) ) ;
#8200=AXIS2_PLACEMENT_3D ( 'NONE', #37412, #37618, #12823 ) ;
#8214=DIRECTION ( 'NONE',  ( 1.000000000000000000, 0.000000000000000000, 0.000000000000000000 ) ) ;
#8218=DIRECTION ( 'NONE',  ( 1.000000000000000000, 0.000000000000000000, 0.000000000000000000 ) ) ;
#8235=EDGE_LOOP ( 'NONE', ( #12441, #18947 ) ) ;
#8244=ORIENTED_EDGE ( 'NONE', *, *, #24642, .F. ) ;
#8263=VECTOR ( 'NONE', #32000, 1000.000000000000000 ) ;
#8271=DIRECTION ( 'NONE',  ( 0.000000000000000000, 0.000000000000000000, 1.000000000000000000 ) ) ;
#8274=CARTESIAN_POINT ( 'NONE',  ( 3.118671991557230516, 37.17221401100731981, 13.00000000000000178 ) ) ;
#8277=ORIENTED_EDGE ( 'NONE', *, *, #2242, .T. ) ;
#8279=DIRECTION ( 'NONE',  ( 1.000000000000000000, 0.000000000000000000, 0.000000000000000000 ) ) ;
#8294=CARTESIAN_POINT ( 'NONE',  ( 6.330070799514983193, 27.28854476845134513, 6.000000000000000000 ) ) ;
#8303=CARTESIAN_POINT ( 'NONE',  ( -11.14717575287011542, 32.53695909538323860, 12.00000000000000000 ) ) ;
#8306=FACE_OUTER_BOUND ( 'NONE', #3245, .T. ) ;
#8312=ORIENTED_EDGE ( 'NONE', *, *, #13832, .F. ) ;
#8315=DIRECTION ( 'NONE',  ( 0.000000000000000000, 0.000000000000000000, 1.000000000000000000 ) ) ;
#8316=ORIENTED_EDGE ( 'NONE', *, *, #22087, .T. ) ;
#8317=DIRECTION ( 'NONE',  ( 0.000000000000000000, 0.000000000000000000, 1.000000000000000000 ) ) ;
#8320=AXIS2_PLACEMENT_3D ( 'NONE', #20197, #4752, #27880 ) ;
#8321=DIRECTION ( 'NONE',  ( 0.000000000000000000, 0.000000000000000000, 1.000000000000000000 ) ) ;
#8323=DIRECTION ( 'NONE',  ( 0.000000000000000000, 0.000000000000000000, 1.000000000000000000 ) ) ;
#8336=FACE_OUTER_BOUND ( 'NONE', #3458, .T. ) ;
#8343=ORIENTED_EDGE ( 'NONE', *, *, #20256, .F. ) ;
#8348=VECTOR ( 'NONE', #32056, 1000.000000000000000 ) ;
#8355=EDGE_CURVE ( 'NONE', #2590, #29319, #26168, .T. ) ;
#8357=ORIENTED_EDGE ( 'NONE', *, *, #19332, .T. ) ;
#8363=ORIENTED_EDGE ( 'NONE', *, *, #17331, .T. ) ;
#8366=DIRECTION ( 'NONE',  ( 0.000000000000000000, 0.000000000000000000, 1.000000000000000000 ) ) ;
#8368=DIRECTION ( 'NONE',  ( 0.000000000000000000, 0.000000000000000000, 1.000000000000000000 ) ) ;
#8369=ORIENTED_EDGE ( 'NONE', *, *, #28043, .F. ) ;
#8370=CARTESIAN_POINT ( 'NONE',  ( -3.476907992048017260, 18.63850621467409496, 6.000000000000000000 ) ) ;
#8380=DIRECTION ( 'NONE',  ( 1.000000000000000000, 0.000000000000000000, 0.000000000000000000 ) ) ;
#8381=CIRCLE ( 'NONE', #7055, 1.000000000000000000 ) ;
#8382=FACE_OUTER_BOUND ( 'NONE', #9118, .T. ) ;
#8384=ORIENTED_EDGE ( 'NONE', *, *, #16329, .F. ) ;
#8396=FACE_OUTER_BOUND ( 'NONE', #33033, .T. ) ;
#8398=CARTESIAN_POINT ( 'NONE',  ( 8.577540944421576441, 33.15743037285414374, 12.00000000000000000 ) ) ;
#8406=CARTESIAN_POINT ( 'NONE',  ( -6.330077540933487512, 17.71145523154927659, 6.000000000000000000 ) ) ;
#8408=VERTEX_POINT ( 'NONE', #34309 ) ;
#8411=ORIENTED_EDGE ( 'NONE', *, *, #36100, .T. ) ;
#8415=ORIENTED_EDGE ( 'NONE', *, *, #1529, .T. ) ;
#8419=CARTESIAN_POINT ( 'NONE',  ( -0.2655091840902661926, 8.754836972118123839, 6.000000000000000000 ) ) ;
#8423=EDGE_CURVE ( 'NONE', #19485, #10298, #9921, .T. ) ;
#8427=FACE_OUTER_BOUND ( 'NONE', #23439, .T. ) ;
#8430=DIRECTION ( 'NONE',  ( 0.000000000000000000, 0.000000000000000000, 1.000000000000000000 ) ) ;
#8434=AXIS2_PLACEMENT_3D ( 'NONE', #15711, #27903, #18767 ) ;
#8443=ORIENTED_EDGE ( 'NONE', *, *, #37334, .F. ) ;
#8452=EDGE_LOOP ( 'NONE', ( #24578, #37470 ) ) ;
#8454=CARTESIAN_POINT ( 'NONE',  ( -3.724378136954612284, 12.76962061027129458, 12.00000000000000000 ) ) ;
#8455=CYLINDRICAL_SURFACE ( 'NONE', #19915, 1.000000000000000888 ) ;
#8457=EDGE_LOOP ( 'NONE', ( #8343, #33467, #35337, #17984 ) ) ;
#8470=EDGE_LOOP ( 'NONE', ( #35385, #21278, #37935, #8363 ) ) ;
#8473=DIRECTION ( 'NONE',  ( 1.000000000000000000, 0.000000000000000000, 0.000000000000000000 ) ) ;
#8475=DIRECTION ( 'NONE',  ( 0.000000000000000000, 0.000000000000000000, 1.000000000000000000 ) ) ;
#8481=VECTOR ( 'NONE', #13146, 1000.000000000000000 ) ;
#8483=DIRECTION ( 'NONE',  ( 0.000000000000000000, 0.000000000000000000, 1.000000000000000000 ) ) ;
#8490=CARTESIAN_POINT ( 'NONE',  ( 2.587660364795204782, 9.681887955242936883, 13.00000000000000178 ) ) ;
#8495=DIRECTION ( 'NONE',  ( 0.000000000000000000, 0.000000000000000000, 1.000000000000000000 ) ) ;
#8497=CIRCLE ( 'NONE', #31194, 1.000000000000000000 ) ;
#8501=VERTEX_POINT ( 'NONE', #31851 ) ;
#8502=CYLINDRICAL_SURFACE ( 'NONE', #1776, 1.000000000000000888 ) ;
#8508=EDGE_CURVE ( 'NONE', #24105, #26292, #36588, .T. ) ;
#8542=CARTESIAN_POINT ( 'NONE',  ( 12.39463915635820612, 18.33192650902018883, 6.000000000000000000 ) ) ;
#8552=EDGE_CURVE ( 'NONE', #33546, #16724, #39148, .T. ) ;
#8559=DIRECTION ( 'NONE',  ( 1.224646799147353207E-16, 1.000000000000000000, -0.000000000000000000 ) ) ;
#8562=DIRECTION ( 'NONE',  ( 1.000000000000000000, 0.000000000000000000, 0.000000000000000000 ) ) ;
#8567=DIRECTION ( 'NONE',  ( 0.000000000000000000, 0.000000000000000000, 1.000000000000000000 ) ) ;
#8569=CIRCLE ( 'NONE', #5990, 1.000000000000000000 ) ;
#8570=ADVANCED_FACE ( 'NONE', ( #32672 ), #29810, .F. ) ;
#8581=CIRCLE ( 'NONE', #808, 1.000000000000000000 ) ;
#8591=ORIENTED_EDGE ( 'NONE', *, *, #38128, .F. ) ;
#8593=UNCERTAINTY_MEASURE_WITH_UNIT (LENGTH_MEASURE( 1.000000000000000082E-05 ), #11767, 'distance_accuracy_value', 'NONE');
#8595=CIRCLE ( 'NONE', #26747, 1.000000000000000888 ) ;
#8601=DIRECTION ( 'NONE',  ( 1.000000000000000000, 0.000000000000000000, 0.000000000000000000 ) ) ;
#8604=EDGE_CURVE ( 'NONE', #31324, #15244, #27475, .T. ) ;
#8608=ORIENTED_EDGE ( 'NONE', *, *, #32251, .T. ) ;
#8610=EDGE_CURVE ( 'NONE', #22293, #19810, #22302, .T. ) ;
#8615=AXIS2_PLACEMENT_3D ( 'NONE', #18741, #18542, #39671 ) ;
#8616=CARTESIAN_POINT ( 'NONE',  ( 3.835130509701798918, 15.55077355964573904, 12.00000000000000000 ) ) ;
#8620=FACE_OUTER_BOUND ( 'NONE', #22417, .T. ) ;
#8635=DIRECTION ( 'NONE',  ( 1.000000000000000000, 0.000000000000000000, 0.000000000000000000 ) ) ;
#8637=ORIENTED_EDGE ( 'NONE', *, *, #18062, .F. ) ;
#8652=FACE_OUTER_BOUND ( 'NONE', #308, .T. ) ;
#8654=ORIENTED_EDGE ( 'NONE', *, *, #7559, .F. ) ;
#8661=EDGE_CURVE ( 'NONE', #12475, #9569, #3489, .T. ) ;
#8665=EDGE_CURVE ( 'NONE', #5003, #4736, #23599, .T. ) ;
#8669=AXIS2_PLACEMENT_3D ( 'NONE', #6453, #19051, #7046 ) ;
#8670=DIRECTION ( 'NONE',  ( 1.000000000000000000, 0.000000000000000000, 0.000000000000000000 ) ) ;
#8671=VERTEX_POINT ( 'NONE', #20271 ) ;
#8675=CARTESIAN_POINT ( 'NONE',  ( -14.01838097023000707, 23.73363068877903359, 12.00000000000000000 ) ) ;
#8677=DIRECTION ( 'NONE',  ( 1.000000000000000000, 0.000000000000000000, 0.000000000000000000 ) ) ;
#8678=DIRECTION ( 'NONE',  ( 1.000000000000000000, 0.000000000000000000, 0.000000000000000000 ) ) ;
#8680=EDGE_CURVE ( 'NONE', #16522, #24243, #14510, .T. ) ;
#8685=DIRECTION ( 'NONE',  ( 0.000000000000000000, 0.000000000000000000, 1.000000000000000000 ) ) ;
#8687=CARTESIAN_POINT ( 'NONE',  ( -9.183247089818959097, 16.78440424842446532, 12.00000000000000000 ) ) ;
#8705=EDGE_CURVE ( 'NONE', #1690, #12341, #37222, .T. ) ;
#8711=AXIS2_PLACEMENT_3D ( 'NONE', #18866, #33371, #30313 ) ;
#8713=DIRECTION ( 'NONE',  ( 1.000000000000000000, 0.000000000000000000, 0.000000000000000000 ) ) ;
#8734=DIRECTION ( 'NONE',  ( 0.000000000000000000, 0.000000000000000000, 1.000000000000000000 ) ) ;
#8743=EDGE_LOOP ( 'NONE', ( #32696, #15311 ) ) ;
#8747=VECTOR ( 'NONE', #20529, 1000.000000000000000 ) ;
#8752=DIRECTION ( 'NONE',  ( 0.000000000000000000, 0.000000000000000000, 1.000000000000000000 ) ) ;
#8754=VECTOR ( 'NONE', #7618, 1000.000000000000000 ) ;
#8767=EDGE_LOOP ( 'NONE', ( #212, #35777 ) ) ;
#8769=CARTESIAN_POINT ( 'NONE',  ( 6.312035131040564906, 19.41226734497195849, 12.00000000000000000 ) ) ;
#8782=ORIENTED_EDGE ( 'NONE', *, *, #14308, .F. ) ;
#8785=AXIS2_PLACEMENT_3D ( 'NONE', #36978, #6483, #6087 ) ;
#8789=DIRECTION ( 'NONE',  ( 0.000000000000000000, 0.000000000000000000, 1.000000000000000000 ) ) ;
#8794=ORIENTED_EDGE ( 'NONE', *, *, #13451, .F. ) ;
#8799=EDGE_LOOP ( 'NONE', ( #3690, #16153, #13797, #17464 ) ) ;
#8805=DIRECTION ( 'NONE',  ( 0.000000000000000000, 0.000000000000000000, 1.000000000000000000 ) ) ;
#8807=ORIENTED_EDGE ( 'NONE', *, *, #25637, .F. ) ;
#8821=FACE_BOUND ( 'NONE', #9879, .T. ) ;
#8822=DIRECTION ( 'NONE',  ( 0.000000000000000000, 0.000000000000000000, 1.000000000000000000 ) ) ;
#8823=ORIENTED_EDGE ( 'NONE', *, *, #19192, .T. ) ;
#8827=FACE_OUTER_BOUND ( 'NONE', #33325, .T. ) ;
#8836=DIRECTION ( 'NONE',  ( 1.000000000000000000, 0.000000000000000000, 0.000000000000000000 ) ) ;
#8839=CYLINDRICAL_SURFACE ( 'NONE', #36535, 1.000000000000000000 ) ;
#8854=LINE ( 'NONE', #39723, #10219 ) ;
#8857=VERTEX_POINT ( 'NONE', #6801 ) ;
#8863=EDGE_CURVE ( 'NONE', #37261, #5543, #13196, .T. ) ;
#8864=CARTESIAN_POINT ( 'NONE',  ( 12.03640989728592459, 29.14264673470096767, 13.00000000000000178 ) ) ;
#8865=EDGE_LOOP ( 'NONE', ( #18999, #10452, #7093, #7037 ) ) ;
#8866=DIRECTION ( 'NONE',  ( 0.000000000000000000, 0.000000000000000000, 1.000000000000000000 ) ) ;
#8867=AXIS2_PLACEMENT_3D ( 'NONE', #38058, #37856, #13269 ) ;
#8868=CARTESIAN_POINT ( 'NONE',  ( -10.77091082532341204, 29.60251629318183575, 12.00000000000000000 ) ) ;
#8869=CARTESIAN_POINT ( 'NONE',  ( -6.082607396026893376, 23.58034083595207875, 13.00000000000000178 ) ) ;
#8876=ADVANCED_FACE ( 'NONE', ( #6412 ), #16926, .F. ) ;
#8880=EDGE_LOOP ( 'NONE', ( #3182, #1833, #5250, #22618 ) ) ;
#8892=EDGE_CURVE ( 'NONE', #25752, #10001, #31421, .T. ) ;
#8901=CIRCLE ( 'NONE', #19266, 16.00000000000000000 ) ;
#8913=CIRCLE ( 'NONE', #36799, 1.000000000000000000 ) ;
#8917=CARTESIAN_POINT ( 'NONE',  ( -5.082607396026893376, 23.58034083595207875, 12.00000000000000000 ) ) ;
#8943=EDGE_LOOP ( 'NONE', ( #18200, #23996 ) ) ;
#8946=FACE_OUTER_BOUND ( 'NONE', #10028, .T. ) ;
#8951=CYLINDRICAL_SURFACE ( 'NONE', #10921, 1.000000000000000000 ) ;
#8956=CARTESIAN_POINT ( 'NONE',  ( -6.330077540933487512, 17.71145523154927659, 6.000000000000000000 ) ) ;
#8960=VECTOR ( 'NONE', #24090, 1000.000000000000000 ) ;
#8963=EDGE_CURVE ( 'NONE', #26936, #35634, #38653, .T. ) ;
#8973=DIRECTION ( 'NONE',  ( 1.000000000000000000, 0.000000000000000000, 0.000000000000000000 ) ) ;
#8975=CARTESIAN_POINT ( 'NONE',  ( 0.7344908159097338629, 8.754836972118123839, 12.00000000000000000 ) ) ;
#8979=CARTESIAN_POINT ( 'NONE',  ( -12.03641663870442713, 15.85735326529964873, 6.000000000000000000 ) ) ;
#8981=EDGE_LOOP ( 'NONE', ( #37968, #25711 ) ) ;
#8986=DIRECTION ( 'NONE',  ( 0.000000000000000000, 0.000000000000000000, 1.000000000000000000 ) ) ;
#8991=CYLINDRICAL_SURFACE ( 'NONE', #23802, 1.000000000000000000 ) ;
#8993=DIRECTION ( 'NONE',  ( 0.000000000000000000, 0.000000000000000000, 1.000000000000000000 ) ) ;
#8995=ORIENTED_EDGE ( 'NONE', *, *, #14619, .T. ) ;
#9008=EDGE_CURVE ( 'NONE', #3338, #19810, #24908, .T. ) ;
#9015=EDGE_CURVE ( 'NONE', #38676, #2411, #34261, .T. ) ;
#9016=CARTESIAN_POINT ( 'NONE',  ( 10.77090408390491127, 15.39748370681878775, 6.000000000000000000 ) ) ;
#9018=VECTOR ( 'NONE', #7557, 1000.000000000000000 ) ;
#9020=FACE_BOUND ( 'NONE', #26337, .T. ) ;
#9027=DIRECTION ( 'NONE',  ( 1.000000000000000000, 0.000000000000000000, 0.000000000000000000 ) ) ;
#9034=EDGE_CURVE ( 'NONE', #10554, #25424, #37878, .T. ) ;
#9035=CARTESIAN_POINT ( 'NONE',  ( -2.835137251120299684, 29.44922644035488446, 12.00000000000000000 ) ) ;
#9038=CARTESIAN_POINT ( 'NONE',  ( -1.605702774688126722, 27.44183462127829642, 6.000000000000000000 ) ) ;
#9039=EDGE_LOOP ( 'NONE', ( #1634, #25978 ) ) ;
#9044=CIRCLE ( 'NONE', #31743, 1.000000000000000000 ) ;
#9053=CARTESIAN_POINT ( 'NONE',  ( -5.082607396026893376, 23.58034083595207875, 13.00000000000000178 ) ) ;
#9059=CARTESIAN_POINT ( 'NONE',  ( -10.16521142134453548, 24.66068167190384841, 13.00000000000000178 ) ) ;
#9066=DIRECTION ( 'NONE',  ( 0.000000000000000000, 0.000000000000000000, 1.000000000000000000 ) ) ;
#9069=DIRECTION ( 'NONE',  ( 1.000000000000000000, 0.000000000000000000, 0.000000000000000000 ) ) ;
#9076=CYLINDRICAL_SURFACE ( 'NONE', #30695, 1.000000000000000888 ) ;
#9079=DIRECTION ( 'NONE',  ( 1.000000000000000000, 0.000000000000000000, 0.000000000000000000 ) ) ;
#9082=DIRECTION ( 'NONE',  ( 1.000000000000000000, 0.000000000000000000, 0.000000000000000000 ) ) ;
#9083=LINE ( 'NONE', #21468, #26355 ) ;
#9085=EDGE_CURVE ( 'NONE', #37515, #4328, #39849, .T. ) ;
#9090=DIRECTION ( 'NONE',  ( 0.000000000000000000, 0.000000000000000000, 1.000000000000000000 ) ) ;
#9099=EDGE_LOOP ( 'NONE', ( #30483, #7131 ) ) ;
#9102=ORIENTED_EDGE ( 'NONE', *, *, #21885, .F. ) ;
#9103=DIRECTION ( 'NONE',  ( 1.000000000000000000, 0.000000000000000000, 0.000000000000000000 ) ) ;
#9117=LINE ( 'NONE', #18662, #632 ) ;
#9118=EDGE_LOOP ( 'NONE', ( #5289, #31981, #22, #34575 ) ) ;
#9130=DIRECTION ( 'NONE',  ( 0.000000000000000000, 0.000000000000000000, 1.000000000000000000 ) ) ;
#9132=EDGE_CURVE ( 'NONE', #36141, #19767, #34669, .T. ) ;
#9140=VERTEX_POINT ( 'NONE', #4929 ) ;
#9145=CARTESIAN_POINT ( 'NONE',  ( 0.6056960332696259552, 17.55816537872232530, 6.000000000000000000 ) ) ;
#9154=EDGE_CURVE ( 'NONE', #36335, #7574, #912, .T. ) ;
#9159=ORIENTED_EDGE ( 'NONE', *, *, #35436, .T. ) ;
#9163=CYLINDRICAL_SURFACE ( 'NONE', #31243, 1.000000000000000888 ) ;
#9165=CARTESIAN_POINT ( 'NONE',  ( -14.26585111513660031, 17.86474508437623143, 13.00000000000000178 ) ) ;
#9184=AXIS2_PLACEMENT_3D ( 'NONE', #12786, #31875, #19087 ) ;
#9198=DIRECTION ( 'NONE',  ( 0.000000000000000000, 0.000000000000000000, 1.000000000000000000 ) ) ;
#9208=EDGE_CURVE ( 'NONE', #26791, #30382, #21050, .T. ) ;
#9216=FACE_BOUND ( 'NONE', #34566, .T. ) ;
#9221=CARTESIAN_POINT ( 'NONE',  ( 0.6417673702184640838, 33.31072022568110924, 6.000000000000000000 ) ) ;
#9227=AXIS2_PLACEMENT_3D ( 'NONE', #5722, #27660, #27862 ) ;
#9230=CARTESIAN_POINT ( 'NONE',  ( -10.16521142134453548, 24.66068167190384841, 13.00000000000000178 ) ) ;
#9236=CARTESIAN_POINT ( 'NONE',  ( -4.706342468480190000, 20.64589803375067945, 6.000000000000000000 ) ) ;
#9247=AXIS2_PLACEMENT_3D ( 'NONE', #19690, #37979, #9950 ) ;
#9249=ADVANCED_FACE ( 'NONE', ( #6118 ), #9579, .F. ) ;
#9262=CARTESIAN_POINT ( 'NONE',  ( 6.688300058587269170, 16.47782454277055564, 13.00000000000000178 ) ) ;
#9264=VECTOR ( 'NONE', #4974, 1000.000000000000000 ) ;
#9280=CARTESIAN_POINT ( 'NONE',  ( 11.41267482483262619, 26.20820393249957192, 13.00000000000000178 ) ) ;
#9287=CARTESIAN_POINT ( 'NONE',  ( -1.247473515615844075, 16.63111439559750693, 13.00000000000000178 ) ) ;
#9293=CIRCLE ( 'NONE', #30055, 1.000000000000000000 ) ;
#9305=EDGE_LOOP ( 'NONE', ( #20390, #27864, #26888, #2883 ) ) ;
#9307=FACE_OUTER_BOUND ( 'NONE', #28594, .T. ) ;
#9310=CIRCLE ( 'NONE', #32005, 1.000000000000000000 ) ;
#9311=EDGE_LOOP ( 'NONE', ( #34775, #17167, #38553, #29028, #33776, #23985, #35306 ) ) ;
#9318=AXIS2_PLACEMENT_3D ( 'NONE', #33228, #1943, #27114 ) ;
#9320=ORIENTED_EDGE ( 'NONE', *, *, #22924, .F. ) ;
#9321=AXIS2_PLACEMENT_3D ( 'NONE', #35044, #19598, #31993 ) ;
#9324=LINE ( 'NONE', #34108, #14396 ) ;
#9330=ORIENTED_EDGE ( 'NONE', *, *, #30869, .F. ) ;
#9335=CARTESIAN_POINT ( 'NONE',  ( -2.587667106213709101, 35.31811204475769728, 12.00000000000000000 ) ) ;
#9346=CARTESIAN_POINT ( 'NONE',  ( -0.2655091840902661926, 8.754836972118123839, 6.000000000000000000 ) ) ;
#9369=CARTESIAN_POINT ( 'NONE',  ( 10.77090408390491127, 15.39748370681878775, 13.00000000000000178 ) ) ;
#9374=DIRECTION ( 'NONE',  ( 1.000000000000000000, 0.000000000000000000, 0.000000000000000000 ) ) ;
#9379=AXIS2_PLACEMENT_3D ( 'NONE', #39998, #39606, #11978 ) ;
#9387=VERTEX_POINT ( 'NONE', #4480 ) ;
#9389=CIRCLE ( 'NONE', #405, 1.000000000000000000 ) ;
#9391=FACE_BOUND ( 'NONE', #24982, .T. ) ;
#9400=DIRECTION ( 'NONE',  ( 1.000000000000000000, 0.000000000000000000, 0.000000000000000000 ) ) ;
#9401=DIRECTION ( 'NONE',  ( 1.000000000000000000, 0.000000000000000000, 0.000000000000000000 ) ) ;
#9410=EDGE_CURVE ( 'NONE', #3673, #21094, #36646, .T. ) ;
#9416=DIRECTION ( 'NONE',  ( 1.000000000000000000, 0.000000000000000000, 0.000000000000000000 ) ) ;
#9418=AXIS2_PLACEMENT_3D ( 'NONE', #40190, #2823, #17682 ) ;
#9421=FACE_OUTER_BOUND ( 'NONE', #8457, .T. ) ;
#9424=DIRECTION ( 'NONE',  ( 0.000000000000000000, 0.000000000000000000, 1.000000000000000000 ) ) ;
#9426=LINE ( 'NONE', #27509, #14420 ) ;
#9450=CARTESIAN_POINT ( 'NONE',  ( -8.917741276437942233, 30.52956727630665057, 12.00000000000000000 ) ) ;
#9452=DIRECTION ( 'NONE',  ( 0.000000000000000000, 0.000000000000000000, 1.000000000000000000 ) ) ;
#9453=AXIS2_PLACEMENT_3D ( 'NONE', #32830, #2347, #23472 ) ;
#9461=EDGE_LOOP ( 'NONE', ( #6938, #26733, #12735, #21537 ) ) ;
#9463=DIRECTION ( 'NONE',  ( 1.000000000000000000, 0.000000000000000000, 0.000000000000000000 ) ) ;
#9468=LINE ( 'NONE', #28145, #9954 ) ;
#9472=CYLINDRICAL_SURFACE ( 'NONE', #22649, 1.000000000000000888 ) ;
#9474=CARTESIAN_POINT ( 'NONE',  ( -1.623738443162547007, 19.56555719779890978, 6.000000000000000000 ) ) ;
#9476=CARTESIAN_POINT ( 'NONE',  ( 2.118671991557230516, 37.17221401100731981, 6.000000000000000000 ) ) ;
#9482=CARTESIAN_POINT ( 'NONE',  ( 13.01837422881150452, 21.26636931122159169, 6.000000000000000000 ) ) ;
#9483=VECTOR ( 'NONE', #10280, 1000.000000000000000 ) ;
#9491=DIRECTION ( 'NONE',  ( 0.000000000000000000, 0.000000000000000000, 1.000000000000000000 ) ) ;
#9514=LINE ( 'NONE', #24945, #7681 ) ;
#9537=CYLINDRICAL_SURFACE ( 'NONE', #27829, 1.000000000000000888 ) ;
#9538=AXIS2_PLACEMENT_3D ( 'NONE', #37478, #40117, #24683 ) ;
#9544=ADVANCED_FACE ( 'NONE', ( #8336 ), #23164, .F. ) ;
#9549=FACE_OUTER_BOUND ( 'NONE', #19529, .T. ) ;
#9551=CARTESIAN_POINT ( 'NONE',  ( -5.082607396026893376, 23.58034083595207875, 13.00000000000000178 ) ) ;
#9554=LINE ( 'NONE', #12985, #38160 ) ;
#9555=DIRECTION ( 'NONE',  ( 1.000000000000000000, 0.000000000000000000, 0.000000000000000000 ) ) ;
#9556=EDGE_LOOP ( 'NONE', ( #21139, #6770, #30253, #34296 ) ) ;
#9565=EDGE_CURVE ( 'NONE', #12651, #13548, #38583, .T. ) ;
#9567=AXIS2_PLACEMENT_3D ( 'NONE', #8087, #20496, #20699 ) ;
#9568=CARTESIAN_POINT ( 'NONE',  ( 9.183240348400453001, 28.21559575157615996, 6.000000000000000000 ) ) ;
#9569=VERTEX_POINT ( 'NONE', #2244 ) ;
#9570=DIRECTION ( 'NONE',  ( 0.000000000000000000, 0.000000000000000000, 1.000000000000000000 ) ) ;
#9573=CIRCLE ( 'NONE', #36200, 1.000000000000000000 ) ;
#9579=CYLINDRICAL_SURFACE ( 'NONE', #32711, 1.000000000000000000 ) ;
#9585=CYLINDRICAL_SURFACE ( 'NONE', #3639, 1.000000000000000000 ) ;
#9587=ORIENTED_EDGE ( 'NONE', *, *, #9882, .F. ) ;
#9591=FACE_BOUND ( 'NONE', #35840, .T. ) ;
#9594=ORIENTED_EDGE ( 'NONE', *, *, #10139, .T. ) ;
#9602=AXIS2_PLACEMENT_3D ( 'NONE', #35948, #8315, #8713 ) ;
#9607=CIRCLE ( 'NONE', #40073, 1.000000000000000000 ) ;
#9618=FACE_OUTER_BOUND ( 'NONE', #20340, .T. ) ;
#9621=EDGE_CURVE ( 'NONE', #40046, #15493, #29459, .T. ) ;
#9622=FACE_BOUND ( 'NONE', #1815, .T. ) ;
#9631=ORIENTED_EDGE ( 'NONE', *, *, #21441, .F. ) ;
#9639=VERTEX_POINT ( 'NONE', #33129 ) ;
#9642=EDGE_CURVE ( 'NONE', #2072, #13470, #28193, .T. ) ;
#9654=CARTESIAN_POINT ( 'NONE',  ( 0.000000000000000000, 22.50000000000000355, 13.00000000000000178 ) ) ;
#9657=ORIENTED_EDGE ( 'NONE', *, *, #27246, .T. ) ;
#9661=AXIS2_PLACEMENT_3D ( 'NONE', #22501, #34911, #35513 ) ;
#9663=EDGE_LOOP ( 'NONE', ( #38524, #7589 ) ) ;
#9676=CARTESIAN_POINT ( 'NONE',  ( 8.183240348400453001, 28.21559575157615996, 6.000000000000000000 ) ) ;
#9679=CARTESIAN_POINT ( 'NONE',  ( -5.953812613386785912, 14.77701242934787906, 6.000000000000000000 ) ) ;
#9684=EDGE_LOOP ( 'NONE', ( #1207, #28331 ) ) ;
#9703=CARTESIAN_POINT ( 'NONE',  ( 2.476901250629512941, 26.36149378532653031, 6.000000000000000000 ) ) ;
#9707=EDGE_LOOP ( 'NONE', ( #26526, #30380, #26386, #17885 ) ) ;
#9716=ORIENTED_EDGE ( 'NONE', *, *, #26517, .T. ) ;
#9717=DIRECTION ( 'NONE',  ( 1.000000000000000000, 0.000000000000000000, 0.000000000000000000 ) ) ;
#9722=CARTESIAN_POINT ( 'NONE',  ( -12.77091082532341382, 29.60251629318183575, 13.00000000000000178 ) ) ;
#9724=LINE ( 'NONE', #6653, #28611 ) ;
#9725=CARTESIAN_POINT ( 'NONE',  ( -12.39464589777671044, 26.66807349098043289, 6.000000000000000000 ) ) ;
#9728=ORIENTED_EDGE ( 'NONE', *, *, #38799, .T. ) ;
#9735=CARTESIAN_POINT ( 'NONE',  ( -8.312041872459065672, 25.58773265502866678, 12.00000000000000000 ) ) ;
#9747=DIRECTION ( 'NONE',  ( 0.000000000000000000, 0.000000000000000000, 1.000000000000000000 ) ) ;
#9750=ADVANCED_FACE ( 'NONE', ( #17891 ), #30871, .F. ) ;
#9752=CARTESIAN_POINT ( 'NONE',  ( -16.00000000000000000, 22.50000000000000711, 12.00000000000000000 ) ) ;
#9754=EDGE_LOOP ( 'NONE', ( #1603, #1414, #16253, #35134 ) ) ;
#9756=CARTESIAN_POINT ( 'NONE',  ( -2.118678732975735279, 7.827785988993307242, 12.00000000000000000 ) ) ;
#9757=VERTEX_POINT ( 'NONE', #2636 ) ;
#9759=VECTOR ( 'NONE', #11165, 1000.000000000000000 ) ;
#9771=EDGE_CURVE ( 'NONE', #8098, #34344, #15212, .T. ) ;
#9773=CYLINDRICAL_SURFACE ( 'NONE', #39633, 1.000000000000000000 ) ;
#9781=CIRCLE ( 'NONE', #37680, 1.000000000000000000 ) ;
#9784=AXIS2_PLACEMENT_3D ( 'NONE', #10261, #29154, #22642 ) ;
#9791=FACE_BOUND ( 'NONE', #16095, .T. ) ;
#9797=DIRECTION ( 'NONE',  ( 0.000000000000000000, 0.000000000000000000, 1.000000000000000000 ) ) ;
#9798=DIRECTION ( 'NONE',  ( 1.000000000000000000, 0.000000000000000000, 0.000000000000000000 ) ) ;
#9800=ORIENTED_EDGE ( 'NONE', *, *, #22586, .F. ) ;
#9802=ORIENTED_EDGE ( 'NONE', *, *, #6314, .F. ) ;
#9804=CARTESIAN_POINT ( 'NONE',  ( 10.78893975237932956, 23.27376113029817617, 6.000000000000000000 ) ) ;
#9814=CARTESIAN_POINT ( 'NONE',  ( 3.458865582155095986, 18.48521636184714012, 12.00000000000000000 ) ) ;
#9815=EDGE_CURVE ( 'NONE', #17253, #4988, #26897, .T. ) ;
#9816=FACE_BOUND ( 'NONE', #24433, .T. ) ;
#9820=DIRECTION ( 'NONE',  ( 1.000000000000000000, 0.000000000000000000, 0.000000000000000000 ) ) ;
#9831=LINE ( 'NONE', #890, #16674 ) ;
#9833=EDGE_CURVE ( 'NONE', #2411, #37016, #32088, .T. ) ;
#9835=ORIENTED_EDGE ( 'NONE', *, *, #25365, .T. ) ;
#9838=CARTESIAN_POINT ( 'NONE',  ( 10.14716901145161465, 12.46304090461738667, 13.00000000000000178 ) ) ;
#9842=CIRCLE ( 'NONE', #7807, 1.000000000000000888 ) ;
#9847=ORIENTED_EDGE ( 'NONE', *, *, #18062, .T. ) ;
#9855=ORIENTED_EDGE ( 'NONE', *, *, #39775, .F. ) ;
#9858=EDGE_CURVE ( 'NONE', #32934, #16598, #24950, .T. ) ;
#9860=FACE_OUTER_BOUND ( 'NONE', #15537, .T. ) ;
#9862=DIRECTION ( 'NONE',  ( 0.000000000000000000, 0.000000000000000000, 1.000000000000000000 ) ) ;
#9864=DIRECTION ( 'NONE',  ( 1.000000000000000000, 0.000000000000000000, 0.000000000000000000 ) ) ;
#9868=DIRECTION ( 'NONE',  ( 0.000000000000000000, 0.000000000000000000, 1.000000000000000000 ) ) ;
#9879=EDGE_LOOP ( 'NONE', ( #19015, #23541 ) ) ;
#9880=CARTESIAN_POINT ( 'NONE',  ( 0.000000000000000000, 22.50000000000000355, 12.00000000000000000 ) ) ;
#9882=EDGE_CURVE ( 'NONE', #25824, #8022, #7427, .T. ) ;
#9900=CARTESIAN_POINT ( 'NONE',  ( 7.559505275947156377, 25.28115294937476065, 13.00000000000000178 ) ) ;
#9904=AXIS2_PLACEMENT_3D ( 'NONE', #10374, #6168, #15915 ) ;
#9906=ORIENTED_EDGE ( 'NONE', *, *, #13876, .T. ) ;
#9908=ORIENTED_EDGE ( 'NONE', *, *, #36332, .F. ) ;
#9911=EDGE_CURVE ( 'NONE', #2500, #5105, #10690, .T. ) ;
#9913=CIRCLE ( 'NONE', #26119, 1.000000000000000000 ) ;
#9920=DIRECTION ( 'NONE',  ( 0.000000000000000000, 0.000000000000000000, 1.000000000000000000 ) ) ;
#9921=LINE ( 'NONE', #22301, #17781 ) ;
#9924=VERTEX_POINT ( 'NONE', #389 ) ;
#9941=ORIENTED_EDGE ( 'NONE', *, *, #11540, .T. ) ;
#9948=VERTEX_POINT ( 'NONE', #19262 ) ;
#9950=DIRECTION ( 'NONE',  ( 1.000000000000000000, 0.000000000000000000, 0.000000000000000000 ) ) ;
#9952=ORIENTED_EDGE ( 'NONE', *, *, #34721, .T. ) ;
#9954=VECTOR ( 'NONE', #27751, 1000.000000000000000 ) ;
#9961=DIRECTION ( 'NONE',  ( 1.000000000000000000, 0.000000000000000000, 0.000000000000000000 ) ) ;
#9967=CARTESIAN_POINT ( 'NONE',  ( -9.541476348891238857, 27.59512447410525127, 12.00000000000000000 ) ) ;
#9970=AXIS2_PLACEMENT_3D ( 'NONE', #15607, #24948, #3608 ) ;
#9971=EDGE_LOOP ( 'NONE', ( #3286, #4263, #21759, #1641 ) ) ;
#9974=DIRECTION ( 'NONE',  ( 1.000000000000000000, 0.000000000000000000, 0.000000000000000000 ) ) ;
#9975=EDGE_LOOP ( 'NONE', ( #14329, #13582 ) ) ;
#9977=AXIS2_PLACEMENT_3D ( 'NONE', #16157, #15959, #26090 ) ;
#9980=CARTESIAN_POINT ( 'NONE',  ( 1.605696033269625955, 17.55816537872232530, 13.00000000000000178 ) ) ;
#9984=LINE ( 'NONE', #19731, #26931 ) ;
#9988=CYLINDRICAL_SURFACE ( 'NONE', #39751, 1.000000000000000000 ) ;
#9991=CARTESIAN_POINT ( 'NONE',  ( -2.229437847141422679, 24.50739181907689712, 6.000000000000000000 ) ) ;
#9993=EDGE_CURVE ( 'NONE', #22329, #11380, #22113, .T. ) ;
#9998=AXIS2_PLACEMENT_3D ( 'NONE', #11117, #4003, #17015 ) ;
#10001=VERTEX_POINT ( 'NONE', #7264 ) ;
#10011=DIRECTION ( 'NONE',  ( 1.000000000000000000, 0.000000000000000000, -0.000000000000000000 ) ) ;
#10012=EDGE_CURVE ( 'NONE', #29252, #697, #32802, .T. ) ;
#10017=DIRECTION ( 'NONE',  ( 0.000000000000000000, 0.000000000000000000, 1.000000000000000000 ) ) ;
#10027=CARTESIAN_POINT ( 'NONE',  ( 2.587660364795204782, 9.681887955242936883, 6.000000000000000000 ) ) ;
#10028=EDGE_LOOP ( 'NONE', ( #10422, #32834, #19828, #20633 ) ) ;
#10032=DIRECTION ( 'NONE',  ( 0.000000000000000000, 0.000000000000000000, 1.000000000000000000 ) ) ;
#10033=ORIENTED_EDGE ( 'NONE', *, *, #20080, .T. ) ;
#10051=CIRCLE ( 'NONE', #36651, 1.000000000000000000 ) ;
#10053=DIRECTION ( 'NONE',  ( 1.000000000000000000, 0.000000000000000000, 0.000000000000000000 ) ) ;
#10062=CARTESIAN_POINT ( 'NONE',  ( 0.2655024426717602637, 36.24516302788250499, 6.000000000000000000 ) ) ;
#10076=DIRECTION ( 'NONE',  ( 0.000000000000000000, 0.000000000000000000, 1.000000000000000000 ) ) ;
#10080=ORIENTED_EDGE ( 'NONE', *, *, #20930, .F. ) ;
#10099=CYLINDRICAL_SURFACE ( 'NONE', #22603, 1.000000000000000888 ) ;
#10103=ORIENTED_EDGE ( 'NONE', *, *, #18716, .F. ) ;
#10106=AXIS2_PLACEMENT_3D ( 'NONE', #24421, #11641, #40 ) ;
#10107=CARTESIAN_POINT ( 'NONE',  ( 0.6056960332696259552, 17.55816537872232530, 13.00000000000000178 ) ) ;
#10129=CARTESIAN_POINT ( 'NONE',  ( -11.14717575287011542, 32.53695909538323860, 13.00000000000000178 ) ) ;
#10139=EDGE_CURVE ( 'NONE', #22765, #19611, #21101, .T. ) ;
#10142=CIRCLE ( 'NONE', #39976, 1.000000000000000000 ) ;
#10143=EDGE_CURVE ( 'NONE', #32505, #33425, #4880, .T. ) ;
#10147=ORIENTED_EDGE ( 'NONE', *, *, #26670, .T. ) ;
#10175=ORIENTED_EDGE ( 'NONE', *, *, #12408, .F. ) ;
#10178=DIRECTION ( 'NONE',  ( 1.000000000000000000, 0.000000000000000000, 0.000000000000000000 ) ) ;
#10185=EDGE_LOOP ( 'NONE', ( #2026, #21465 ) ) ;
#10191=VERTEX_POINT ( 'NONE', #4834 ) ;
#10193=DIRECTION ( 'NONE',  ( 1.000000000000000000, 0.000000000000000000, 0.000000000000000000 ) ) ;
#10198=VERTEX_POINT ( 'NONE', #5237 ) ;
#10200=AXIS2_PLACEMENT_3D ( 'NONE', #36131, #14991, #27378 ) ;
#10208=CYLINDRICAL_SURFACE ( 'NONE', #35611, 1.000000000000000000 ) ;
#10209=CARTESIAN_POINT ( 'NONE',  ( -5.440836655099179353, 34.39106106163288246, 6.000000000000000000 ) ) ;
#10210=FACE_BOUND ( 'NONE', #30267, .T. ) ;
#10217=EDGE_LOOP ( 'NONE', ( #9330, #25774, #2520, #14074, #36247, #16003 ) ) ;
#10219=VECTOR ( 'NONE', #29982, 1000.000000000000000 ) ;
#10221=DIRECTION ( 'NONE',  ( 1.000000000000000000, 0.000000000000000000, 0.000000000000000000 ) ) ;
#10225=CARTESIAN_POINT ( 'NONE',  ( 8.293999462566144842, 11.53598992149257008, 6.000000000000000000 ) ) ;
#10241=CARTESIAN_POINT ( 'NONE',  ( 0.9819609608163288872, 14.62372257652092422, 6.000000000000000000 ) ) ;
#10242=ORIENTED_EDGE ( 'NONE', *, *, #20795, .F. ) ;
#10255=AXIS2_PLACEMENT_3D ( 'NONE', #24780, #12789, #18695 ) ;
#10257=DIRECTION ( 'NONE',  ( 1.000000000000000000, 0.000000000000000000, 0.000000000000000000 ) ) ;
#10260=EDGE_CURVE ( 'NONE', #24757, #27796, #30182, .T. ) ;
#10261=CARTESIAN_POINT ( 'NONE',  ( 12.39463915635820612, 18.33192650902018883, 6.000000000000000000 ) ) ;
#10271=CARTESIAN_POINT ( 'NONE',  ( 0.000000000000000000, 22.50000000000000355, 6.000000000000000000 ) ) ;
#10280=DIRECTION ( 'NONE',  ( 0.000000000000000000, 0.000000000000000000, 1.000000000000000000 ) ) ;
#10287=ORIENTED_EDGE ( 'NONE', *, *, #14868, .T. ) ;
#10292=CIRCLE ( 'NONE', #26503, 1.000000000000000888 ) ;
#10295=EDGE_CURVE ( 'NONE', #5543, #5069, #13976, .T. ) ;
#10298=VERTEX_POINT ( 'NONE', #38760 ) ;
#10306=CARTESIAN_POINT ( 'NONE',  ( -12.14717575287011719, 32.53695909538323860, 6.000000000000000000 ) ) ;
#10309=CARTESIAN_POINT ( 'NONE',  ( 18.00000000000000000, 22.50000000000000711, 13.00000000000000178 ) ) ;
#10310=ORIENTED_EDGE ( 'NONE', *, *, #7349, .F. ) ;
#10317=LINE ( 'NONE', #13154, #37243 ) ;
#10318=DIRECTION ( 'NONE',  ( 1.000000000000000000, 0.000000000000000000, 0.000000000000000000 ) ) ;
#10324=DIRECTION ( 'NONE',  ( 0.000000000000000000, 0.000000000000000000, 1.000000000000000000 ) ) ;
#10341=CIRCLE ( 'NONE', #33067, 1.000000000000000000 ) ;
#10349=AXIS2_PLACEMENT_3D ( 'NONE', #9568, #37788, #9961 ) ;
#10351=ORIENTED_EDGE ( 'NONE', *, *, #10476, .F. ) ;
#10354=ORIENTED_EDGE ( 'NONE', *, *, #34499, .T. ) ;
#10357=VERTEX_POINT ( 'NONE', #2787 ) ;
#10362=FACE_OUTER_BOUND ( 'NONE', #8191, .T. ) ;
#10365=DIRECTION ( 'NONE',  ( 1.000000000000000000, 0.000000000000000000, 0.000000000000000000 ) ) ;
#10368=CARTESIAN_POINT ( 'NONE',  ( -9.183247089818959097, 16.78440424842446532, 6.000000000000000000 ) ) ;
#10372=VECTOR ( 'NONE', #9424, 1000.000000000000000 ) ;
#10373=ORIENTED_EDGE ( 'NONE', *, *, #29443, .T. ) ;
#10374=CARTESIAN_POINT ( 'NONE',  ( -4.724378136954611840, 12.76962061027129458, 6.000000000000000000 ) ) ;
#10387=DIRECTION ( 'NONE',  ( 1.000000000000000000, 0.000000000000000000, 0.000000000000000000 ) ) ;
#10388=EDGE_CURVE ( 'NONE', #19790, #28635, #36008, .T. ) ;
#10389=DIRECTION ( 'NONE',  ( 1.000000000000000000, 0.000000000000000000, 0.000000000000000000 ) ) ;
#10390=EDGE_CURVE ( 'NONE', #37016, #2411, #3571, .T. ) ;
#10397=DIRECTION ( 'NONE',  ( 1.000000000000000000, 0.000000000000000000, 0.000000000000000000 ) ) ;
#10407=EDGE_LOOP ( 'NONE', ( #25265, #39680, #30251, #9941 ) ) ;
#10413=EDGE_CURVE ( 'NONE', #25213, #19790, #37813, .T. ) ;
#10414=FACE_BOUND ( 'NONE', #11853, .T. ) ;
#10416=CIRCLE ( 'NONE', #35075, 1.000000000000000000 ) ;
#10422=ORIENTED_EDGE ( 'NONE', *, *, #2271, .F. ) ;
#10425=FACE_OUTER_BOUND ( 'NONE', #17393, .T. ) ;
#10427=ORIENTED_EDGE ( 'NONE', *, *, #4068, .T. ) ;
#10441=EDGE_LOOP ( 'NONE', ( #18860, #26067 ) ) ;
#10452=ORIENTED_EDGE ( 'NONE', *, *, #4938, .F. ) ;
#10454=DIRECTION ( 'NONE',  ( 0.000000000000000000, 0.000000000000000000, 1.000000000000000000 ) ) ;
#10460=CARTESIAN_POINT ( 'NONE',  ( 2.229431105722923245, 20.49260818092372460, 6.000000000000000000 ) ) ;
#10462=ORIENTED_EDGE ( 'NONE', *, *, #39478, .F. ) ;
#10469=FILL_AREA_STYLE_COLOUR ( '', #7436 ) ;
#10476=EDGE_CURVE ( 'NONE', #5055, #36861, #9984, .T. ) ;
#10481=ORIENTED_EDGE ( 'NONE', *, *, #8665, .F. ) ;
#10492=AXIS2_PLACEMENT_3D ( 'NONE', #20295, #38777, #17256 ) ;
#10495=VERTEX_POINT ( 'NONE', #3684 ) ;
#10510=ORIENTED_EDGE ( 'NONE', *, *, #618, .T. ) ;
#10517=DIRECTION ( 'NONE',  ( 1.000000000000000000, 0.000000000000000000, 0.000000000000000000 ) ) ;
#10542=ORIENTED_EDGE ( 'NONE', *, *, #25872, .T. ) ;
#10548=EDGE_CURVE ( 'NONE', #27371, #15493, #1640, .T. ) ;
#10551=ADVANCED_FACE ( 'NONE', ( #35169 ), #35575, .F. ) ;
#10554=VERTEX_POINT ( 'NONE', #11397 ) ;
#10585=CARTESIAN_POINT ( 'NONE',  ( -0.01803903918367114056, 14.62372257652092422, 13.00000000000000178 ) ) ;
#10591=CARTESIAN_POINT ( 'NONE',  ( 14.01837422881150452, 21.26636931122159169, 6.000000000000000000 ) ) ;
#10608=ORIENTED_EDGE ( 'NONE', *, *, #25798, .T. ) ;
#10616=EDGE_CURVE ( 'NONE', #3736, #17087, #7932, .T. ) ;
#10617=CARTESIAN_POINT ( 'NONE',  ( 4.348106467989403257, 35.16482219193073178, 6.000000000000000000 ) ) ;
#10618=AXIS2_PLACEMENT_3D ( 'NONE', #17973, #6355, #18170 ) ;
#10664=VECTOR ( 'NONE', #38995, 1000.000000000000000 ) ;
#10668=CARTESIAN_POINT ( 'NONE',  ( 9.165204679926031162, 20.33931832809677331, 12.00000000000000000 ) ) ;
#10671=DIRECTION ( 'NONE',  ( 1.000000000000000000, 0.000000000000000000, 0.000000000000000000 ) ) ;
#10676=DIRECTION ( 'NONE',  ( 1.000000000000000000, 0.000000000000000000, 0.000000000000000000 ) ) ;
#10677=ORIENTED_EDGE ( 'NONE', *, *, #33881, .T. ) ;
#10690=CIRCLE ( 'NONE', #13932, 1.000000000000000888 ) ;
#10705=DIRECTION ( 'NONE',  ( 0.000000000000000000, 0.000000000000000000, 1.000000000000000000 ) ) ;
#10707=DIRECTION ( 'NONE',  ( 0.000000000000000000, 0.000000000000000000, 1.000000000000000000 ) ) ;
#10713=AXIS2_PLACEMENT_3D ( 'NONE', #4634, #26164, #2198 ) ;
#10720=DIRECTION ( 'NONE',  ( 0.000000000000000000, 0.000000000000000000, 1.000000000000000000 ) ) ;
#10721=CYLINDRICAL_SURFACE ( 'NONE', #4172, 1.000000000000000888 ) ;
#10722=CARTESIAN_POINT ( 'NONE',  ( -1.247473515615844075, 16.63111439559750693, 13.00000000000000178 ) ) ;
#10724=CARTESIAN_POINT ( 'NONE',  ( 0.000000000000000000, 22.50000000000000355, 13.00000000000000178 ) ) ;
#10730=DIRECTION ( 'NONE',  ( 0.000000000000000000, 0.000000000000000000, 1.000000000000000000 ) ) ;
#10732=DIRECTION ( 'NONE',  ( 0.000000000000000000, 0.000000000000000000, 1.000000000000000000 ) ) ;
#10740=DIRECTION ( 'NONE',  ( 1.000000000000000000, 0.000000000000000000, 0.000000000000000000 ) ) ;
#10748=CARTESIAN_POINT ( 'NONE',  ( 4.118671991557230072, 37.17221401100731981, 12.00000000000000000 ) ) ;
#10751=ORIENTED_EDGE ( 'NONE', *, *, #2717, .T. ) ;
#10759=ORIENTED_EDGE ( 'NONE', *, *, #20330, .F. ) ;
#10766=ORIENTED_EDGE ( 'NONE', *, *, #18060, .F. ) ;
#10767=DIRECTION ( 'NONE',  ( 0.000000000000000000, 0.000000000000000000, 1.000000000000000000 ) ) ;
#10770=DIRECTION ( 'NONE',  ( 1.000000000000000000, 0.000000000000000000, 0.000000000000000000 ) ) ;
#10773=EDGE_LOOP ( 'NONE', ( #25581, #18890, #34965, #24286 ) ) ;
#10775=CARTESIAN_POINT ( 'NONE',  ( 3.494936919103933448, 34.23777120880591696, 13.00000000000000178 ) ) ;
#10780=CIRCLE ( 'NONE', #15327, 1.000000000000000000 ) ;
#10782=VERTEX_POINT ( 'NONE', #38617 ) ;
#10788=AXIS2_PLACEMENT_3D ( 'NONE', #26365, #1590, #38758 ) ;
#10791=ORIENTED_EDGE ( 'NONE', *, *, #26108, .F. ) ;
#10796=CARTESIAN_POINT ( 'NONE',  ( 7.312035131040564906, 19.41226734497195849, 6.000000000000000000 ) ) ;
#10803=ORIENTED_EDGE ( 'NONE', *, *, #31583, .F. ) ;
#10818=VERTEX_POINT ( 'NONE', #18689 ) ;
#10821=DIRECTION ( 'NONE',  ( 0.000000000000000000, 0.000000000000000000, 1.000000000000000000 ) ) ;
#10827=DIRECTION ( 'NONE',  ( 0.000000000000000000, 0.000000000000000000, 1.000000000000000000 ) ) ;
#10828=ORIENTED_EDGE ( 'NONE', *, *, #8705, .T. ) ;
#10833=CARTESIAN_POINT ( 'NONE',  ( -4.100643064501314328, 15.70406341247269211, 12.00000000000000000 ) ) ;
#10837=EDGE_LOOP ( 'NONE', ( #557, #35903, #21776, #18731 ) ) ;
#10843=CIRCLE ( 'NONE', #20568, 1.000000000000000888 ) ;
#10851=DIRECTION ( 'NONE',  ( 0.000000000000000000, 0.000000000000000000, 1.000000000000000000 ) ) ;
#10852=LINE ( 'NONE', #23244, #27081 ) ;
#10858=ADVANCED_FACE ( 'NONE', ( #8946 ), #14840, .F. ) ;
#10861=EDGE_CURVE ( 'NONE', #32505, #32004, #17323, .T. ) ;
#10868=VECTOR ( 'NONE', #32890, 1000.000000000000000 ) ;
#10872=VERTEX_POINT ( 'NONE', #2648 ) ;
#10874=DIRECTION ( 'NONE',  ( 1.000000000000000000, 0.000000000000000000, 0.000000000000000000 ) ) ;
#10879=ADVANCED_FACE ( 'NONE', ( #9549 ), #6482, .F. ) ;
#10881=LINE ( 'NONE', #1531, #28768 ) ;
#10882=EDGE_CURVE ( 'NONE', #37740, #26271, #1772, .T. ) ;
#10884=CIRCLE ( 'NONE', #35532, 1.000000000000000888 ) ;
#10886=ORIENTED_EDGE ( 'NONE', *, *, #36374, .T. ) ;
#10892=EDGE_LOOP ( 'NONE', ( #83, #30543, #39994, #38398 ) ) ;
#10905=CARTESIAN_POINT ( 'NONE',  ( 0.000000000000000000, 22.50000000000000355, 13.00000000000000178 ) ) ;
#10906=DIRECTION ( 'NONE',  ( 0.000000000000000000, 0.000000000000000000, 1.000000000000000000 ) ) ;
#10910=VECTOR ( 'NONE', #206, 1000.000000000000000 ) ;
#10917=AXIS2_PLACEMENT_3D ( 'NONE', #23453, #5558, #32809 ) ;
#10921=AXIS2_PLACEMENT_3D ( 'NONE', #17308, #29682, #1864 ) ;
#10922=EDGE_LOOP ( 'NONE', ( #17116, #8357 ) ) ;
#10923=DIRECTION ( 'NONE',  ( 0.000000000000000000, 0.000000000000000000, 1.000000000000000000 ) ) ;
#10926=ORIENTED_EDGE ( 'NONE', *, *, #20727, .F. ) ;
#10928=CARTESIAN_POINT ( 'NONE',  ( -10.54147634889124063, 27.59512447410525127, 12.00000000000000000 ) ) ;
#10930=CARTESIAN_POINT ( 'NONE',  ( 7.917734535019441466, 14.47043272369397116, 6.000000000000000000 ) ) ;
#10931=DIRECTION ( 'NONE',  ( 1.000000000000000000, 0.000000000000000000, 0.000000000000000000 ) ) ;
#10932=DIRECTION ( 'NONE',  ( 1.000000000000000000, 0.000000000000000000, 0.000000000000000000 ) ) ;
#10933=AXIS2_PLACEMENT_3D ( 'NONE', #17667, #38981, #23544 ) ;
#10943=AXIS2_PLACEMENT_3D ( 'NONE', #29549, #26502, #20415 ) ;
#10954=EDGE_LOOP ( 'NONE', ( #17716, #16368 ) ) ;
#10961=ORIENTED_EDGE ( 'NONE', *, *, #7479, .F. ) ;
#10964=AXIS2_PLACEMENT_3D ( 'NONE', #24250, #5760, #12055 ) ;
#10968=CIRCLE ( 'NONE', #30435, 1.000000000000000888 ) ;
#10969=CARTESIAN_POINT ( 'NONE',  ( -7.935776944912362296, 22.65328985282726393, 12.00000000000000000 ) ) ;
#10974=LINE ( 'NONE', #8112, #956 ) ;
#10975=CYLINDRICAL_SURFACE ( 'NONE', #26691, 1.000000000000000000 ) ;
#10982=ADVANCED_FACE ( 'NONE', ( #20046 ), #14142, .F. ) ;
#10985=CARTESIAN_POINT ( 'NONE',  ( -1.000003370709253492, 22.50000000000031264, 13.00000000000000178 ) ) ;
#10999=DIRECTION ( 'NONE',  ( 0.000000000000000000, 0.000000000000000000, 1.000000000000000000 ) ) ;
#11000=FACE_BOUND ( 'NONE', #5700, .T. ) ;
#11003=EDGE_LOOP ( 'NONE', ( #33057, #36990 ) ) ;
#11005=DIRECTION ( 'NONE',  ( 1.000000000000000000, 0.000000000000000000, 0.000000000000000000 ) ) ;
#11015=ORIENTED_EDGE ( 'NONE', *, *, #24715, .F. ) ;
#11019=CARTESIAN_POINT ( 'NONE',  ( 11.14716901145161643, 12.46304090461738667, 13.00000000000000178 ) ) ;
#11031=DIRECTION ( 'NONE',  ( 1.000000000000000000, 0.000000000000000000, 0.000000000000000000 ) ) ;
#11033=DIRECTION ( 'NONE',  ( 1.000000000000000000, 0.000000000000000000, 0.000000000000000000 ) ) ;
#11034=ADVANCED_FACE ( 'NONE', ( #17001 ), #15838, .F. ) ;
#11040=DIRECTION ( 'NONE',  ( 0.000000000000000000, 0.000000000000000000, 1.000000000000000000 ) ) ;
#11045=ORIENTED_EDGE ( 'NONE', *, *, #35695, .T. ) ;
#11057=DIRECTION ( 'NONE',  ( 1.000000000000000000, 0.000000000000000000, 0.000000000000000000 ) ) ;
#11058=FACE_OUTER_BOUND ( 'NONE', #26880, .T. ) ;
#11059=AXIS2_PLACEMENT_3D ( 'NONE', #1573, #30003, #33269 ) ;
#11067=EDGE_CURVE ( 'NONE', #35978, #21042, #8901, .T. ) ;
#11069=FACE_OUTER_BOUND ( 'NONE', #9305, .T. ) ;
#11070=TOROIDAL_SURFACE ( 'NONE', #25341, 16.00000000000000000, 1.000000000000000000 ) ;
#11072=DIRECTION ( 'NONE',  ( 1.000000000000000000, 0.000000000000000000, 0.000000000000000000 ) ) ;
#11075=EDGE_LOOP ( 'NONE', ( #25737, #16681 ) ) ;
#11078=CYLINDRICAL_SURFACE ( 'NONE', #21395, 1.000000000000000000 ) ;
#11081=CARTESIAN_POINT ( 'NONE',  ( 9.917734535019443243, 14.47043272369397116, 6.000000000000000000 ) ) ;
#11083=EDGE_CURVE ( 'NONE', #37992, #21042, #17982, .T. ) ;
#11089=DIRECTION ( 'NONE',  ( 0.000000000000000000, 0.000000000000000000, 1.000000000000000000 ) ) ;
#11093=VERTEX_POINT ( 'NONE', #18203 ) ;
#11103=CIRCLE ( 'NONE', #22102, 1.000000000000000000 ) ;
#11107=ORIENTED_EDGE ( 'NONE', *, *, #30341, .F. ) ;
#11115=FACE_OUTER_BOUND ( 'NONE', #5079, .T. ) ;
#11116=ORIENTED_EDGE ( 'NONE', *, *, #38589, .T. ) ;
#11117=CARTESIAN_POINT ( 'NONE',  ( 5.348106467989403257, 35.16482219193073178, 6.000000000000000000 ) ) ;
#11118=CIRCLE ( 'NONE', #28652, 1.000000000000000000 ) ;
#11125=CARTESIAN_POINT ( 'NONE',  ( 7.953805871968279817, 30.22298757065274444, 6.000000000000000000 ) ) ;
#11127=CARTESIAN_POINT ( 'NONE',  ( 9.165204679926031162, 20.33931832809677331, 6.000000000000000000 ) ) ;
#11130=EDGE_LOOP ( 'NONE', ( #7367, #20396 ) ) ;
#11133=CARTESIAN_POINT ( 'NONE',  ( 2.229431105722923245, 20.49260818092372460, 12.00000000000000000 ) ) ;
#11134=ADVANCED_FACE ( 'NONE', ( #20854 ), #8455, .F. ) ;
#11141=EDGE_CURVE ( 'NONE', #13470, #5684, #20653, .T. ) ;
#11154=ORIENTED_EDGE ( 'NONE', *, *, #668, .T. ) ;
#11156=EDGE_CURVE ( 'NONE', #333, #10298, #23801, .T. ) ;
#11157=VERTEX_POINT ( 'NONE', #5402 ) ;
#11162=CYLINDRICAL_SURFACE ( 'NONE', #19335, 1.000000000000000000 ) ;
#11165=DIRECTION ( 'NONE',  ( 0.000000000000000000, 0.000000000000000000, 1.000000000000000000 ) ) ;
#11168=ORIENTED_EDGE ( 'NONE', *, *, #29443, .F. ) ;
#11194=FACE_BOUND ( 'NONE', #38576, .T. ) ;
#11197=DIRECTION ( 'NONE',  ( 1.000000000000000000, 0.000000000000000000, 0.000000000000000000 ) ) ;
#11198=ORIENTED_EDGE ( 'NONE', *, *, #39945, .F. ) ;
#11203=ORIENTED_EDGE ( 'NONE', *, *, #14245, .F. ) ;
#11206=FACE_OUTER_BOUND ( 'NONE', #22661, .T. ) ;
#11216=CIRCLE ( 'NONE', #37163, 16.00000000000000000 ) ;
#11226=DIRECTION ( 'NONE',  ( 0.000000000000000000, 0.000000000000000000, 1.000000000000000000 ) ) ;
#11229=VERTEX_POINT ( 'NONE', #39122 ) ;
#11230=CIRCLE ( 'NONE', #843, 1.000000000000000000 ) ;
#11236=LINE ( 'NONE', #8181, #19858 ) ;
#11242=DIRECTION ( 'NONE',  ( 1.000000000000000000, 0.000000000000000000, 0.000000000000000000 ) ) ;
#11244=CARTESIAN_POINT ( 'NONE',  ( 9.293999462566146619, 11.53598992149257008, 13.00000000000000178 ) ) ;
#11246=ORIENTED_EDGE ( 'NONE', *, *, #32881, .F. ) ;
#11249=CARTESIAN_POINT ( 'NONE',  ( 12.14716901145161643, 12.46304090461738667, 6.000000000000000000 ) ) ;
#11253=AXIS2_PLACEMENT_3D ( 'NONE', #9038, #21422, #5977 ) ;
#11261=ORIENTED_EDGE ( 'NONE', *, *, #575, .T. ) ;
#11267=DIRECTION ( 'NONE',  ( 0.000000000000000000, 0.000000000000000000, 1.000000000000000000 ) ) ;
#11268=ADVANCED_FACE ( 'NONE', ( #8652 ), #23688, .F. ) ;
#11278=DIRECTION ( 'NONE',  ( 1.000000000000000000, 0.000000000000000000, 0.000000000000000000 ) ) ;
#11281=DIRECTION ( 'NONE',  ( 1.000000000000000000, 0.000000000000000000, 0.000000000000000000 ) ) ;
#11290=ADVANCED_FACE ( 'NONE', ( #3739 ), #6778, .T. ) ;
#11291=EDGE_CURVE ( 'NONE', #25337, #11380, #12148, .T. ) ;
#11292=CARTESIAN_POINT ( 'NONE',  ( -7.064571727552472424, 31.45661825943146894, 6.000000000000000000 ) ) ;
#11310=ORIENTED_EDGE ( 'NONE', *, *, #7647, .T. ) ;
#11315=DIRECTION ( 'NONE',  ( 1.000000000000000000, 0.000000000000000000, 0.000000000000000000 ) ) ;
#11316=EDGE_CURVE ( 'NONE', #33425, #1690, #11480, .T. ) ;
#11319=AXIS2_PLACEMENT_3D ( 'NONE', #29595, #28993, #35090 ) ;
#11321=CARTESIAN_POINT ( 'NONE',  ( -1.853172919594719970, 21.57294901687549427, 12.00000000000000000 ) ) ;
#11324=AXIS2_PLACEMENT_3D ( 'NONE', #382, #9920, #25155 ) ;
#11340=DIRECTION ( 'NONE',  ( 1.000000000000000000, 0.000000000000000000, 0.000000000000000000 ) ) ;
#11356=LINE ( 'NONE', #30040, #7035 ) ;
#11358=ORIENTED_EDGE ( 'NONE', *, *, #31257, .F. ) ;
#11365=EDGE_LOOP ( 'NONE', ( #30741, #30918, #2060, #29849 ) ) ;
#11372=DIRECTION ( 'NONE',  ( 0.000000000000000000, 0.000000000000000000, 1.000000000000000000 ) ) ;
#11374=SURFACE_STYLE_FILL_AREA ( #5070 ) ;
#11380=VERTEX_POINT ( 'NONE', #5991 ) ;
#11382=FACE_OUTER_BOUND ( 'NONE', #19042, .T. ) ;
#11386=EDGE_CURVE ( 'NONE', #33800, #14056, #27054, .T. ) ;
#11392=DIRECTION ( 'NONE',  ( 0.000000000000000000, 0.000000000000000000, 1.000000000000000000 ) ) ;
#11393=ORIENTED_EDGE ( 'NONE', *, *, #7509, .F. ) ;
#11394=VERTEX_POINT ( 'NONE', #22032 ) ;
#11397=CARTESIAN_POINT ( 'NONE',  ( 13.03640989728592459, 29.14264673470096767, 12.00000000000000000 ) ) ;
#11399=CIRCLE ( 'NONE', #23045, 1.000000000000000888 ) ;
#11403=LINE ( 'NONE', #30085, #20667 ) ;
#11419=DIRECTION ( 'NONE',  ( 1.000000000000000000, 0.000000000000000000, 0.000000000000000000 ) ) ;
#11420=ORIENTED_EDGE ( 'NONE', *, *, #12085, .F. ) ;
#11421=DIRECTION ( 'NONE',  ( 1.000000000000000000, 0.000000000000000000, 0.000000000000000000 ) ) ;
#11423=AXIS2_PLACEMENT_3D ( 'NONE', #10833, #1900, #20180 ) ;
#11424=VECTOR ( 'NONE', #36261, 1000.000000000000000 ) ;
#11435=ORIENTED_EDGE ( 'NONE', *, *, #30665, .T. ) ;
#11447=EDGE_LOOP ( 'NONE', ( #10351, #8443, #25730, #9847 ) ) ;
#11453=CARTESIAN_POINT ( 'NONE',  ( -5.100643064501314328, 15.70406341247269211, 6.000000000000000000 ) ) ;
#11455=VECTOR ( 'NONE', #5482, 1000.000000000000000 ) ;
#11459=CIRCLE ( 'NONE', #19212, 1.000000000000000000 ) ;
#11461=VECTOR ( 'NONE', #33834, 1000.000000000000000 ) ;
#11469=DIRECTION ( 'NONE',  ( 0.000000000000000000, 0.000000000000000000, 1.000000000000000000 ) ) ;
#11477=CARTESIAN_POINT ( 'NONE',  ( 6.577540944421576441, 33.15743037285414374, 6.000000000000000000 ) ) ;
#11480=CIRCLE ( 'NONE', #34189, 16.00000000000000000 ) ;
#11498=DIRECTION ( 'NONE',  ( 1.000000000000000000, 0.000000000000000000, 0.000000000000000000 ) ) ;
#11501=ORIENTED_EDGE ( 'NONE', *, *, #37687, .F. ) ;
#11503=LINE ( 'NONE', #27336, #3093 ) ;
#11504=CARTESIAN_POINT ( 'NONE',  ( 14.26584437371809777, 27.13525491562438319, 6.000000000000000000 ) ) ;
#11510=DIRECTION ( 'NONE',  ( 1.000000000000000000, 0.000000000000000000, 0.000000000000000000 ) ) ;
#11513=DIRECTION ( 'NONE',  ( 0.000000000000000000, 0.000000000000000000, 1.000000000000000000 ) ) ;
#11515=ADVANCED_FACE ( 'NONE', ( #26284 ), #22829, .F. ) ;
#11517=EDGE_CURVE ( 'NONE', #7227, #13219, #10852, .T. ) ;
#11518=FACE_OUTER_BOUND ( 'NONE', #29434, .T. ) ;
#11519=AXIS2_PLACEMENT_3D ( 'NONE', #25885, #1315, #23043 ) ;
#11520=AXIS2_PLACEMENT_3D ( 'NONE', #39549, #8475, #11725 ) ;
#11521=CARTESIAN_POINT ( 'NONE',  ( -8.559512017365658920, 19.71884705062586107, 13.00000000000000178 ) ) ;
#11527=DIRECTION ( 'NONE',  ( 0.000000000000000000, 0.000000000000000000, 1.000000000000000000 ) ) ;
#11528=DIRECTION ( 'NONE',  ( 1.000000000000000000, 0.000000000000000000, 0.000000000000000000 ) ) ;
#11531=DIRECTION ( 'NONE',  ( 1.000000000000000000, 0.000000000000000000, 0.000000000000000000 ) ) ;
#11540=EDGE_CURVE ( 'NONE', #12049, #28113, #17377, .T. ) ;
#11549=ORIENTED_EDGE ( 'NONE', *, *, #11787, .F. ) ;
#11556=DIRECTION ( 'NONE',  ( 0.000000000000000000, 0.000000000000000000, 1.000000000000000000 ) ) ;
#11561=EDGE_LOOP ( 'NONE', ( #1103, #28853, #7859, #13257 ) ) ;
#11567=DIRECTION ( 'NONE',  ( 0.000000000000000000, 0.000000000000000000, 1.000000000000000000 ) ) ;
#11572=CARTESIAN_POINT ( 'NONE',  ( 15.21690391738993320, 27.44427296666788862, 12.00000000000000000 ) ) ;
#11574=CARTESIAN_POINT ( 'NONE',  ( -2.587667106213709101, 35.31811204475769728, 13.00000000000000178 ) ) ;
#11580=DIRECTION ( 'NONE',  ( 0.000000000000000000, 0.000000000000000000, 1.000000000000000000 ) ) ;
#11581=CARTESIAN_POINT ( 'NONE',  ( 3.476901250629512941, 26.36149378532653031, 6.000000000000000000 ) ) ;
#11585=EDGE_CURVE ( 'NONE', #22756, #26036, #27704, .T. ) ;
#11598=AXIS2_PLACEMENT_3D ( 'NONE', #4608, #36300, #35693 ) ;
#11600=ADVANCED_FACE ( 'NONE', ( #23642 ), #33003, .F. ) ;
#11606=AXIS2_PLACEMENT_3D ( 'NONE', #8616, #36448, #31341 ) ;
#11607=ORIENTED_EDGE ( 'NONE', *, *, #32408, .F. ) ;
#11616=ADVANCED_FACE ( 'NONE', ( #11058 ), #33598, .F. ) ;
#11618=EDGE_CURVE ( 'NONE', #19095, #20361, #2313, .T. ) ;
#11620=CARTESIAN_POINT ( 'NONE',  ( -11.14717575287011542, 32.53695909538323860, 13.00000000000000178 ) ) ;
#11621=EDGE_LOOP ( 'NONE', ( #26582, #25860, #7537, #31168 ) ) ;
#11641=DIRECTION ( 'NONE',  ( 0.000000000000000000, 0.000000000000000000, 1.000000000000000000 ) ) ;
#11651=ADVANCED_FACE ( 'NONE', ( #36246 ), #27290, .F. ) ;
#11655=EDGE_LOOP ( 'NONE', ( #36318, #33748 ) ) ;
#11658=CARTESIAN_POINT ( 'NONE',  ( -2.229437847141422679, 24.50739181907689712, 12.00000000000000000 ) ) ;
#11659=EDGE_LOOP ( 'NONE', ( #16653, #3522 ) ) ;
#11668=EDGE_CURVE ( 'NONE', #488, #30103, #31626, .T. ) ;
#11669=CARTESIAN_POINT ( 'NONE',  ( 6.935770203493858865, 22.34671014717335780, 13.00000000000000178 ) ) ;
#11670=CARTESIAN_POINT ( 'NONE',  ( 3.211395437248501850, 12.61633075744433796, 12.00000000000000000 ) ) ;
#11671=FACE_BOUND ( 'NONE', #34035, .T. ) ;
#11673=VERTEX_POINT ( 'NONE', #5547 ) ;
#11678=DIRECTION ( 'NONE',  ( 0.000000000000000000, 0.000000000000000000, 1.000000000000000000 ) ) ;
#11681=CIRCLE ( 'NONE', #39574, 1.000000000000000000 ) ;
#11682=EDGE_LOOP ( 'NONE', ( #33193, #23823, #28220, #18056 ) ) ;
#11695=DIRECTION ( 'NONE',  ( 0.000000000000000000, 0.000000000000000000, 1.000000000000000000 ) ) ;
#11698=DIRECTION ( 'NONE',  ( 0.000000000000000000, 0.000000000000000000, 1.000000000000000000 ) ) ;
#11702=CARTESIAN_POINT ( 'NONE',  ( -9.788946493797832105, 21.72623886970244911, 6.000000000000000000 ) ) ;
#11716=CIRCLE ( 'NONE', #32455, 1.000000000000000000 ) ;
#11725=DIRECTION ( 'NONE',  ( 1.000000000000000000, 0.000000000000000000, 0.000000000000000000 ) ) ;
#11726=CARTESIAN_POINT ( 'NONE',  ( -7.577547685840081648, 11.84256962714647798, 12.00000000000000000 ) ) ;
#11733=CARTESIAN_POINT ( 'NONE',  ( -9.806982162272253944, 13.84996144622306247, 13.00000000000000178 ) ) ;
#11735=VECTOR ( 'NONE', #17022, 1000.000000000000000 ) ;
#11741=CARTESIAN_POINT ( 'NONE',  ( -11.77091082532341204, 29.60251629318183575, 12.00000000000000000 ) ) ;
#11746=DIRECTION ( 'NONE',  ( 1.000000000000000000, 0.000000000000000000, 0.000000000000000000 ) ) ;
#11754=DIRECTION ( 'NONE',  ( 0.000000000000000000, 0.000000000000000000, 1.000000000000000000 ) ) ;
#11764=LINE ( 'NONE', #2623, #37584 ) ;
#11767=( LENGTH_UNIT ( ) NAMED_UNIT ( * ) SI_UNIT ( .MILLI., .METRE. ) );
#11768=CARTESIAN_POINT ( 'NONE',  ( -4.835137251120299240, 29.44922644035488446, 13.00000000000000178 ) ) ;
#11780=CARTESIAN_POINT ( 'NONE',  ( -8.294006203984645609, 33.46401007850805343, 6.000000000000000000 ) ) ;
#11783=AXIS2_PLACEMENT_3D ( 'NONE', #5663, #14621, #30663 ) ;
#11787=EDGE_CURVE ( 'NONE', #36348, #36134, #34882, .T. ) ;
#11789=EDGE_CURVE ( 'NONE', #29252, #9948, #22178, .T. ) ;
#11791=VERTEX_POINT ( 'NONE', #15292 ) ;
#11813=DIRECTION ( 'NONE',  ( 0.000000000000000000, 0.000000000000000000, 1.000000000000000000 ) ) ;
#11832=CARTESIAN_POINT ( 'NONE',  ( 11.16520467992603294, 20.33931832809677331, 6.000000000000000000 ) ) ;
#11834=EDGE_LOOP ( 'NONE', ( #2498, #11420, #30736, #38681 ) ) ;
#11838=CARTESIAN_POINT ( 'NONE',  ( 2.247466774197339756, 28.36888560440311480, 13.00000000000000178 ) ) ;
#11840=CARTESIAN_POINT ( 'NONE',  ( 2.605696033269626177, 17.55816537872232530, 6.000000000000000000 ) ) ;
#11845=CIRCLE ( 'NONE', #35890, 1.000000000000000888 ) ;
#11849=CYLINDRICAL_SURFACE ( 'NONE', #8320, 1.000000000000000000 ) ;
#11853=EDGE_LOOP ( 'NONE', ( #28716, #17661 ) ) ;
#11864=EDGE_CURVE ( 'NONE', #10191, #8118, #3715, .T. ) ;
#11868=CARTESIAN_POINT ( 'NONE',  ( -7.330077540933487512, 17.71145523154927659, 13.00000000000000178 ) ) ;
#11869=ORIENTED_EDGE ( 'NONE', *, *, #1944, .F. ) ;
#11872=DIRECTION ( 'NONE',  ( 1.000000000000000000, 0.000000000000000000, -0.000000000000000000 ) ) ;
#11880=AXIS2_PLACEMENT_3D ( 'NONE', #28446, #622, #13003 ) ;
#11881=CARTESIAN_POINT ( 'NONE',  ( 4.724371395536106633, 32.23037938972932892, 13.00000000000000178 ) ) ;
#11883=EDGE_LOOP ( 'NONE', ( #3306, #18465 ) ) ;
#11887=CARTESIAN_POINT ( 'NONE',  ( -3.476907992048017260, 18.63850621467409496, 13.00000000000000178 ) ) ;
#11891=EDGE_CURVE ( 'NONE', #11229, #17253, #12803, .T. ) ;
#11900=DIRECTION ( 'NONE',  ( 1.000000000000000000, 0.000000000000000000, 0.000000000000000000 ) ) ;
#11901=DIRECTION ( 'NONE',  ( 0.000000000000000000, 0.000000000000000000, 1.000000000000000000 ) ) ;
#11904=CIRCLE ( 'NONE', #20312, 1.000000000000000000 ) ;
#11910=AXIS2_PLACEMENT_3D ( 'NONE', #36559, #23968, #36163 ) ;
#11915=CARTESIAN_POINT ( 'NONE',  ( -10.54147634889124063, 27.59512447410525127, 6.000000000000000000 ) ) ;
#11923=DIRECTION ( 'NONE',  ( 1.000000000000000000, 0.000000000000000000, 0.000000000000000000 ) ) ;
#11931=AXIS2_PLACEMENT_3D ( 'NONE', #28542, #919, #4360 ) ;
#11939=CARTESIAN_POINT ( 'NONE',  ( -5.330077540933487512, 17.71145523154927659, 13.00000000000000178 ) ) ;
#11948=VERTEX_POINT ( 'NONE', #1054 ) ;
#11952=ORIENTED_EDGE ( 'NONE', *, *, #29393, .F. ) ;
#11962=DIRECTION ( 'NONE',  ( 0.000000000000000000, 0.000000000000000000, 1.000000000000000000 ) ) ;
#11964=LINE ( 'NONE', #30659, #28527 ) ;
#11965=ORIENTED_EDGE ( 'NONE', *, *, #19795, .F. ) ;
#11973=CIRCLE ( 'NONE', #19104, 1.000000000000000888 ) ;
#11978=DIRECTION ( 'NONE',  ( 1.000000000000000000, 0.000000000000000000, 0.000000000000000000 ) ) ;
#11989=DIRECTION ( 'NONE',  ( 0.000000000000000000, 0.000000000000000000, 1.000000000000000000 ) ) ;
#12022=DIRECTION ( 'NONE',  ( 1.000000000000000000, 0.000000000000000000, 0.000000000000000000 ) ) ;
#12032=ORIENTED_EDGE ( 'NONE', *, *, #13963, .F. ) ;
#12033=ORIENTED_EDGE ( 'NONE', *, *, #12514, .T. ) ;
#12039=EDGE_LOOP ( 'NONE', ( #22325, #26671 ) ) ;
#12049=VERTEX_POINT ( 'NONE', #22575 ) ;
#12054=AXIS2_PLACEMENT_3D ( 'NONE', #20588, #11040, #23424 ) ;
#12055=DIRECTION ( 'NONE',  ( -1.000000000000000000, 0.000000000000000000, 0.000000000000000000 ) ) ;
#12057=AXIS2_PLACEMENT_3D ( 'NONE', #24318, #18425, #2589 ) ;
#12060=DIRECTION ( 'NONE',  ( 0.000000000000000000, 0.000000000000000000, 1.000000000000000000 ) ) ;
#12062=FACE_BOUND ( 'NONE', #37572, .T. ) ;
#12079=CYLINDRICAL_SURFACE ( 'NONE', #11253, 1.000000000000000000 ) ;
#12085=EDGE_CURVE ( 'NONE', #33602, #13627, #18670, .T. ) ;
#12086=DIRECTION ( 'NONE',  ( 0.000000000000000000, 0.000000000000000000, 1.000000000000000000 ) ) ;
#12096=DIRECTION ( 'NONE',  ( 1.000000000000000000, 0.000000000000000000, 0.000000000000000000 ) ) ;
#12103=EDGE_CURVE ( 'NONE', #8501, #1841, #19326, .T. ) ;
#12109=EDGE_CURVE ( 'NONE', #1553, #30133, #31653, .T. ) ;
#12111=ADVANCED_FACE ( 'NONE', ( #19334 ), #32133, .F. ) ;
#12115=DIRECTION ( 'NONE',  ( 1.000000000000000000, 0.000000000000000000, 0.000000000000000000 ) ) ;
#12118=DIRECTION ( 'NONE',  ( 0.000000000000000000, 0.000000000000000000, 1.000000000000000000 ) ) ;
#12134=VERTEX_POINT ( 'NONE', #19943 ) ;
#12148=CIRCLE ( 'NONE', #15356, 1.000000000000000888 ) ;
#12151=VERTEX_POINT ( 'NONE', #5493 ) ;
#12152=CARTESIAN_POINT ( 'NONE',  ( 2.605696033269626177, 17.55816537872232530, 13.00000000000000178 ) ) ;
#12158=LINE ( 'NONE', #28189, #27807 ) ;
#12162=CARTESIAN_POINT ( 'NONE',  ( -4.100643064501314328, 15.70406341247269211, 6.000000000000000000 ) ) ;
#12163=ORIENTED_EDGE ( 'NONE', *, *, #4437, .F. ) ;
#12172=AXIS2_PLACEMENT_3D ( 'NONE', #33453, #26938, #36291 ) ;
#12173=VERTEX_POINT ( 'NONE', #17511 ) ;
#12175=DIRECTION ( 'NONE',  ( 0.000000000000000000, 0.000000000000000000, 1.000000000000000000 ) ) ;
#12177=DIRECTION ( 'NONE',  ( 1.000000000000000000, 0.000000000000000000, 0.000000000000000000 ) ) ;
#12186=ORIENTED_EDGE ( 'NONE', *, *, #17363, .T. ) ;
#12191=EDGE_LOOP ( 'NONE', ( #6282, #31315 ) ) ;
#12195=AXIS2_PLACEMENT_3D ( 'NONE', #37406, #633, #10178 ) ;
#12199=ORIENTED_EDGE ( 'NONE', *, *, #33261, .F. ) ;
#12201=CIRCLE ( 'NONE', #19972, 1.000000000000000000 ) ;
#12202=AXIS2_PLACEMENT_3D ( 'NONE', #36434, #33199, #11057 ) ;
#12210=CARTESIAN_POINT ( 'NONE',  ( -6.440836655099179353, 34.39106106163288246, 12.00000000000000000 ) ) ;
#12215=CARTESIAN_POINT ( 'NONE',  ( 4.100636323082810009, 29.29593658752792962, 6.000000000000000000 ) ) ;
#12220=EDGE_CURVE ( 'NONE', #4132, #16724, #29045, .T. ) ;
#12222=DIRECTION ( 'NONE',  ( 1.000000000000000000, 0.000000000000000000, 0.000000000000000000 ) ) ;
#12223=DIRECTION ( 'NONE',  ( 0.000000000000000000, 0.000000000000000000, 1.000000000000000000 ) ) ;
#12224=CARTESIAN_POINT ( 'NONE',  ( -2.229437847141422679, 24.50739181907689712, 13.00000000000000178 ) ) ;
#12225=ORIENTED_EDGE ( 'NONE', *, *, #9771, .F. ) ;
#12227=VECTOR ( 'NONE', #20350, 1000.000000000000000 ) ;
#12232=ORIENTED_EDGE ( 'NONE', *, *, #25773, .T. ) ;
#12236=CIRCLE ( 'NONE', #33019, 1.000000000000000888 ) ;
#12258=CIRCLE ( 'NONE', #15511, 1.000000000000000000 ) ;
#12259=CARTESIAN_POINT ( 'NONE',  ( -13.64211604268330724, 20.79918788657763429, 12.00000000000000000 ) ) ;
#12260=DIRECTION ( 'NONE',  ( 0.000000000000000000, 0.000000000000000000, 1.000000000000000000 ) ) ;
#12264=FACE_BOUND ( 'NONE', #37590, .T. ) ;
#12268=CARTESIAN_POINT ( 'NONE',  ( 5.348106467989403257, 35.16482219193073178, 6.000000000000000000 ) ) ;
#12272=CARTESIAN_POINT ( 'NONE',  ( -2.835137251120299684, 29.44922644035488446, 13.00000000000000178 ) ) ;
#12277=DIRECTION ( 'NONE',  ( 0.000000000000000000, 0.000000000000000000, 1.000000000000000000 ) ) ;
#12280=CARTESIAN_POINT ( 'NONE',  ( 2.853166178176219425, 23.42705098312512746, 12.00000000000000000 ) ) ;
#12283=CARTESIAN_POINT ( 'NONE',  ( -2.853172919594720192, 21.57294901687549427, 12.00000000000000000 ) ) ;
#12291=ORIENTED_EDGE ( 'NONE', *, *, #10413, .F. ) ;
#12296=EDGE_CURVE ( 'NONE', #2033, #19314, #23219, .T. ) ;
#12302=DIRECTION ( 'NONE',  ( 0.000000000000000000, 0.000000000000000000, 1.000000000000000000 ) ) ;
#12318=CARTESIAN_POINT ( 'NONE',  ( 6.312035131040564906, 19.41226734497195849, 6.000000000000000000 ) ) ;
#12322=DIRECTION ( 'NONE',  ( 1.000000000000000000, 0.000000000000000000, 0.000000000000000000 ) ) ;
#12331=ORIENTED_EDGE ( 'NONE', *, *, #22945, .F. ) ;
#12332=CARTESIAN_POINT ( 'NONE',  ( 2.853166178176219425, 23.42705098312512746, 6.000000000000000000 ) ) ;
#12341=VERTEX_POINT ( 'NONE', #9752 ) ;
#12347=CARTESIAN_POINT ( 'NONE',  ( 5.064564986133971658, 13.54338174056915456, 12.00000000000000000 ) ) ;
#12352=DIRECTION ( 'NONE',  ( 0.000000000000000000, 0.000000000000000000, 1.000000000000000000 ) ) ;
#12353=ORIENTED_EDGE ( 'NONE', *, *, #11141, .T. ) ;
#12375=AXIS2_PLACEMENT_3D ( 'NONE', #11574, #39596, #23962 ) ;
#12392=FACE_OUTER_BOUND ( 'NONE', #7483, .T. ) ;
#12394=ORIENTED_EDGE ( 'NONE', *, *, #21707, .T. ) ;
#12401=AXIS2_PLACEMENT_3D ( 'NONE', #7056, #13153, #17025 ) ;
#12403=DIRECTION ( 'NONE',  ( 1.000000000000000000, 0.000000000000000000, 0.000000000000000000 ) ) ;
#12408=EDGE_CURVE ( 'NONE', #33298, #12173, #12830, .T. ) ;
#12412=DIRECTION ( 'NONE',  ( 1.000000000000000000, 0.000000000000000000, 0.000000000000000000 ) ) ;
#12416=CIRCLE ( 'NONE', #39590, 1.000000000000000000 ) ;
#12418=DIRECTION ( 'NONE',  ( 0.000000000000000000, 0.000000000000000000, 1.000000000000000000 ) ) ;
#12419=CARTESIAN_POINT ( 'NONE',  ( 11.14716901145161643, 12.46304090461738667, 13.00000000000000178 ) ) ;
#12428=ORIENTED_EDGE ( 'NONE', *, *, #36274, .F. ) ;
#12431=FACE_BOUND ( 'NONE', #8073, .T. ) ;
#12441=ORIENTED_EDGE ( 'NONE', *, *, #26045, .T. ) ;
#12443=ORIENTED_EDGE ( 'NONE', *, *, #37203, .F. ) ;
#12455=CIRCLE ( 'NONE', #19591, 1.000000000000000888 ) ;
#12458=FACE_BOUND ( 'NONE', #5993, .T. ) ;
#12462=EDGE_CURVE ( 'NONE', #9140, #26271, #15243, .T. ) ;
#12465=LINE ( 'NONE', #15120, #13186 ) ;
#12474=CARTESIAN_POINT ( 'NONE',  ( 0.3582258883630317636, 11.68927977431952137, 12.00000000000000000 ) ) ;
#12475=VERTEX_POINT ( 'NONE', #21345 ) ;
#12480=EDGE_LOOP ( 'NONE', ( #25001, #6270 ) ) ;
#12491=VERTEX_POINT ( 'NONE', #12595 ) ;
#12495=AXIS2_PLACEMENT_3D ( 'NONE', #16946, #500, #19784 ) ;
#12504=LINE ( 'NONE', #19196, #35962 ) ;
#12506=AXIS2_PLACEMENT_3D ( 'NONE', #14720, #23461, #33223 ) ;
#12510=DIRECTION ( 'NONE',  ( 0.000000000000000000, 0.000000000000000000, 1.000000000000000000 ) ) ;
#12514=EDGE_CURVE ( 'NONE', #26968, #33412, #12201, .T. ) ;
#12525=FACE_OUTER_BOUND ( 'NONE', #19492, .T. ) ;
#12539=FACE_OUTER_BOUND ( 'NONE', #5328, .T. ) ;
#12540=CIRCLE ( 'NONE', #35241, 1.000000000000000888 ) ;
#12546=EDGE_LOOP ( 'NONE', ( #31894, #32692 ) ) ;
#12548=DIRECTION ( 'NONE',  ( 0.000000000000000000, 0.000000000000000000, 1.000000000000000000 ) ) ;
#12557=CARTESIAN_POINT ( 'NONE',  ( 15.21690391738993320, 27.44427296666788862, 13.00000000000000178 ) ) ;
#12558=DIRECTION ( 'NONE',  ( -0.000000000000000000, -0.000000000000000000, -1.000000000000000000 ) ) ;
#12559=ORIENTED_EDGE ( 'NONE', *, *, #6603, .T. ) ;
#12567=AXIS2_PLACEMENT_3D ( 'NONE', #10722, #32469, #13967 ) ;
#12569=EDGE_LOOP ( 'NONE', ( #21951, #27029, #12672, #17270 ) ) ;
#12583=CARTESIAN_POINT ( 'NONE',  ( -3.118678732975735279, 7.827785988993307242, 13.00000000000000178 ) ) ;
#12584=ORIENTED_EDGE ( 'NONE', *, *, #39945, .T. ) ;
#12595=CARTESIAN_POINT ( 'NONE',  ( 10.18324034840045478, 28.21559575157615996, 13.00000000000000178 ) ) ;
#12599=ORIENTED_EDGE ( 'NONE', *, *, #36274, .T. ) ;
#12603=EDGE_LOOP ( 'NONE', ( #3637, #5857, #34971, #4382 ) ) ;
#12606=DIRECTION ( 'NONE',  ( 0.000000000000000000, 0.000000000000000000, 1.000000000000000000 ) ) ;
#12620=CARTESIAN_POINT ( 'NONE',  ( 11.77090408390491305, 15.39748370681878775, 13.00000000000000178 ) ) ;
#12622=AXIS2_PLACEMENT_3D ( 'NONE', #36966, #18086, #30476 ) ;
#12627=FACE_OUTER_BOUND ( 'NONE', #33457, .T. ) ;
#12634=FACE_OUTER_BOUND ( 'NONE', #31590, .T. ) ;
#12651=VERTEX_POINT ( 'NONE', #26786 ) ;
#12654=AXIS2_PLACEMENT_3D ( 'NONE', #16485, #28872, #10387 ) ;
#12658=VECTOR ( 'NONE', #39106, 1000.000000000000000 ) ;
#12659=FACE_BOUND ( 'NONE', #38868, .T. ) ;
#12665=CARTESIAN_POINT ( 'NONE',  ( -7.312041872459064784, 25.58773265502866678, 13.00000000000000178 ) ) ;
#12667=VERTEX_POINT ( 'NONE', #2216 ) ;
#12670=CARTESIAN_POINT ( 'NONE',  ( 11.41267482483262619, 26.20820393249957192, 12.00000000000000000 ) ) ;
#12672=ORIENTED_EDGE ( 'NONE', *, *, #22769, .T. ) ;
#12678=DIRECTION ( 'NONE',  ( 1.000000000000000000, 0.000000000000000000, 0.000000000000000000 ) ) ;
#12689=VECTOR ( 'NONE', #39854, 1000.000000000000000 ) ;
#12698=VERTEX_POINT ( 'NONE', #30042 ) ;
#12701=DIRECTION ( 'NONE',  ( 0.000000000000000000, 0.000000000000000000, 1.000000000000000000 ) ) ;
#12708=DIRECTION ( 'NONE',  ( 1.000000000000000000, 0.000000000000000000, 0.000000000000000000 ) ) ;
#12713=AXIS2_PLACEMENT_3D ( 'NONE', #17234, #17438, #38349 ) ;
#12717=AXIS2_PLACEMENT_3D ( 'NONE', #22754, #28859, #35159 ) ;
#12735=ORIENTED_EDGE ( 'NONE', *, *, #6145, .T. ) ;
#12738=ORIENTED_EDGE ( 'NONE', *, *, #27897, .F. ) ;
#12742=EDGE_CURVE ( 'NONE', #4655, #20339, #6353, .T. ) ;
#12746=AXIS2_PLACEMENT_3D ( 'NONE', #11887, #5192, #2151 ) ;
#12754=DIRECTION ( 'NONE',  ( 0.000000000000000000, 0.000000000000000000, 1.000000000000000000 ) ) ;
#12761=CYLINDRICAL_SURFACE ( 'NONE', #22964, 1.000000000000000000 ) ;
#12780=DIRECTION ( 'NONE',  ( 1.000000000000000000, 0.000000000000000000, 0.000000000000000000 ) ) ;
#12783=CARTESIAN_POINT ( 'NONE',  ( -1.871208588069141143, 13.69667159339610762, 6.000000000000000000 ) ) ;
#12786=CARTESIAN_POINT ( 'NONE',  ( 11.77090408390491305, 15.39748370681878775, 13.00000000000000178 ) ) ;
#12789=DIRECTION ( 'NONE',  ( 0.000000000000000000, 0.000000000000000000, 1.000000000000000000 ) ) ;
#12792=EDGE_CURVE ( 'NONE', #14009, #33298, #14603, .T. ) ;
#12803=CIRCLE ( 'NONE', #38081, 1.000000000000000888 ) ;
#12808=DIRECTION ( 'NONE',  ( 0.000000000000000000, 0.000000000000000000, 1.000000000000000000 ) ) ;
#12813=CIRCLE ( 'NONE', #23867, 1.000000000000000000 ) ;
#12815=EDGE_CURVE ( 'NONE', #15842, #333, #13993, .T. ) ;
#12823=DIRECTION ( 'NONE',  ( 1.000000000000000000, 0.000000000000000000, 0.000000000000000000 ) ) ;
#12825=ORIENTED_EDGE ( 'NONE', *, *, #2219, .F. ) ;
#12829=FACE_BOUND ( 'NONE', #32113, .T. ) ;
#12830=CIRCLE ( 'NONE', #27742, 1.000000000000000000 ) ;
#12831=VECTOR ( 'NONE', #30982, 1000.000000000000000 ) ;
#12832=VERTEX_POINT ( 'NONE', #21098 ) ;
#12836=VERTEX_POINT ( 'NONE', #12347 ) ;
#12849=VERTEX_POINT ( 'NONE', #24139 ) ;
#12850=CYLINDRICAL_SURFACE ( 'NONE', #38342, 1.000000000000000000 ) ;
#12856=FACE_BOUND ( 'NONE', #7609, .T. ) ;
#12864=EDGE_LOOP ( 'NONE', ( #35534, #8312, #19786, #7983 ) ) ;
#12866=EDGE_CURVE ( 'NONE', #32396, #33978, #40121, .T. ) ;
#12872=ORIENTED_EDGE ( 'NONE', *, *, #29294, .F. ) ;
#12876=CARTESIAN_POINT ( 'NONE',  ( 7.330070799514983193, 27.28854476845134513, 6.000000000000000000 ) ) ;
#12888=ADVANCED_FACE ( 'NONE', ( #9307 ), #31046, .F. ) ;
#12891=CIRCLE ( 'NONE', #35605, 1.000000000000000000 ) ;
#12893=AXIS2_PLACEMENT_3D ( 'NONE', #20277, #8685, #30018 ) ;
#12898=DIRECTION ( 'NONE',  ( 0.000000000000000000, 0.000000000000000000, 1.000000000000000000 ) ) ;
#12901=DIRECTION ( 'NONE',  ( 0.000000000000000000, 0.000000000000000000, 1.000000000000000000 ) ) ;
#12923=AXIS2_PLACEMENT_3D ( 'NONE', #9165, #30901, #15861 ) ;
#12926=LINE ( 'NONE', #15182, #8168 ) ;
#12932=VERTEX_POINT ( 'NONE', #3400 ) ;
#12939=EDGE_LOOP ( 'NONE', ( #8608, #17877 ) ) ;
#12942=EDGE_CURVE ( 'NONE', #21619, #31370, #39454, .T. ) ;
#12947=ORIENTED_EDGE ( 'NONE', *, *, #2912, .F. ) ;
#12948=EDGE_LOOP ( 'NONE', ( #28906, #25288 ) ) ;
#12949=ADVANCED_FACE ( 'NONE', ( #36939 ), #30450, .F. ) ;
#12957=CARTESIAN_POINT ( 'NONE',  ( 2.605696033269626177, 17.55816537872232530, 12.00000000000000000 ) ) ;
#12958=DIRECTION ( 'NONE',  ( 0.000000000000000000, 0.000000000000000000, 1.000000000000000000 ) ) ;
#12983=EDGE_LOOP ( 'NONE', ( #25627, #24043, #34494, #27307 ) ) ;
#12985=CARTESIAN_POINT ( 'NONE',  ( 13.26584437371809777, 27.13525491562438319, 6.000000000000000000 ) ) ;
#12988=VERTEX_POINT ( 'NONE', #39975 ) ;
#12999=CARTESIAN_POINT ( 'NONE',  ( 11.16520467992603294, 20.33931832809677331, 13.00000000000000178 ) ) ;
#13002=ORIENTED_EDGE ( 'NONE', *, *, #15926, .F. ) ;
#13003=DIRECTION ( 'NONE',  ( 1.000000000000000000, 0.000000000000000000, 0.000000000000000000 ) ) ;
#13005=DIRECTION ( 'NONE',  ( 1.000000000000000000, 0.000000000000000000, 0.000000000000000000 ) ) ;
#13021=ORIENTED_EDGE ( 'NONE', *, *, #23913, .F. ) ;
#13025=FACE_BOUND ( 'NONE', #16401, .T. ) ;
#13031=DIRECTION ( 'NONE',  ( 0.000000000000000000, 0.000000000000000000, 1.000000000000000000 ) ) ;
#13037=ORIENTED_EDGE ( 'NONE', *, *, #26727, .T. ) ;
#13039=DIRECTION ( 'NONE',  ( 0.000000000000000000, 0.000000000000000000, 1.000000000000000000 ) ) ;
#13041=VERTEX_POINT ( 'NONE', #9900 ) ;
#13045=CYLINDRICAL_SURFACE ( 'NONE', #7708, 16.99999999999999645 ) ;
#13048=FACE_BOUND ( 'NONE', #30721, .T. ) ;
#13076=AXIS2_PLACEMENT_3D ( 'NONE', #37343, #567, #168 ) ;
#13077=DIRECTION ( 'NONE',  ( 0.000000000000000000, 0.000000000000000000, 1.000000000000000000 ) ) ;
#13078=DIRECTION ( 'NONE',  ( 0.000000000000000000, 0.000000000000000000, 1.000000000000000000 ) ) ;
#13091=FACE_OUTER_BOUND ( 'NONE', #18936, .T. ) ;
#13103=CARTESIAN_POINT ( 'NONE',  ( -12.01838097023000529, 23.73363068877903359, 12.00000000000000000 ) ) ;
#13104=CARTESIAN_POINT ( 'NONE',  ( -7.312041872459064784, 25.58773265502866678, 6.000000000000000000 ) ) ;
#13105=ADVANCED_FACE ( 'NONE', ( #28787 ), #7238, .F. ) ;
#13111=DIRECTION ( 'NONE',  ( 0.000000000000000000, 0.000000000000000000, 1.000000000000000000 ) ) ;
#13127=DIRECTION ( 'NONE',  ( -0.000000000000000000, -0.000000000000000000, -1.000000000000000000 ) ) ;
#13131=EDGE_CURVE ( 'NONE', #20339, #37305, #16604, .T. ) ;
#13134=EDGE_LOOP ( 'NONE', ( #32941, #831, #30296, #28742 ) ) ;
#13144=ORIENTED_EDGE ( 'NONE', *, *, #1376, .T. ) ;
#13146=DIRECTION ( 'NONE',  ( 0.000000000000000000, 0.000000000000000000, 1.000000000000000000 ) ) ;
#13147=CIRCLE ( 'NONE', #12495, 1.000000000000000888 ) ;
#13153=DIRECTION ( 'NONE',  ( 0.000000000000000000, 0.000000000000000000, 1.000000000000000000 ) ) ;
#13154=CARTESIAN_POINT ( 'NONE',  ( 1.265502442671760264, 36.24516302788250499, 6.000000000000000000 ) ) ;
#13158=ORIENTED_EDGE ( 'NONE', *, *, #9815, .T. ) ;
#13160=DIRECTION ( 'NONE',  ( 0.000000000000000000, 0.000000000000000000, 1.000000000000000000 ) ) ;
#13167=CARTESIAN_POINT ( 'NONE',  ( 4.440829913680675034, 10.60893893836775348, 6.000000000000000000 ) ) ;
#13172=AXIS2_PLACEMENT_3D ( 'NONE', #12280, #34611, #30581 ) ;
#13175=ORIENTED_EDGE ( 'NONE', *, *, #27650, .T. ) ;
#13177=AXIS2_PLACEMENT_3D ( 'NONE', #2030, #32299, #20111 ) ;
#13178=DIRECTION ( 'NONE',  ( 0.000000000000000000, 0.000000000000000000, 1.000000000000000000 ) ) ;
#13186=VECTOR ( 'NONE', #24857, 1000.000000000000000 ) ;
#13196=CIRCLE ( 'NONE', #35924, 1.000000000000000888 ) ;
#13217=FACE_OUTER_BOUND ( 'NONE', #33564, .T. ) ;
#13219=VERTEX_POINT ( 'NONE', #29994 ) ;
#13223=FACE_BOUND ( 'NONE', #21301, .T. ) ;
#13227=EDGE_LOOP ( 'NONE', ( #14845, #35933, #7243, #38899 ) ) ;
#13232=EDGE_LOOP ( 'NONE', ( #29492, #20880 ) ) ;
#13246=VECTOR ( 'NONE', #23810, 1000.000000000000000 ) ;
#13249=PRODUCT ( 'Protective Beveled Outer Blade Guard', 'Protective Beveled Outer Blade Guard', '', ( #1017 ) ) ;
#13251=FACE_BOUND ( 'NONE', #12546, .T. ) ;
#13256=ADVANCED_FACE ( 'NONE', ( #32653 ), #17420, .F. ) ;
#13257=ORIENTED_EDGE ( 'NONE', *, *, #21062, .F. ) ;
#13269=DIRECTION ( 'NONE',  ( 1.000000000000000000, 0.000000000000000000, 0.000000000000000000 ) ) ;
#13275=FACE_OUTER_BOUND ( 'NONE', #35931, .T. ) ;
#13287=EDGE_CURVE ( 'NONE', #36438, #13219, #14199, .T. ) ;
#13292=ORIENTED_EDGE ( 'NONE', *, *, #21163, .F. ) ;
#13293=DIRECTION ( 'NONE',  ( 0.000000000000000000, 0.000000000000000000, 1.000000000000000000 ) ) ;
#13295=FACE_OUTER_BOUND ( 'NONE', #32891, .T. ) ;
#13298=CARTESIAN_POINT ( 'NONE',  ( -2.587667106213709101, 35.31811204475769728, 13.00000000000000178 ) ) ;
#13303=EDGE_CURVE ( 'NONE', #8057, #26968, #29795, .T. ) ;
#13306=DIRECTION ( 'NONE',  ( 1.000000000000000000, 0.000000000000000000, 0.000000000000000000 ) ) ;
#13307=EDGE_LOOP ( 'NONE', ( #5344, #18503 ) ) ;
#13309=CARTESIAN_POINT ( 'NONE',  ( 2.247466774197339756, 28.36888560440311480, 6.000000000000000000 ) ) ;
#13329=EDGE_LOOP ( 'NONE', ( #36152, #24643 ) ) ;
#13339=EDGE_CURVE ( 'NONE', #19934, #24994, #17468, .T. ) ;
#13346=CARTESIAN_POINT ( 'NONE',  ( -0.9819677022348329842, 30.37627742347970283, 6.000000000000000000 ) ) ;
#13347=AXIS2_PLACEMENT_3D ( 'NONE', #3526, #31760, #34608 ) ;
#13350=CIRCLE ( 'NONE', #31515, 1.000000000000000888 ) ;
#13351=CARTESIAN_POINT ( 'NONE',  ( 7.577540944421576441, 33.15743037285414374, 13.00000000000000178 ) ) ;
#13352=ORIENTED_EDGE ( 'NONE', *, *, #7998, .T. ) ;
#13354=DIRECTION ( 'NONE',  ( 0.000000000000000000, 0.000000000000000000, 1.000000000000000000 ) ) ;
#13358=DIRECTION ( 'NONE',  ( 0.000000000000000000, 0.000000000000000000, 1.000000000000000000 ) ) ;
#13364=ORIENTED_EDGE ( 'NONE', *, *, #29494, .F. ) ;
#13368=ADVANCED_FACE ( 'NONE', ( #28083 ), #657, .F. ) ;
#13378=DIRECTION ( 'NONE',  ( 1.000000000000000000, 0.000000000000000000, 0.000000000000000000 ) ) ;
#13379=CARTESIAN_POINT ( 'NONE',  ( -8.935776944912362296, 22.65328985282726393, 13.00000000000000178 ) ) ;
#13380=EDGE_LOOP ( 'NONE', ( #5099, #37129 ) ) ;
#13393=EDGE_LOOP ( 'NONE', ( #38742, #30335, #7244, #38053 ) ) ;
#13413=CARTESIAN_POINT ( 'NONE',  ( 6.082600654608392610, 21.41965916404854298, 6.000000000000000000 ) ) ;
#13417=LINE ( 'NONE', #38604, #26328 ) ;
#13418=EDGE_LOOP ( 'NONE', ( #14854, #6108, #6731, #37887, #29685, #20703 ) ) ;
#13422=DIRECTION ( 'NONE',  ( 0.000000000000000000, 0.000000000000000000, 1.000000000000000000 ) ) ;
#13429=CARTESIAN_POINT ( 'NONE',  ( 7.312035131040564906, 19.41226734497195849, 12.00000000000000000 ) ) ;
#13439=AXIS2_PLACEMENT_3D ( 'NONE', #33200, #30547, #14700 ) ;
#13440=VECTOR ( 'NONE', #33696, 1000.000000000000000 ) ;
#13441=LINE ( 'NONE', #4302, #6391 ) ;
#13444=ORIENTED_EDGE ( 'NONE', *, *, #18952, .F. ) ;
#13451=EDGE_CURVE ( 'NONE', #39486, #6684, #6935, .T. ) ;
#13457=EDGE_LOOP ( 'NONE', ( #33937, #37507, #502, #31842 ) ) ;
#13470=VERTEX_POINT ( 'NONE', #22782 ) ;
#13476=CIRCLE ( 'NONE', #18681, 1.000000000000000000 ) ;
#13482=ORIENTED_EDGE ( 'NONE', *, *, #31335, .F. ) ;
#13486=EDGE_LOOP ( 'NONE', ( #32167, #39668, #21937, #17003 ) ) ;
#13504=ORIENTED_EDGE ( 'NONE', *, *, #10388, .F. ) ;
#13506=DIRECTION ( 'NONE',  ( 0.000000000000000000, 0.000000000000000000, 1.000000000000000000 ) ) ;
#13515=EDGE_CURVE ( 'NONE', #15244, #22373, #13441, .T. ) ;
#13537=AXIS2_PLACEMENT_3D ( 'NONE', #14914, #17779, #39881 ) ;
#13548=VERTEX_POINT ( 'NONE', #16910 ) ;
#13554=ORIENTED_EDGE ( 'NONE', *, *, #5509, .F. ) ;
#13563=DIRECTION ( 'NONE',  ( 1.000000000000000000, 0.000000000000000000, 0.000000000000000000 ) ) ;
#13578=CARTESIAN_POINT ( 'NONE',  ( 6.348106467989403257, 35.16482219193073178, 12.00000000000000000 ) ) ;
#13580=VERTEX_POINT ( 'NONE', #7070 ) ;
#13582=ORIENTED_EDGE ( 'NONE', *, *, #3268, .F. ) ;
#13583=VECTOR ( 'NONE', #7816, 1000.000000000000000 ) ;
#13585=ORIENTED_EDGE ( 'NONE', *, *, #17620, .F. ) ;
#13587=CARTESIAN_POINT ( 'NONE',  ( -7.917741276437941345, 30.52956727630665057, 13.00000000000000178 ) ) ;
#13590=PRODUCT_DEFINITION_SHAPE ( 'NONE', 'NONE',  #17230 ) ;
#13603=EDGE_CURVE ( 'NONE', #27813, #37255, #16230, .T. ) ;
#13604=CARTESIAN_POINT ( 'NONE',  ( -0.6057027746881266106, 27.44183462127829642, 12.00000000000000000 ) ) ;
#13615=LINE ( 'NONE', #3123, #10372 ) ;
#13617=DIRECTION ( 'NONE',  ( 0.000000000000000000, 0.000000000000000000, 1.000000000000000000 ) ) ;
#13627=VERTEX_POINT ( 'NONE', #9735 ) ;
#13632=FACE_BOUND ( 'NONE', #22168, .T. ) ;
#13648=ADVANCED_FACE ( 'NONE', ( #34318 ), #9537, .F. ) ;
#13691=CIRCLE ( 'NONE', #38371, 1.000000000000000000 ) ;
#13700=CIRCLE ( 'NONE', #14355, 1.000000000000000888 ) ;
#13702=DIRECTION ( 'NONE',  ( 1.000000000000000000, 0.000000000000000000, 0.000000000000000000 ) ) ;
#13708=CARTESIAN_POINT ( 'NONE',  ( 0.3582258883630317636, 11.68927977431952137, 6.000000000000000000 ) ) ;
#13711=DIRECTION ( 'NONE',  ( 0.000000000000000000, 0.000000000000000000, 1.000000000000000000 ) ) ;
#13712=ORIENTED_EDGE ( 'NONE', *, *, #6811, .T. ) ;
#13713=AXIS2_PLACEMENT_3D ( 'NONE', #37943, #37350, #30861 ) ;
#13717=EDGE_CURVE ( 'NONE', #36138, #839, #15472, .T. ) ;
#13739=ORIENTED_EDGE ( 'NONE', *, *, #7998, .F. ) ;
#13742=ORIENTED_EDGE ( 'NONE', *, *, #11291, .F. ) ;
#13744=DIRECTION ( 'NONE',  ( 1.000000000000000000, 0.000000000000000000, 0.000000000000000000 ) ) ;
#13745=DIRECTION ( 'NONE',  ( 0.000000000000000000, 0.000000000000000000, 1.000000000000000000 ) ) ;
#13754=EDGE_LOOP ( 'NONE', ( #6739, #32294 ) ) ;
#13763=CARTESIAN_POINT ( 'NONE',  ( -7.688306800005769048, 28.52217545723006609, 13.00000000000000178 ) ) ;
#13768=CARTESIAN_POINT ( 'NONE',  ( -4.706342468480190000, 20.64589803375067945, 13.00000000000000178 ) ) ;
#13785=ORIENTED_EDGE ( 'NONE', *, *, #12462, .T. ) ;
#13794=ORIENTED_EDGE ( 'NONE', *, *, #26745, .F. ) ;
#13797=ORIENTED_EDGE ( 'NONE', *, *, #35945, .T. ) ;
#13800=ADVANCED_FACE ( 'NONE', ( #4436 ), #16635, .F. ) ;
#13805=EDGE_LOOP ( 'NONE', ( #3574, #28919 ) ) ;
#13817=LINE ( 'NONE', #14021, #406 ) ;
#13823=EDGE_CURVE ( 'NONE', #28074, #35813, #991, .T. ) ;
#13826=ORIENTED_EDGE ( 'NONE', *, *, #29165, .F. ) ;
#13827=ORIENTED_EDGE ( 'NONE', *, *, #14570, .F. ) ;
#13831=CARTESIAN_POINT ( 'NONE',  ( -0.2655091840902661926, 8.754836972118123839, 13.00000000000000178 ) ) ;
#13832=EDGE_CURVE ( 'NONE', #29063, #29833, #37546, .T. ) ;
#13834=FACE_OUTER_BOUND ( 'NONE', #1558, .T. ) ;
#13841=VERTEX_POINT ( 'NONE', #4637 ) ;
#13854=EDGE_CURVE ( 'NONE', #6833, #27468, #12891, .T. ) ;
#13858=AXIS2_PLACEMENT_3D ( 'NONE', #26193, #4464, #38586 ) ;
#13870=EDGE_CURVE ( 'NONE', #38519, #10872, #23309, .T. ) ;
#13872=AXIS2_PLACEMENT_3D ( 'NONE', #32259, #35910, #10517 ) ;
#13876=EDGE_CURVE ( 'NONE', #39039, #26584, #16426, .T. ) ;
#13884=DIRECTION ( 'NONE',  ( 0.000000000000000000, 0.000000000000000000, 1.000000000000000000 ) ) ;
#13887=VECTOR ( 'NONE', #7245, 1000.000000000000000 ) ;
#13891=CARTESIAN_POINT ( 'NONE',  ( 3.853166178176219425, 23.42705098312512746, 13.00000000000000178 ) ) ;
#13897=ORIENTED_EDGE ( 'NONE', *, *, #10143, .T. ) ;
#13906=DIRECTION ( 'NONE',  ( 0.000000000000000000, 0.000000000000000000, 1.000000000000000000 ) ) ;
#13919=SURFACE_STYLE_FILL_AREA ( #38706 ) ;
#13926=ORIENTED_EDGE ( 'NONE', *, *, #19107, .T. ) ;
#13928=ORIENTED_EDGE ( 'NONE', *, *, #31238, .F. ) ;
#13932=AXIS2_PLACEMENT_3D ( 'NONE', #10129, #34513, #32060 ) ;
#13938=DIRECTION ( 'NONE',  ( 1.000000000000000000, 0.000000000000000000, 0.000000000000000000 ) ) ;
#13942=ORIENTED_EDGE ( 'NONE', *, *, #32878, .F. ) ;
#13949=CARTESIAN_POINT ( 'NONE',  ( 3.118671991557230516, 37.17221401100731981, 12.00000000000000000 ) ) ;
#13953=ORIENTED_EDGE ( 'NONE', *, *, #25058, .T. ) ;
#13958=DIRECTION ( 'NONE',  ( 1.000000000000000000, 0.000000000000000000, 0.000000000000000000 ) ) ;
#13961=FACE_OUTER_BOUND ( 'NONE', #8865, .T. ) ;
#13963=EDGE_CURVE ( 'NONE', #2398, #6680, #38209, .T. ) ;
#13964=AXIS2_PLACEMENT_3D ( 'NONE', #12670, #36864, #18774 ) ;
#13965=DIRECTION ( 'NONE',  ( 1.000000000000000000, 0.000000000000000000, 0.000000000000000000 ) ) ;
#13966=DIRECTION ( 'NONE',  ( 1.000000000000000000, 0.000000000000000000, 0.000000000000000000 ) ) ;
#13967=DIRECTION ( 'NONE',  ( 1.000000000000000000, 0.000000000000000000, 0.000000000000000000 ) ) ;
#13970=ORIENTED_EDGE ( 'NONE', *, *, #4916, .F. ) ;
#13972=AXIS2_PLACEMENT_3D ( 'NONE', #5, #34527, #3443 ) ;
#13974=LINE ( 'NONE', #32678, #21795 ) ;
#13976=LINE ( 'NONE', #35919, #34061 ) ;
#13979=CARTESIAN_POINT ( 'NONE',  ( 2.494936919103933448, 34.23777120880591696, 12.00000000000000000 ) ) ;
#13993=LINE ( 'NONE', #17463, #23892 ) ;
#14000=AXIS2_PLACEMENT_3D ( 'NONE', #9287, #37716, #6032 ) ;
#14009=VERTEX_POINT ( 'NONE', #36326 ) ;
#14011=CARTESIAN_POINT ( 'NONE',  ( 3.211395437248501850, 12.61633075744433796, 12.00000000000000000 ) ) ;
#14012=CARTESIAN_POINT ( 'NONE',  ( 3.476901250629512941, 26.36149378532653031, 13.00000000000000178 ) ) ;
#14021=CARTESIAN_POINT ( 'NONE',  ( -7.559512017365658920, 19.71884705062586107, 6.000000000000000000 ) ) ;
#14027=EDGE_CURVE ( 'NONE', #26803, #11791, #20889, .T. ) ;
#14028=CARTESIAN_POINT ( 'NONE',  ( 1.265502442671760264, 36.24516302788250499, 12.00000000000000000 ) ) ;
#14034=FACE_BOUND ( 'NONE', #39026, .T. ) ;
#14036=DIRECTION ( 'NONE',  ( 1.000000000000000000, 0.000000000000000000, 0.000000000000000000 ) ) ;
#14051=CARTESIAN_POINT ( 'NONE',  ( -3.835137251120299684, 29.44922644035488446, 12.00000000000000000 ) ) ;
#14055=CARTESIAN_POINT ( 'NONE',  ( 9.917734535019443243, 14.47043272369397116, 12.00000000000000000 ) ) ;
#14056=VERTEX_POINT ( 'NONE', #11939 ) ;
#14057=CYLINDRICAL_SURFACE ( 'NONE', #27328, 1.000000000000000888 ) ;
#14063=CARTESIAN_POINT ( 'NONE',  ( 5.706335727061685681, 24.35410196624994583, 12.00000000000000000 ) ) ;
#14064=DIRECTION ( 'NONE',  ( 1.000000000000000000, 0.000000000000000000, 0.000000000000000000 ) ) ;
#14065=ORIENTED_EDGE ( 'NONE', *, *, #37203, .T. ) ;
#14074=ORIENTED_EDGE ( 'NONE', *, *, #3758, .T. ) ;
#14076=DIRECTION ( 'NONE',  ( 0.000000000000000000, 0.000000000000000000, 1.000000000000000000 ) ) ;
#14080=EDGE_CURVE ( 'NONE', #28074, #10357, #18757, .T. ) ;
#14083=ORIENTED_EDGE ( 'NONE', *, *, #35845, .T. ) ;
#14091=DIRECTION ( 'NONE',  ( 1.000000000000000000, 0.000000000000000000, 0.000000000000000000 ) ) ;
#14104=ADVANCED_FACE ( 'NONE', ( #38858 ), #26661, .F. ) ;
#14106=EDGE_CURVE ( 'NONE', #17784, #3811, #15510, .T. ) ;
#14113=CARTESIAN_POINT ( 'NONE',  ( 2.118671991557230516, 37.17221401100731981, 13.00000000000000178 ) ) ;
#14115=CIRCLE ( 'NONE', #35529, 1.000000000000000000 ) ;
#14117=CARTESIAN_POINT ( 'NONE',  ( -10.78894649379783388, 21.72623886970244911, 12.00000000000000000 ) ) ;
#14121=VERTEX_POINT ( 'NONE', #37707 ) ;
#14129=VERTEX_POINT ( 'NONE', #20379 ) ;
#14132=EDGE_CURVE ( 'NONE', #31370, #21619, #4482, .T. ) ;
#14135=EDGE_CURVE ( 'NONE', #22373, #7177, #9044, .T. ) ;
#14142=CYLINDRICAL_SURFACE ( 'NONE', #25095, 1.000000000000000000 ) ;
#14144=CIRCLE ( 'NONE', #31649, 1.000000000000000000 ) ;
#14152=DIRECTION ( 'NONE',  ( 1.000000000000000000, 0.000000000000000000, 0.000000000000000000 ) ) ;
#14157=EDGE_CURVE ( 'NONE', #8090, #24274, #31601, .T. ) ;
#14158=ORIENTED_EDGE ( 'NONE', *, *, #11585, .F. ) ;
#14162=DIRECTION ( 'NONE',  ( 1.000000000000000000, 0.000000000000000000, 0.000000000000000000 ) ) ;
#14165=DIRECTION ( 'NONE',  ( 0.000000000000000000, 0.000000000000000000, 1.000000000000000000 ) ) ;
#14169=CARTESIAN_POINT ( 'NONE',  ( 6.064564986133971658, 13.54338174056915456, 12.00000000000000000 ) ) ;
#14170=AXIS2_PLACEMENT_3D ( 'NONE', #699, #35636, #25671 ) ;
#14186=LINE ( 'NONE', #1602, #36792 ) ;
#14190=ORIENTED_EDGE ( 'NONE', *, *, #21163, .T. ) ;
#14192=ORIENTED_EDGE ( 'NONE', *, *, #27799, .T. ) ;
#14193=DIRECTION ( 'NONE',  ( 0.000000000000000000, -1.000000000000000000, 0.000000000000000000 ) ) ;
#14197=EDGE_LOOP ( 'NONE', ( #30339, #21513, #2706, #19642 ) ) ;
#14199=CIRCLE ( 'NONE', #28457, 1.000000000000000000 ) ;
#14202=ORIENTED_EDGE ( 'NONE', *, *, #19053, .F. ) ;
#14210=LINE ( 'NONE', #27007, #22000 ) ;
#14213=DIRECTION ( 'NONE',  ( 1.000000000000000000, 0.000000000000000000, 0.000000000000000000 ) ) ;
#14221=CARTESIAN_POINT ( 'NONE',  ( 1.871201846650637046, 31.30332840660451765, 6.000000000000000000 ) ) ;
#14223=VECTOR ( 'NONE', #20579, 1000.000000000000000 ) ;
#14225=AXIS2_PLACEMENT_3D ( 'NONE', #39950, #15174, #15972 ) ;
#14230=EDGE_LOOP ( 'NONE', ( #4788, #14083 ) ) ;
#14232=CIRCLE ( 'NONE', #12923, 1.000000000000000888 ) ;
#14236=FACE_BOUND ( 'NONE', #39887, .T. ) ;
#14238=CARTESIAN_POINT ( 'NONE',  ( 3.853166178176219425, 23.42705098312512746, 12.00000000000000000 ) ) ;
#14245=EDGE_CURVE ( 'NONE', #5502, #26852, #33707, .T. ) ;
#14246=VERTEX_POINT ( 'NONE', #8175 ) ;
#14248=CARTESIAN_POINT ( 'NONE',  ( 13.64210930126480115, 24.20081211342298744, 6.000000000000000000 ) ) ;
#14252=ORIENTED_EDGE ( 'NONE', *, *, #22114, .T. ) ;
#14255=CYLINDRICAL_SURFACE ( 'NONE', #25375, 1.000000000000000000 ) ;
#14260=DIRECTION ( 'NONE',  ( 1.000000000000000000, 0.000000000000000000, 0.000000000000000000 ) ) ;
#14261=EDGE_CURVE ( 'NONE', #29047, #16453, #25705, .T. ) ;
#14264=AXIS2_PLACEMENT_3D ( 'NONE', #28593, #32460, #19447 ) ;
#14271=DIRECTION ( 'NONE',  ( 0.000000000000000000, 0.000000000000000000, 1.000000000000000000 ) ) ;
#14272=ORIENTED_EDGE ( 'NONE', *, *, #10012, .F. ) ;
#14279=ORIENTED_EDGE ( 'NONE', *, *, #30897, .T. ) ;
#14287=ORIENTED_EDGE ( 'NONE', *, *, #2418, .F. ) ;
#14292=ORIENTED_EDGE ( 'NONE', *, *, #30537, .F. ) ;
#14296=AXIS2_PLACEMENT_3D ( 'NONE', #29949, #1520, #11072 ) ;
#14305=CARTESIAN_POINT ( 'NONE',  ( -1.871208588069141143, 13.69667159339610762, 13.00000000000000178 ) ) ;
#14307=DIRECTION ( 'NONE',  ( 1.000000000000000000, 0.000000000000000000, 0.000000000000000000 ) ) ;
#14308=EDGE_CURVE ( 'NONE', #32913, #12698, #19967, .T. ) ;
#14312=FACE_OUTER_BOUND ( 'NONE', #24364, .T. ) ;
#14323=ORIENTED_EDGE ( 'NONE', *, *, #9034, .F. ) ;
#14329=ORIENTED_EDGE ( 'NONE', *, *, #24021, .F. ) ;
#14331=ORIENTED_EDGE ( 'NONE', *, *, #8610, .F. ) ;
#14333=CARTESIAN_POINT ( 'NONE',  ( -5.064571727552472424, 31.45661825943146894, 12.00000000000000000 ) ) ;
#14337=AXIS2_PLACEMENT_3D ( 'NONE', #39442, #5511, #39243 ) ;
#14345=DIRECTION ( 'NONE',  ( 0.000000000000000000, 0.000000000000000000, 1.000000000000000000 ) ) ;
#14346=CARTESIAN_POINT ( 'NONE',  ( -1.587667106213708879, 35.31811204475769728, 6.000000000000000000 ) ) ;
#14355=AXIS2_PLACEMENT_3D ( 'NONE', #3619, #12958, #6460 ) ;
#14359=ADVANCED_FACE ( 'NONE', ( #33962 ), #40045, .F. ) ;
#14360=DIRECTION ( 'NONE',  ( 0.000000000000000000, 0.000000000000000000, 1.000000000000000000 ) ) ;
#14362=EDGE_CURVE ( 'NONE', #11948, #32551, #14878, .T. ) ;
#14363=AXIS2_PLACEMENT_3D ( 'NONE', #428, #12808, #13005 ) ;
#14367=CIRCLE ( 'NONE', #2051, 1.000000000000000888 ) ;
#14368=CARTESIAN_POINT ( 'NONE',  ( 0.2474667741973399226, 28.36888560440311480, 13.00000000000000178 ) ) ;
#14370=FACE_OUTER_BOUND ( 'NONE', #31043, .T. ) ;
#14371=DIRECTION ( 'NONE',  ( 1.000000000000000000, 0.000000000000000000, 0.000000000000000000 ) ) ;
#14372=DIRECTION ( 'NONE',  ( 1.000000000000000000, 0.000000000000000000, 0.000000000000000000 ) ) ;
#14379=CIRCLE ( 'NONE', #3355, 1.000000000000000000 ) ;
#14385=EDGE_CURVE ( 'NONE', #20919, #9948, #26556, .T. ) ;
#14395=ORIENTED_EDGE ( 'NONE', *, *, #29376, .F. ) ;
#14396=VECTOR ( 'NONE', #18864, 1000.000000000000000 ) ;
#14399=DIRECTION ( 'NONE',  ( 1.000000000000000000, 0.000000000000000000, 0.000000000000000000 ) ) ;
#14400=DIRECTION ( 'NONE',  ( 0.000000000000000000, 0.000000000000000000, 1.000000000000000000 ) ) ;
#14403=EDGE_LOOP ( 'NONE', ( #21842, #13021, #28699, #4606 ) ) ;
#14405=ORIENTED_EDGE ( 'NONE', *, *, #35945, .F. ) ;
#14407=CIRCLE ( 'NONE', #32602, 16.00000000000000000 ) ;
#14408=CARTESIAN_POINT ( 'NONE',  ( 11.03640989728592281, 29.14264673470096767, 12.00000000000000000 ) ) ;
#14409=ORIENTED_EDGE ( 'NONE', *, *, #12109, .F. ) ;
#14413=EDGE_LOOP ( 'NONE', ( #13364, #10462 ) ) ;
#14414=CARTESIAN_POINT ( 'NONE',  ( 3.587660364795204782, 9.681887955242936883, 6.000000000000000000 ) ) ;
#14420=VECTOR ( 'NONE', #17980, 1000.000000000000000 ) ;
#14429=ORIENTED_EDGE ( 'NONE', *, *, #22803, .T. ) ;
#14433=CARTESIAN_POINT ( 'NONE',  ( 9.559505275947156377, 25.28115294937476065, 13.00000000000000178 ) ) ;
#14435=DIRECTION ( 'NONE',  ( 0.000000000000000000, 0.000000000000000000, 1.000000000000000000 ) ) ;
#14455=ORIENTED_EDGE ( 'NONE', *, *, #26286, .F. ) ;
#14459=CARTESIAN_POINT ( 'NONE',  ( -6.935776944912362296, 22.65328985282726393, 6.000000000000000000 ) ) ;
#14466=EDGE_CURVE ( 'NONE', #3606, #20361, #6414, .T. ) ;
#14472=CIRCLE ( 'NONE', #33315, 1.000000000000000888 ) ;
#14474=VERTEX_POINT ( 'NONE', #24414 ) ;
#14477=FACE_OUTER_BOUND ( 'NONE', #21642, .T. ) ;
#14479=ORIENTED_EDGE ( 'NONE', *, *, #26745, .T. ) ;
#14493=LINE ( 'NONE', #11453, #34908 ) ;
#14500=VECTOR ( 'NONE', #8430, 1000.000000000000000 ) ;
#14505=AXIS2_PLACEMENT_3D ( 'NONE', #4166, #17790, #26516 ) ;
#14508=CARTESIAN_POINT ( 'NONE',  ( 13.26584437371809777, 27.13525491562438319, 13.00000000000000178 ) ) ;
#14510=CIRCLE ( 'NONE', #33977, 1.000000000000000000 ) ;
#14514=EDGE_LOOP ( 'NONE', ( #34768, #28034 ) ) ;
#14523=EDGE_LOOP ( 'NONE', ( #31161, #33367, #16892, #34801 ) ) ;
#14525=AXIS2_PLACEMENT_3D ( 'NONE', #28191, #31641, #566 ) ;
#14534=DIRECTION ( 'NONE',  ( 0.000000000000000000, 0.000000000000000000, 1.000000000000000000 ) ) ;
#14546=ADVANCED_FACE ( 'NONE', ( #24811 ), #34165, .F. ) ;
#14554=DIRECTION ( 'NONE',  ( 1.000000000000000000, 0.000000000000000000, 0.000000000000000000 ) ) ;
#14557=CYLINDRICAL_SURFACE ( 'NONE', #16427, 1.000000000000000888 ) ;
#14559=VECTOR ( 'NONE', #9066, 1000.000000000000000 ) ;
#14560=VERTEX_POINT ( 'NONE', #25603 ) ;
#14570=EDGE_CURVE ( 'NONE', #10495, #12849, #1826, .T. ) ;
#14572=CARTESIAN_POINT ( 'NONE',  ( 1.247466774197339978, 28.36888560440311480, 13.00000000000000178 ) ) ;
#14573=LINE ( 'NONE', #20270, #23646 ) ;
#14577=DIRECTION ( 'NONE',  ( 1.000000000000000000, 0.000000000000000000, 0.000000000000000000 ) ) ;
#14595=ORIENTED_EDGE ( 'NONE', *, *, #20302, .T. ) ;
#14599=EDGE_CURVE ( 'NONE', #6144, #19765, #15443, .T. ) ;
#14602=DIRECTION ( 'NONE',  ( 0.000000000000000000, 0.000000000000000000, 1.000000000000000000 ) ) ;
#14603=LINE ( 'NONE', #20503, #38145 ) ;
#14619=EDGE_CURVE ( 'NONE', #28635, #19790, #14144, .T. ) ;
#14621=DIRECTION ( 'NONE',  ( 0.000000000000000000, 0.000000000000000000, 1.000000000000000000 ) ) ;
#14625=VERTEX_POINT ( 'NONE', #22158 ) ;
#14635=LINE ( 'NONE', #33539, #11455 ) ;
#14639=AXIS2_PLACEMENT_3D ( 'NONE', #25313, #32215, #37711 ) ;
#14644=VECTOR ( 'NONE', #39667, 1000.000000000000000 ) ;
#14648=DIRECTION ( 'NONE',  ( 0.000000000000000000, 0.000000000000000000, 1.000000000000000000 ) ) ;
#14657=EDGE_LOOP ( 'NONE', ( #548, #29340, #37138, #29448 ) ) ;
#14671=CARTESIAN_POINT ( 'NONE',  ( -3.476907992048017260, 18.63850621467409496, 6.000000000000000000 ) ) ;
#14685=VERTEX_POINT ( 'NONE', #3875 ) ;
#14700=DIRECTION ( 'NONE',  ( 1.000000000000000000, 0.000000000000000000, 0.000000000000000000 ) ) ;
#14708=AXIS2_PLACEMENT_3D ( 'NONE', #20394, #4947, #21576 ) ;
#14713=CARTESIAN_POINT ( 'NONE',  ( 6.312035131040564906, 19.41226734497195849, 13.00000000000000178 ) ) ;
#14716=DIRECTION ( 'NONE',  ( 1.000000000000000000, 0.000000000000000000, 0.000000000000000000 ) ) ;
#14720=CARTESIAN_POINT ( 'NONE',  ( 7.312035131040564906, 19.41226734497195849, 13.00000000000000178 ) ) ;
#14724=CARTESIAN_POINT ( 'NONE',  ( -8.559512017365658920, 19.71884705062586107, 13.00000000000000178 ) ) ;
#14732=CARTESIAN_POINT ( 'NONE',  ( 11.16520467992603294, 20.33931832809677331, 12.00000000000000000 ) ) ;
#14738=CARTESIAN_POINT ( 'NONE',  ( -1.265509184090266137, 8.754836972118123839, 12.00000000000000000 ) ) ;
#14741=CIRCLE ( 'NONE', #32929, 1.000000000000000000 ) ;
#14746=ORIENTED_EDGE ( 'NONE', *, *, #21554, .T. ) ;
#14749=LINE ( 'NONE', #11702, #8960 ) ;
#14758=EDGE_CURVE ( 'NONE', #761, #36183, #13817, .T. ) ;
#14763=ORIENTED_EDGE ( 'NONE', *, *, #8892, .F. ) ;
#14764=CARTESIAN_POINT ( 'NONE',  ( 6.953805871968278929, 30.22298757065274444, 6.000000000000000000 ) ) ;
#14765=CIRCLE ( 'NONE', #11519, 16.00000000000000000 ) ;
#14767=CARTESIAN_POINT ( 'NONE',  ( 4.440829913680675034, 10.60893893836775348, 12.00000000000000000 ) ) ;
#14776=DIRECTION ( 'NONE',  ( 0.000000000000000000, 0.000000000000000000, 1.000000000000000000 ) ) ;
#14787=ORIENTED_EDGE ( 'NONE', *, *, #7426, .T. ) ;
#14795=DIRECTION ( 'NONE',  ( 0.000000000000000000, 0.000000000000000000, 1.000000000000000000 ) ) ;
#14799=EDGE_CURVE ( 'NONE', #6629, #39920, #6846, .T. ) ;
#14802=ORIENTED_EDGE ( 'NONE', *, *, #30259, .T. ) ;
#14803=DIRECTION ( 'NONE',  ( 0.000000000000000000, 0.000000000000000000, 1.000000000000000000 ) ) ;
#14811=CARTESIAN_POINT ( 'NONE',  ( 11.78893975237933134, 23.27376113029817617, 6.000000000000000000 ) ) ;
#14813=CIRCLE ( 'NONE', #27168, 1.000000000000000888 ) ;
#14816=( LENGTH_UNIT ( ) NAMED_UNIT ( * ) SI_UNIT ( .MILLI., .METRE. ) );
#14819=AXIS2_PLACEMENT_3D ( 'NONE', #30849, #12352, #21697 ) ;
#14840=CYLINDRICAL_SURFACE ( 'NONE', #32245, 1.000000000000000888 ) ;
#14842=AXIS2_PLACEMENT_3D ( 'NONE', #32482, #4233, #7267 ) ;
#14845=ORIENTED_EDGE ( 'NONE', *, *, #27631, .F. ) ;
#14850=AXIS2_PLACEMENT_3D ( 'NONE', #39439, #36400, #5507 ) ;
#14854=ORIENTED_EDGE ( 'NONE', *, *, #9008, .F. ) ;
#14861=FACE_OUTER_BOUND ( 'NONE', #29110, .T. ) ;
#14868=EDGE_CURVE ( 'NONE', #4736, #25935, #13350, .T. ) ;
#14869=AXIS2_PLACEMENT_3D ( 'NONE', #8490, #33088, #36126 ) ;
#14876=AXIS2_PLACEMENT_3D ( 'NONE', #15010, #11372, #29648 ) ;
#14878=LINE ( 'NONE', #24015, #21362 ) ;
#14879=ORIENTED_EDGE ( 'NONE', *, *, #37893, .F. ) ;
#14892=EDGE_CURVE ( 'NONE', #36134, #13548, #13417, .T. ) ;
#14893=CARTESIAN_POINT ( 'NONE',  ( 13.64210930126480115, 24.20081211342298744, 13.00000000000000178 ) ) ;
#14907=CIRCLE ( 'NONE', #20739, 1.000000000000000888 ) ;
#14914=CARTESIAN_POINT ( 'NONE',  ( -14.26585111513660031, 17.86474508437623143, 12.00000000000000000 ) ) ;
#14916=CARTESIAN_POINT ( 'NONE',  ( -11.39464589777670867, 26.66807349098043289, 12.00000000000000000 ) ) ;
#14918=VERTEX_POINT ( 'NONE', #10985 ) ;
#14920=CYLINDRICAL_SURFACE ( 'NONE', #6007, 1.000000000000000000 ) ;
#14921=DIRECTION ( 'NONE',  ( 0.000000000000000000, 0.000000000000000000, 1.000000000000000000 ) ) ;
#14927=AXIS2_PLACEMENT_3D ( 'NONE', #23162, #7722, #32525 ) ;
#14947=DIRECTION ( 'NONE',  ( 1.000000000000000000, 0.000000000000000000, 0.000000000000000000 ) ) ;
#14954=DIRECTION ( 'NONE',  ( 0.000000000000000000, 0.000000000000000000, 1.000000000000000000 ) ) ;
#14959=AXIS2_PLACEMENT_3D ( 'NONE', #9967, #230, #16061 ) ;
#14961=CARTESIAN_POINT ( 'NONE',  ( 2.229431105722923245, 20.49260818092372460, 12.00000000000000000 ) ) ;
#14969=CARTESIAN_POINT ( 'NONE',  ( 9.183240348400453001, 28.21559575157615996, 13.00000000000000178 ) ) ;
#14973=ORIENTED_EDGE ( 'NONE', *, *, #30221, .F. ) ;
#14978=DIRECTION ( 'NONE',  ( 0.000000000000000000, 0.000000000000000000, 1.000000000000000000 ) ) ;
#14984=ORIENTED_EDGE ( 'NONE', *, *, #1529, .F. ) ;
#14985=CARTESIAN_POINT ( 'NONE',  ( 3.100636323082810009, 29.29593658752792962, 13.00000000000000178 ) ) ;
#14991=DIRECTION ( 'NONE',  ( 0.000000000000000000, 0.000000000000000000, 1.000000000000000000 ) ) ;
#15007=ORIENTED_EDGE ( 'NONE', *, *, #33226, .T. ) ;
#15010=CARTESIAN_POINT ( 'NONE',  ( -4.458872323573595864, 26.51478363815348160, 12.00000000000000000 ) ) ;
#15011=EDGE_LOOP ( 'NONE', ( #12225, #26376 ) ) ;
#15021=CARTESIAN_POINT ( 'NONE',  ( 0.01803229776516698107, 30.37627742347970283, 12.00000000000000000 ) ) ;
#15022=LINE ( 'NONE', #24366, #16231 ) ;
#15047=VERTEX_POINT ( 'NONE', #24169 ) ;
#15059=CARTESIAN_POINT ( 'NONE',  ( 7.953805871968279817, 30.22298757065274444, 12.00000000000000000 ) ) ;
#15069=CARTESIAN_POINT ( 'NONE',  ( 13.39463915635820790, 18.33192650902018883, 6.000000000000000000 ) ) ;
#15070=DIRECTION ( 'NONE',  ( 0.000000000000000000, 0.000000000000000000, 1.000000000000000000 ) ) ;
#15085=VERTEX_POINT ( 'NONE', #14985 ) ;
#15094=EDGE_CURVE ( 'NONE', #2814, #34302, #39363, .T. ) ;
#15108=CIRCLE ( 'NONE', #20305, 1.000000000000000000 ) ;
#15112=FACE_BOUND ( 'NONE', #9039, .T. ) ;
#15120=CARTESIAN_POINT ( 'NONE',  ( 12.41267482483262796, 26.20820393249957192, 6.000000000000000000 ) ) ;
#15126=AXIS2_PLACEMENT_3D ( 'NONE', #15927, #489, #28309 ) ;
#15144=CARTESIAN_POINT ( 'NONE',  ( -0.9819677022348329842, 30.37627742347970283, 12.00000000000000000 ) ) ;
#15146=CARTESIAN_POINT ( 'NONE',  ( -8.183247089818959097, 16.78440424842446532, 13.00000000000000178 ) ) ;
#15152=VECTOR ( 'NONE', #2769, 1000.000000000000000 ) ;
#15166=CARTESIAN_POINT ( 'NONE',  ( -4.082607396026893376, 23.58034083595207875, 12.00000000000000000 ) ) ;
#15167=CYLINDRICAL_SURFACE ( 'NONE', #19278, 1.000000000000000000 ) ;
#15168=CARTESIAN_POINT ( 'NONE',  ( -11.77091082532341204, 29.60251629318183575, 6.000000000000000000 ) ) ;
#15174=DIRECTION ( 'NONE',  ( 0.000000000000000000, 0.000000000000000000, 1.000000000000000000 ) ) ;
#15176=DIRECTION ( 'NONE',  ( 1.000000000000000000, 0.000000000000000000, 0.000000000000000000 ) ) ;
#15182=CARTESIAN_POINT ( 'NONE',  ( 6.935770203493858865, 22.34671014717335780, 6.000000000000000000 ) ) ;
#15195=AXIS2_PLACEMENT_3D ( 'NONE', #18217, #8866, #27550 ) ;
#15197=ORIENTED_EDGE ( 'NONE', *, *, #10260, .T. ) ;
#15200=CARTESIAN_POINT ( 'NONE',  ( -3.370709253380788084E-06, 22.50000000000031264, 6.000000000000000000 ) ) ;
#15203=CIRCLE ( 'NONE', #269, 1.000000000000000000 ) ;
#15206=DIRECTION ( 'NONE',  ( 1.000000000000000000, 0.000000000000000000, 0.000000000000000000 ) ) ;
#15207=ORIENTED_EDGE ( 'NONE', *, *, #25365, .F. ) ;
#15212=CIRCLE ( 'NONE', #37913, 1.000000000000000000 ) ;
#15234=VERTEX_POINT ( 'NONE', #30827 ) ;
#15243=LINE ( 'NONE', #34140, #10910 ) ;
#15244=VERTEX_POINT ( 'NONE', #3384 ) ;
#15252=ORIENTED_EDGE ( 'NONE', *, *, #11067, .F. ) ;
#15262=FACE_OUTER_BOUND ( 'NONE', #26843, .T. ) ;
#15266=CARTESIAN_POINT ( 'NONE',  ( 2.871201846650637268, 31.30332840660451765, 13.00000000000000178 ) ) ;
#15267=EDGE_CURVE ( 'NONE', #25818, #26036, #12926, .T. ) ;
#15274=AXIS2_PLACEMENT_3D ( 'NONE', #27503, #8822, #17579 ) ;
#15276=CIRCLE ( 'NONE', #1654, 1.000000000000000000 ) ;
#15292=CARTESIAN_POINT ( 'NONE',  ( -6.440836655099179353, 34.39106106163288246, 13.00000000000000178 ) ) ;
#15293=EDGE_LOOP ( 'NONE', ( #18350, #19141, #18742, #30036 ) ) ;
#15302=CIRCLE ( 'NONE', #17900, 1.000000000000000000 ) ;
#15305=CIRCLE ( 'NONE', #19860, 1.000000000000000000 ) ;
#15306=CYLINDRICAL_SURFACE ( 'NONE', #18733, 1.000000000000000000 ) ;
#15309=FACE_BOUND ( 'NONE', #38879, .T. ) ;
#15311=ORIENTED_EDGE ( 'NONE', *, *, #35900, .T. ) ;
#15314=FACE_OUTER_BOUND ( 'NONE', #22562, .T. ) ;
#15316=CARTESIAN_POINT ( 'NONE',  ( 14.01837422881150452, 21.26636931122159169, 12.00000000000000000 ) ) ;
#15327=AXIS2_PLACEMENT_3D ( 'NONE', #16033, #24975, #3636 ) ;
#15329=LINE ( 'NONE', #9236, #36745 ) ;
#15341=CARTESIAN_POINT ( 'NONE',  ( 0.000000000000000000, 22.50000000000000355, 12.00000000000000000 ) ) ;
#15345=EDGE_CURVE ( 'NONE', #9569, #12475, #1039, .T. ) ;
#15348=EDGE_CURVE ( 'NONE', #5069, #16796, #6226, .T. ) ;
#15352=CARTESIAN_POINT ( 'NONE',  ( -8.559512017365658920, 19.71884705062586107, 6.000000000000000000 ) ) ;
#15356=AXIS2_PLACEMENT_3D ( 'NONE', #305, #3544, #6582 ) ;
#15359=FACE_OUTER_BOUND ( 'NONE', #19257, .T. ) ;
#15362=DIRECTION ( 'NONE',  ( 1.000000000000000000, 0.000000000000000000, 0.000000000000000000 ) ) ;
#15363=CARTESIAN_POINT ( 'NONE',  ( 10.16520467992603294, 20.33931832809677331, 12.00000000000000000 ) ) ;
#15364=EDGE_CURVE ( 'NONE', #12341, #17253, #25680, .T. ) ;
#15366=DIRECTION ( 'NONE',  ( 1.000000000000000000, 0.000000000000000000, 0.000000000000000000 ) ) ;
#15374=LINE ( 'NONE', #34067, #19866 ) ;
#15391=VERTEX_POINT ( 'NONE', #34273 ) ;
#15394=VECTOR ( 'NONE', #3694, 1000.000000000000000 ) ;
#15397=ADVANCED_FACE ( 'NONE', ( #36924 ), #18437, .F. ) ;
#15399=CARTESIAN_POINT ( 'NONE',  ( 12.39463915635820612, 18.33192650902018883, 12.00000000000000000 ) ) ;
#15410=VERTEX_POINT ( 'NONE', #18636 ) ;
#15425=EDGE_CURVE ( 'NONE', #11093, #39968, #6234, .T. ) ;
#15439=EDGE_LOOP ( 'NONE', ( #29701, #13504 ) ) ;
#15443=CIRCLE ( 'NONE', #12195, 1.000000000000000000 ) ;
#15447=ORIENTED_EDGE ( 'NONE', *, *, #33004, .F. ) ;
#15450=EDGE_LOOP ( 'NONE', ( #13970, #17065, #34634, #3110 ) ) ;
#15452=EDGE_CURVE ( 'NONE', #36540, #29047, #4279, .T. ) ;
#15453=AXIS2_PLACEMENT_3D ( 'NONE', #27100, #5362, #2125 ) ;
#15466=EDGE_CURVE ( 'NONE', #15880, #14560, #6818, .T. ) ;
#15472=CIRCLE ( 'NONE', #39490, 1.000000000000000888 ) ;
#15480=EDGE_CURVE ( 'NONE', #36412, #24952, #22452, .T. ) ;
#15487=FACE_BOUND ( 'NONE', #921, .T. ) ;
#15493=VERTEX_POINT ( 'NONE', #16183 ) ;
#15495=FACE_OUTER_BOUND ( 'NONE', #19830, .T. ) ;
#15502=ADVANCED_FACE ( 'NONE', ( #38311 ), #19422, .F. ) ;
#15510=CIRCLE ( 'NONE', #28488, 1.000000000000000888 ) ;
#15511=AXIS2_PLACEMENT_3D ( 'NONE', #33073, #39939, #39350 ) ;
#15512=DIRECTION ( 'NONE',  ( 1.000000000000000000, 0.000000000000000000, 0.000000000000000000 ) ) ;
#15513=CARTESIAN_POINT ( 'NONE',  ( -3.326590493086956091, 6.849639119454676184, 12.00000000000000000 ) ) ;
#15516=FACE_BOUND ( 'NONE', #18899, .T. ) ;
#15519=LINE ( 'NONE', #24656, #36531 ) ;
#15528=DIRECTION ( 'NONE',  ( 1.000000000000000000, 0.000000000000000000, 0.000000000000000000 ) ) ;
#15530=ORIENTED_EDGE ( 'NONE', *, *, #38456, .F. ) ;
#15534=DIRECTION ( 'NONE',  ( 0.000000000000000000, 0.000000000000000000, 1.000000000000000000 ) ) ;
#15536=CARTESIAN_POINT ( 'NONE',  ( -13.64211604268330724, 20.79918788657763429, 13.00000000000000178 ) ) ;
#15537=EDGE_LOOP ( 'NONE', ( #6291, #17223, #2846, #33719 ) ) ;
#15542=ORIENTED_EDGE ( 'NONE', *, *, #8661, .T. ) ;
#15544=CARTESIAN_POINT ( 'NONE',  ( -6.688306800005769048, 28.52217545723006609, 12.00000000000000000 ) ) ;
#15564=CARTESIAN_POINT ( 'NONE',  ( -12.03641663870442713, 15.85735326529964873, 12.00000000000000000 ) ) ;
#15565=AXIS2_PLACEMENT_3D ( 'NONE', #18859, #12754, #19054 ) ;
#15570=LINE ( 'NONE', #16367, #32093 ) ;
#15578=CARTESIAN_POINT ( 'NONE',  ( -4.724378136954611840, 12.76962061027129458, 13.00000000000000178 ) ) ;
#15581=ORIENTED_EDGE ( 'NONE', *, *, #7795, .T. ) ;
#15592=ORIENTED_EDGE ( 'NONE', *, *, #23908, .F. ) ;
#15597=DIRECTION ( 'NONE',  ( 1.000000000000000000, 0.000000000000000000, 0.000000000000000000 ) ) ;
#15599=AXIS2_PLACEMENT_3D ( 'NONE', #20213, #23656, #33218 ) ;
#15604=EDGE_LOOP ( 'NONE', ( #4207, #23789 ) ) ;
#15607=CARTESIAN_POINT ( 'NONE',  ( -11.77091082532341204, 29.60251629318183575, 12.00000000000000000 ) ) ;
#15618=DIRECTION ( 'NONE',  ( 0.000000000000000000, 0.000000000000000000, 1.000000000000000000 ) ) ;
#15623=ADVANCED_FACE ( 'NONE', ( #35874 ), #1959, .F. ) ;
#15640=TOROIDAL_SURFACE ( 'NONE', #730, 16.00000000000000000, 1.000000000000000000 ) ;
#15649=CYLINDRICAL_SURFACE ( 'NONE', #24173, 1.000000000000000000 ) ;
#15652=VERTEX_POINT ( 'NONE', #14738 ) ;
#15660=EDGE_LOOP ( 'NONE', ( #38318, #12331 ) ) ;
#15662=DIRECTION ( 'NONE',  ( 1.000000000000000000, 0.000000000000000000, 0.000000000000000000 ) ) ;
#15666=CIRCLE ( 'NONE', #13713, 1.000000000000000000 ) ;
#15667=AXIS2_PLACEMENT_3D ( 'NONE', #1419, #35752, #17067 ) ;
#15675=CIRCLE ( 'NONE', #31887, 1.000000000000000000 ) ;
#15677=EDGE_LOOP ( 'NONE', ( #23777, #25902, #4848, #29332 ) ) ;
#15681=FACE_BOUND ( 'NONE', #14514, .T. ) ;
#15688=DIRECTION ( 'NONE',  ( 0.000000000000000000, 0.000000000000000000, 1.000000000000000000 ) ) ;
#15697=VERTEX_POINT ( 'NONE', #14333 ) ;
#15704=CYLINDRICAL_SURFACE ( 'NONE', #17573, 1.000000000000000000 ) ;
#15711=CARTESIAN_POINT ( 'NONE',  ( 2.494936919103933448, 34.23777120880591696, 6.000000000000000000 ) ) ;
#15715=ORIENTED_EDGE ( 'NONE', *, *, #22187, .F. ) ;
#15719=EDGE_CURVE ( 'NONE', #30551, #2500, #21161, .T. ) ;
#15720=EDGE_CURVE ( 'NONE', #10872, #38519, #26350, .T. ) ;
#15721=DIRECTION ( 'NONE',  ( 1.000000000000000000, 0.000000000000000000, 0.000000000000000000 ) ) ;
#15735=ORIENTED_EDGE ( 'NONE', *, *, #6027, .F. ) ;
#15740=DIRECTION ( 'NONE',  ( 0.000000000000000000, 0.000000000000000000, 1.000000000000000000 ) ) ;
#15741=VERTEX_POINT ( 'NONE', #33443 ) ;
#15751=VERTEX_POINT ( 'NONE', #17403 ) ;
#15753=AXIS2_PLACEMENT_3D ( 'NONE', #30764, #1031, #33622 ) ;
#15758=CARTESIAN_POINT ( 'NONE',  ( 0.000000000000000000, 22.50000000000000355, 13.00000000000000178 ) ) ;
#15759=AXIS2_PLACEMENT_3D ( 'NONE', #34023, #24469, #91 ) ;
#15760=LINE ( 'NONE', #9676, #31770 ) ;
#15762=DIRECTION ( 'NONE',  ( 0.000000000000000000, 0.000000000000000000, 1.000000000000000000 ) ) ;
#15766=VERTEX_POINT ( 'NONE', #20840 ) ;
#15772=ADVANCED_FACE ( 'NONE', ( #5584 ), #5389, .F. ) ;
#15779=AXIS2_PLACEMENT_3D ( 'NONE', #4575, #16976, #38092 ) ;
#15782=AXIS2_PLACEMENT_3D ( 'NONE', #6211, #22842, #10257 ) ;
#15792=CARTESIAN_POINT ( 'NONE',  ( -8.917741276437942233, 30.52956727630665057, 13.00000000000000178 ) ) ;
#15794=DIRECTION ( 'NONE',  ( 1.000000000000000000, 0.000000000000000000, 0.000000000000000000 ) ) ;
#15838=CYLINDRICAL_SURFACE ( 'NONE', #2408, 1.000000000000000000 ) ;
#15840=CIRCLE ( 'NONE', #11324, 1.000000000000000000 ) ;
#15842=VERTEX_POINT ( 'NONE', #37466 ) ;
#15849=CYLINDRICAL_SURFACE ( 'NONE', #16402, 1.000000000000000000 ) ;
#15856=FACE_OUTER_BOUND ( 'NONE', #39773, .T. ) ;
#15861=DIRECTION ( 'NONE',  ( 1.000000000000000000, 0.000000000000000000, 0.000000000000000000 ) ) ;
#15862=ORIENTED_EDGE ( 'NONE', *, *, #9034, .T. ) ;
#15863=DIRECTION ( 'NONE',  ( 1.000000000000000000, 0.000000000000000000, 0.000000000000000000 ) ) ;
#15880=VERTEX_POINT ( 'NONE', #27523 ) ;
#15885=FACE_BOUND ( 'NONE', #11003, .T. ) ;
#15886=AXIS2_PLACEMENT_3D ( 'NONE', #33520, #30464, #7053 ) ;
#15897=ORIENTED_EDGE ( 'NONE', *, *, #13603, .F. ) ;
#15912=FACE_BOUND ( 'NONE', #4755, .T. ) ;
#15915=DIRECTION ( 'NONE',  ( 1.000000000000000000, 0.000000000000000000, 0.000000000000000000 ) ) ;
#15922=EDGE_CURVE ( 'NONE', #697, #20919, #15329, .T. ) ;
#15926=EDGE_CURVE ( 'NONE', #31607, #6918, #11459, .T. ) ;
#15927=CARTESIAN_POINT ( 'NONE',  ( -5.706342468480190000, 20.64589803375067945, 6.000000000000000000 ) ) ;
#15932=DIRECTION ( 'NONE',  ( 1.000000000000000000, 0.000000000000000000, 0.000000000000000000 ) ) ;
#15933=ORIENTED_EDGE ( 'NONE', *, *, #186, .T. ) ;
#15940=DIRECTION ( 'NONE',  ( 1.000000000000000000, 0.000000000000000000, 0.000000000000000000 ) ) ;
#15953=DIRECTION ( 'NONE',  ( 1.000000000000000000, 0.000000000000000000, 0.000000000000000000 ) ) ;
#15959=DIRECTION ( 'NONE',  ( 0.000000000000000000, 0.000000000000000000, 1.000000000000000000 ) ) ;
#15961=CARTESIAN_POINT ( 'NONE',  ( 3.326583613081082635, 38.15036234293571482, 12.00000000000000000 ) ) ;
#15968=FACE_OUTER_BOUND ( 'NONE', #18142, .T. ) ;
#15969=CIRCLE ( 'NONE', #32840, 1.000000000000000000 ) ;
#15972=DIRECTION ( 'NONE',  ( 1.000000000000000000, 0.000000000000000000, 0.000000000000000000 ) ) ;
#15974=CIRCLE ( 'NONE', #30887, 1.000000000000000000 ) ;
#15975=EDGE_CURVE ( 'NONE', #37255, #19619, #17295, .T. ) ;
#15987=ADVANCED_FACE ( 'NONE', ( #34222 ), #36672, .F. ) ;
#15988=EDGE_LOOP ( 'NONE', ( #7186, #15715 ) ) ;
#16003=ORIENTED_EDGE ( 'NONE', *, *, #4197, .F. ) ;
#16025=ADVANCED_FACE ( 'NONE', ( #35421 ), #16328, .F. ) ;
#16027=CIRCLE ( 'NONE', #24441, 1.000000000000000000 ) ;
#16033=CARTESIAN_POINT ( 'NONE',  ( -0.3582326297815359162, 33.31072022568110924, 12.00000000000000000 ) ) ;
#16052=EDGE_CURVE ( 'NONE', #8090, #21833, #35496, .T. ) ;
#16054=AXIS2_PLACEMENT_3D ( 'NONE', #32595, #19789, #4754 ) ;
#16056=LINE ( 'NONE', #5910, #7086 ) ;
#16061=DIRECTION ( 'NONE',  ( 1.000000000000000000, 0.000000000000000000, 0.000000000000000000 ) ) ;
#16075=CARTESIAN_POINT ( 'NONE',  ( -2.476907992048017260, 18.63850621467409496, 6.000000000000000000 ) ) ;
#16081=FACE_BOUND ( 'NONE', #12191, .T. ) ;
#16083=AXIS2_PLACEMENT_3D ( 'NONE', #1555, #38521, #31823 ) ;
#16087=CARTESIAN_POINT ( 'NONE',  ( -14.64211604268330902, 20.79918788657763429, 13.00000000000000178 ) ) ;
#16090=DIRECTION ( 'NONE',  ( 0.000000000000000000, 0.000000000000000000, 1.000000000000000000 ) ) ;
#16095=EDGE_LOOP ( 'NONE', ( #20163, #23550 ) ) ;
#16106=DIRECTION ( 'NONE',  ( -0.000000000000000000, -0.000000000000000000, -1.000000000000000000 ) ) ;
#16107=CYLINDRICAL_SURFACE ( 'NONE', #36380, 1.000000000000000888 ) ;
#16116=EDGE_CURVE ( 'NONE', #1841, #17659, #9831, .T. ) ;
#16118=AXIS2_PLACEMENT_3D ( 'NONE', #2611, #14193, #32899 ) ;
#16127=DIRECTION ( 'NONE',  ( 1.000000000000000000, 0.000000000000000000, 0.000000000000000000 ) ) ;
#16132=CYLINDRICAL_SURFACE ( 'NONE', #3013, 1.000000000000000888 ) ;
#16136=DIRECTION ( 'NONE',  ( 1.000000000000000000, 0.000000000000000000, 0.000000000000000000 ) ) ;
#16138=ORIENTED_EDGE ( 'NONE', *, *, #15364, .F. ) ;
#16153=ORIENTED_EDGE ( 'NONE', *, *, #27265, .F. ) ;
#16157=CARTESIAN_POINT ( 'NONE',  ( 0.9819609608163288872, 14.62372257652092422, 12.00000000000000000 ) ) ;
#16162=CARTESIAN_POINT ( 'NONE',  ( 6.440829913680675034, 10.60893893836775348, 13.00000000000000178 ) ) ;
#16164=LINE ( 'NONE', #35252, #8263 ) ;
#16169=CYLINDRICAL_SURFACE ( 'NONE', #22362, 1.000000000000000000 ) ;
#16170=AXIS2_PLACEMENT_3D ( 'NONE', #36515, #8483, #8279 ) ;
#16178=ORIENTED_EDGE ( 'NONE', *, *, #39171, .F. ) ;
#16183=CARTESIAN_POINT ( 'NONE',  ( 3.229431105722923245, 20.49260818092372460, 13.00000000000000178 ) ) ;
#16191=CARTESIAN_POINT ( 'NONE',  ( 7.688300058587269170, 16.47782454277055564, 13.00000000000000178 ) ) ;
#16193=ORIENTED_EDGE ( 'NONE', *, *, #18070, .F. ) ;
#16224=LINE ( 'NONE', #1384, #32360 ) ;
#16230=LINE ( 'NONE', #13167, #34299 ) ;
#16231=VECTOR ( 'NONE', #2634, 1000.000000000000000 ) ;
#16241=CIRCLE ( 'NONE', #35702, 1.000000000000000888 ) ;
#16248=ORIENTED_EDGE ( 'NONE', *, *, #18782, .T. ) ;
#16253=ORIENTED_EDGE ( 'NONE', *, *, #31938, .T. ) ;
#16264=CIRCLE ( 'NONE', #29892, 1.000000000000000888 ) ;
#16268=ORIENTED_EDGE ( 'NONE', *, *, #6124, .T. ) ;
#16271=DIRECTION ( 'NONE',  ( 0.000000000000000000, 0.000000000000000000, 1.000000000000000000 ) ) ;
#16272=ORIENTED_EDGE ( 'NONE', *, *, #6603, .F. ) ;
#16278=ADVANCED_FACE ( 'NONE', ( #8396 ), #33190, .F. ) ;
#16294=ORIENTED_EDGE ( 'NONE', *, *, #21557, .T. ) ;
#16298=ORIENTED_EDGE ( 'NONE', *, *, #9015, .T. ) ;
#16310=FACE_BOUND ( 'NONE', #11883, .T. ) ;
#16325=EDGE_CURVE ( 'NONE', #6684, #35424, #22484, .T. ) ;
#16328=CYLINDRICAL_SURFACE ( 'NONE', #8867, 1.000000000000000000 ) ;
#16329=EDGE_CURVE ( 'NONE', #2814, #18344, #10843, .T. ) ;
#16332=EDGE_CURVE ( 'NONE', #697, #29252, #16027, .T. ) ;
#16334=VERTEX_POINT ( 'NONE', #23631 ) ;
#16347=EDGE_LOOP ( 'NONE', ( #5804, #39811, #21048, #13292 ) ) ;
#16352=EDGE_CURVE ( 'NONE', #1614, #2419, #20594, .T. ) ;
#16355=CYLINDRICAL_SURFACE ( 'NONE', #17173, 1.000000000000000888 ) ;
#16357=LINE ( 'NONE', #38084, #34595 ) ;
#16358=AXIS2_PLACEMENT_3D ( 'NONE', #32369, #26660, #17134 ) ;
#16360=VERTEX_POINT ( 'NONE', #20985 ) ;
#16362=FACE_OUTER_BOUND ( 'NONE', #36499, .T. ) ;
#16367=CARTESIAN_POINT ( 'NONE',  ( -5.064571727552472424, 31.45661825943146894, 6.000000000000000000 ) ) ;
#16368=ORIENTED_EDGE ( 'NONE', *, *, #17692, .F. ) ;
#16372=CIRCLE ( 'NONE', #30679, 1.000000000000000888 ) ;
#16388=ORIENTED_EDGE ( 'NONE', *, *, #30757, .T. ) ;
#16401=EDGE_LOOP ( 'NONE', ( #13826, #13742 ) ) ;
#16402=AXIS2_PLACEMENT_3D ( 'NONE', #25580, #22137, #25784 ) ;
#16408=ORIENTED_EDGE ( 'NONE', *, *, #38128, .T. ) ;
#16421=DIRECTION ( 'NONE',  ( 1.000000000000000000, 0.000000000000000000, 0.000000000000000000 ) ) ;
#16426=LINE ( 'NONE', #25761, #28397 ) ;
#16427=AXIS2_PLACEMENT_3D ( 'NONE', #16809, #13745, #4406 ) ;
#16433=AXIS2_PLACEMENT_3D ( 'NONE', #38261, #16735, #25452 ) ;
#16438=VECTOR ( 'NONE', #23464, 1000.000000000000000 ) ;
#16452=AXIS2_PLACEMENT_3D ( 'NONE', #33470, #36705, #27947 ) ;
#16453=VERTEX_POINT ( 'NONE', #11838 ) ;
#16456=CARTESIAN_POINT ( 'NONE',  ( 3.476901250629512941, 26.36149378532653031, 12.00000000000000000 ) ) ;
#16465=DIRECTION ( 'NONE',  ( 1.000000000000000000, 0.000000000000000000, 0.000000000000000000 ) ) ;
#16470=CIRCLE ( 'NONE', #39174, 1.000000000000000000 ) ;
#16471=ORIENTED_EDGE ( 'NONE', *, *, #30493, .F. ) ;
#16472=CARTESIAN_POINT ( 'NONE',  ( -11.77091082532341204, 29.60251629318183575, 13.00000000000000178 ) ) ;
#16483=ORIENTED_EDGE ( 'NONE', *, *, #28867, .F. ) ;
#16485=CARTESIAN_POINT ( 'NONE',  ( 2.229431105722923245, 20.49260818092372460, 13.00000000000000178 ) ) ;
#16487=FACE_BOUND ( 'NONE', #8452, .T. ) ;
#16491=EDGE_LOOP ( 'NONE', ( #5112, #10751 ) ) ;
#16492=CIRCLE ( 'NONE', #19002, 1.000000000000000888 ) ;
#16496=ADVANCED_FACE ( 'NONE', ( #24426 ), #8991, .F. ) ;
#16497=VERTEX_POINT ( 'NONE', #26375 ) ;
#16500=EDGE_LOOP ( 'NONE', ( #13037, #5830, #16664, #25233 ) ) ;
#16511=ADVANCED_FACE ( 'NONE', ( #38770 ), #17046, .F. ) ;
#16512=DIRECTION ( 'NONE',  ( 0.000000000000000000, 0.000000000000000000, 1.000000000000000000 ) ) ;
#16516=CARTESIAN_POINT ( 'NONE',  ( 4.211395437248501850, 12.61633075744433796, 12.00000000000000000 ) ) ;
#16522=VERTEX_POINT ( 'NONE', #13578 ) ;
#16523=AXIS2_PLACEMENT_3D ( 'NONE', #34155, #5715, #15662 ) ;
#16536=CARTESIAN_POINT ( 'NONE',  ( 3.458865582155095986, 18.48521636184714012, 6.000000000000000000 ) ) ;
#16542=ORIENTED_EDGE ( 'NONE', *, *, #21166, .F. ) ;
#16549=VECTOR ( 'NONE', #16689, 1000.000000000000000 ) ;
#16558=LINE ( 'NONE', #7195, #29081 ) ;
#16560=EDGE_CURVE ( 'NONE', #33408, #37025, #27055, .T. ) ;
#16563=CARTESIAN_POINT ( 'NONE',  ( 12.01837422881150275, 21.26636931122159169, 13.00000000000000178 ) ) ;
#16565=CYLINDRICAL_SURFACE ( 'NONE', #9784, 1.000000000000000888 ) ;
#16566=LINE ( 'NONE', #1938, #13583 ) ;
#16582=EDGE_LOOP ( 'NONE', ( #29837, #17138, #30579, #39397 ) ) ;
#16583=VECTOR ( 'NONE', #29566, 1000.000000000000000 ) ;
#16598=VERTEX_POINT ( 'NONE', #7274 ) ;
#16604=LINE ( 'NONE', #22681, #36221 ) ;
#16607=ORIENTED_EDGE ( 'NONE', *, *, #16800, .T. ) ;
#16609=DIRECTION ( 'NONE',  ( 0.000000000000000000, 0.000000000000000000, 1.000000000000000000 ) ) ;
#16613=EDGE_CURVE ( 'NONE', #33185, #22962, #14186, .T. ) ;
#16615=VECTOR ( 'NONE', #9491, 1000.000000000000000 ) ;
#16617=ORIENTED_EDGE ( 'NONE', *, *, #4457, .T. ) ;
#16619=CYLINDRICAL_SURFACE ( 'NONE', #36020, 1.000000000000000000 ) ;
#16620=VECTOR ( 'NONE', #23722, 1000.000000000000000 ) ;
#16635=CYLINDRICAL_SURFACE ( 'NONE', #14842, 1.000000000000000000 ) ;
#16647=AXIS2_PLACEMENT_3D ( 'NONE', #28312, #27918, #94 ) ;
#16653=ORIENTED_EDGE ( 'NONE', *, *, #38334, .F. ) ;
#16664=ORIENTED_EDGE ( 'NONE', *, *, #12942, .T. ) ;
#16665=( NAMED_UNIT ( * ) SI_UNIT ( $, .STERADIAN. ) SOLID_ANGLE_UNIT ( ) );
#16670=CARTESIAN_POINT ( 'NONE',  ( -0.3762682982559537037, 25.43444280220171194, 6.000000000000000000 ) ) ;
#16674=VECTOR ( 'NONE', #35021, 1000.000000000000000 ) ;
#16675=ORIENTED_EDGE ( 'NONE', *, *, #683, .T. ) ;
#16681=ORIENTED_EDGE ( 'NONE', *, *, #10390, .F. ) ;
#16689=DIRECTION ( 'NONE',  ( 0.000000000000000000, 0.000000000000000000, 1.000000000000000000 ) ) ;
#16690=FACE_BOUND ( 'NONE', #12948, .T. ) ;
#16695=CARTESIAN_POINT ( 'NONE',  ( -6.935776944912362296, 22.65328985282726393, 12.00000000000000000 ) ) ;
#16696=DIRECTION ( 'NONE',  ( 1.000000000000000000, 0.000000000000000000, 0.000000000000000000 ) ) ;
#16698=EDGE_LOOP ( 'NONE', ( #22109, #34809 ) ) ;
#16700=DIRECTION ( 'NONE',  ( 1.000000000000000000, 0.000000000000000000, 0.000000000000000000 ) ) ;
#16705=DIRECTION ( 'NONE',  ( 0.000000000000000000, 0.000000000000000000, 1.000000000000000000 ) ) ;
#16707=ORIENTED_EDGE ( 'NONE', *, *, #13854, .F. ) ;
#16714=FACE_OUTER_BOUND ( 'NONE', #26132, .T. ) ;
#16717=CYLINDRICAL_SURFACE ( 'NONE', #19086, 1.000000000000000000 ) ;
#16724=VERTEX_POINT ( 'NONE', #33296 ) ;
#16733=ORIENTED_EDGE ( 'NONE', *, *, #12085, .T. ) ;
#16735=DIRECTION ( 'NONE',  ( 0.000000000000000000, 0.000000000000000000, 1.000000000000000000 ) ) ;
#16742=AXIS2_PLACEMENT_3D ( 'NONE', #6387, #11901, #107 ) ;
#16767=FACE_OUTER_BOUND ( 'NONE', #17800, .T. ) ;
#16768=CARTESIAN_POINT ( 'NONE',  ( -1.229437847141422901, 24.50739181907689712, 12.00000000000000000 ) ) ;
#16780=DIRECTION ( 'NONE',  ( 0.000000000000000000, 0.000000000000000000, 1.000000000000000000 ) ) ;
#16784=ORIENTED_EDGE ( 'NONE', *, *, #10143, .F. ) ;
#16792=CIRCLE ( 'NONE', #39491, 1.000000000000000000 ) ;
#16796=VERTEX_POINT ( 'NONE', #21287 ) ;
#16800=EDGE_CURVE ( 'NONE', #37976, #37515, #29826, .T. ) ;
#16802=CIRCLE ( 'NONE', #27836, 1.000000000000000888 ) ;
#16803=ORIENTED_EDGE ( 'NONE', *, *, #23455, .F. ) ;
#16806=ORIENTED_EDGE ( 'NONE', *, *, #6027, .T. ) ;
#16809=CARTESIAN_POINT ( 'NONE',  ( 11.41267482483262619, 26.20820393249957192, 6.000000000000000000 ) ) ;
#16815=EDGE_CURVE ( 'NONE', #11229, #26705, #23732, .T. ) ;
#16818=ORIENTED_EDGE ( 'NONE', *, *, #12792, .F. ) ;
#16819=EDGE_CURVE ( 'NONE', #36134, #36348, #31585, .T. ) ;
#16830=ORIENTED_EDGE ( 'NONE', *, *, #14892, .T. ) ;
#16831=ADVANCED_FACE ( 'NONE', ( #39570 ), #24336, .F. ) ;
#16844=CARTESIAN_POINT ( 'NONE',  ( 10.16520467992603294, 20.33931832809677331, 6.000000000000000000 ) ) ;
#16867=DIRECTION ( 'NONE',  ( 1.000000000000000000, 0.000000000000000000, 0.000000000000000000 ) ) ;
#16872=ADVANCED_FACE ( 'NONE', ( #17658 ), #18247, .F. ) ;
#16875=CARTESIAN_POINT ( 'NONE',  ( 8.917734535019441466, 14.47043272369397116, 6.000000000000000000 ) ) ;
#16881=DIRECTION ( 'NONE',  ( 1.000000000000000000, 0.000000000000000000, 0.000000000000000000 ) ) ;
#16885=VECTOR ( 'NONE', #26351, 1000.000000000000000 ) ;
#16891=CARTESIAN_POINT ( 'NONE',  ( -3.100643064501314328, 15.70406341247269211, 6.000000000000000000 ) ) ;
#16892=ORIENTED_EDGE ( 'NONE', *, *, #3040, .T. ) ;
#16899=CYLINDRICAL_SURFACE ( 'NONE', #19555, 1.000000000000000000 ) ;
#16902=CARTESIAN_POINT ( 'NONE',  ( -11.16521142134453726, 24.66068167190384841, 12.00000000000000000 ) ) ;
#16905=ORIENTED_EDGE ( 'NONE', *, *, #22636, .F. ) ;
#16908=ORIENTED_EDGE ( 'NONE', *, *, #34833, .F. ) ;
#16910=CARTESIAN_POINT ( 'NONE',  ( -3.494943660522439099, 10.76222879119470832, 13.00000000000000178 ) ) ;
#16912=EDGE_LOOP ( 'NONE', ( #17812, #24668 ) ) ;
#16914=CIRCLE ( 'NONE', #1983, 1.000000000000000888 ) ;
#16918=DIRECTION ( 'NONE',  ( 1.000000000000000000, 0.000000000000000000, 0.000000000000000000 ) ) ;
#16921=LINE ( 'NONE', #10617, #13246 ) ;
#16926=CYLINDRICAL_SURFACE ( 'NONE', #26841, 1.000000000000000000 ) ;
#16938=EDGE_LOOP ( 'NONE', ( #3042, #28835 ) ) ;
#16942=DIRECTION ( 'NONE',  ( 1.000000000000000000, 0.000000000000000000, 0.000000000000000000 ) ) ;
#16946=CARTESIAN_POINT ( 'NONE',  ( -10.78894649379783388, 21.72623886970244911, 13.00000000000000178 ) ) ;
#16950=ADVANCED_FACE ( 'NONE', ( #36734 ), #24533, .F. ) ;
#16960=ORIENTED_EDGE ( 'NONE', *, *, #31843, .T. ) ;
#16965=CARTESIAN_POINT ( 'NONE',  ( 9.541469607472739867, 17.40487552589537401, 12.00000000000000000 ) ) ;
#16966=CARTESIAN_POINT ( 'NONE',  ( -8.917741276437942233, 30.52956727630665057, 12.00000000000000000 ) ) ;
#16976=DIRECTION ( 'NONE',  ( 0.000000000000000000, 0.000000000000000000, 1.000000000000000000 ) ) ;
#16978=CARTESIAN_POINT ( 'NONE',  ( 12.77090408390491305, 15.39748370681878775, 6.000000000000000000 ) ) ;
#16980=AXIS2_PLACEMENT_3D ( 'NONE', #4265, #7715, #14213 ) ;
#16985=CARTESIAN_POINT ( 'NONE',  ( -4.118678732975735279, 7.827785988993307242, 13.00000000000000178 ) ) ;
#16999=CARTESIAN_POINT ( 'NONE',  ( 1.871201846650637046, 31.30332840660451765, 12.00000000000000000 ) ) ;
#17001=FACE_OUTER_BOUND ( 'NONE', #33210, .T. ) ;
#17003=ORIENTED_EDGE ( 'NONE', *, *, #20230, .F. ) ;
#17015=DIRECTION ( 'NONE',  ( 1.000000000000000000, 0.000000000000000000, 0.000000000000000000 ) ) ;
#17017=FACE_OUTER_BOUND ( 'NONE', #36101, .T. ) ;
#17022=DIRECTION ( 'NONE',  ( 0.000000000000000000, 0.000000000000000000, 1.000000000000000000 ) ) ;
#17025=DIRECTION ( 'NONE',  ( 1.000000000000000000, 0.000000000000000000, 0.000000000000000000 ) ) ;
#17027=DIRECTION ( 'NONE',  ( 0.000000000000000000, 0.000000000000000000, 1.000000000000000000 ) ) ;
#17046=CYLINDRICAL_SURFACE ( 'NONE', #28990, 1.000000000000000888 ) ;
#17053=CARTESIAN_POINT ( 'NONE',  ( -0.3582326297815359162, 33.31072022568110924, 13.00000000000000178 ) ) ;
#17057=ORIENTED_EDGE ( 'NONE', *, *, #7889, .F. ) ;
#17062=EDGE_LOOP ( 'NONE', ( #19037, #27726 ) ) ;
#17065=ORIENTED_EDGE ( 'NONE', *, *, #1452, .T. ) ;
#17067=DIRECTION ( 'NONE',  ( 1.000000000000000000, 0.000000000000000000, 0.000000000000000000 ) ) ;
#17074=ADVANCED_FACE ( 'NONE', ( #12539 ), #18445, .F. ) ;
#17075=DIRECTION ( 'NONE',  ( 1.000000000000000000, 0.000000000000000000, 0.000000000000000000 ) ) ;
#17076=EDGE_CURVE ( 'NONE', #2950, #31370, #34675, .T. ) ;
#17078=AXIS2_PLACEMENT_3D ( 'NONE', #39399, #11580, #36363 ) ;
#17080=ORIENTED_EDGE ( 'NONE', *, *, #2442, .T. ) ;
#17081=LINE ( 'NONE', #1234, #28738 ) ;
#17087=VERTEX_POINT ( 'NONE', #16191 ) ;
#17092=CARTESIAN_POINT ( 'NONE',  ( 0.2474667741973399226, 28.36888560440311480, 12.00000000000000000 ) ) ;
#17099=FACE_BOUND ( 'NONE', #34930, .T. ) ;
#17104=EDGE_CURVE ( 'NONE', #31085, #26783, #6436, .T. ) ;
#17113=CIRCLE ( 'NONE', #39133, 1.000000000000000000 ) ;
#17116=ORIENTED_EDGE ( 'NONE', *, *, #20058, .T. ) ;
#17122=CIRCLE ( 'NONE', #13858, 1.000000000000000888 ) ;
#17125=DIRECTION ( 'NONE',  ( 1.000000000000000000, 0.000000000000000000, 0.000000000000000000 ) ) ;
#17134=DIRECTION ( 'NONE',  ( 1.000000000000000000, 0.000000000000000000, 0.000000000000000000 ) ) ;
#17135=CARTESIAN_POINT ( 'NONE',  ( -9.294006203984645609, 33.46401007850805343, 6.000000000000000000 ) ) ;
#17138=ORIENTED_EDGE ( 'NONE', *, *, #32251, .F. ) ;
#17143=EDGE_LOOP ( 'NONE', ( #32402, #369, #27199, #4943 ) ) ;
#17151=AXIS2_PLACEMENT_3D ( 'NONE', #36305, #14360, #36897 ) ;
#17160=FACE_OUTER_BOUND ( 'NONE', #14403, .T. ) ;
#17167=ORIENTED_EDGE ( 'NONE', *, *, #4437, .T. ) ;
#17171=CARTESIAN_POINT ( 'NONE',  ( 1.623731701744046241, 25.43444280220171194, 12.00000000000000000 ) ) ;
#17173=AXIS2_PLACEMENT_3D ( 'NONE', #20571, #29149, #32965 ) ;
#17174=FACE_OUTER_BOUND ( 'NONE', #10217, .T. ) ;
#17175=CARTESIAN_POINT ( 'NONE',  ( 14.64210930126480115, 24.20081211342298744, 12.00000000000000000 ) ) ;
#17195=ORIENTED_EDGE ( 'NONE', *, *, #9642, .F. ) ;
#17207=CARTESIAN_POINT ( 'NONE',  ( 8.935770203493859754, 22.34671014717335780, 13.00000000000000178 ) ) ;
#17215=EDGE_CURVE ( 'NONE', #27796, #24757, #33617, .T. ) ;
#17223=ORIENTED_EDGE ( 'NONE', *, *, #28496, .F. ) ;
#17227=CARTESIAN_POINT ( 'NONE',  ( -2.118678732975735279, 7.827785988993307242, 13.00000000000000178 ) ) ;
#17230=PRODUCT_DEFINITION ( 'UNKNOWN', '', #6074, #36631 ) ;
#17234=CARTESIAN_POINT ( 'NONE',  ( 11.77090408390491305, 15.39748370681878775, 6.000000000000000000 ) ) ;
#17240=EDGE_CURVE ( 'NONE', #3455, #12932, #24495, .T. ) ;
#17247=CARTESIAN_POINT ( 'NONE',  ( -3.476907992048017260, 18.63850621467409496, 13.00000000000000178 ) ) ;
#17253=VERTEX_POINT ( 'NONE', #26334 ) ;
#17256=DIRECTION ( 'NONE',  ( 1.000000000000000000, 0.000000000000000000, 0.000000000000000000 ) ) ;
#17258=DIRECTION ( 'NONE',  ( 0.000000000000000000, 0.000000000000000000, 1.000000000000000000 ) ) ;
#17263=AXIS2_PLACEMENT_3D ( 'NONE', #25410, #6715, #28266 ) ;
#17270=ORIENTED_EDGE ( 'NONE', *, *, #2196, .F. ) ;
#17272=CARTESIAN_POINT ( 'NONE',  ( 1.494936919103933226, 34.23777120880591696, 13.00000000000000178 ) ) ;
#17273=ORIENTED_EDGE ( 'NONE', *, *, #24715, .T. ) ;
#17288=FACE_OUTER_BOUND ( 'NONE', #31417, .T. ) ;
#17291=VECTOR ( 'NONE', #34767, 1000.000000000000000 ) ;
#17293=ORIENTED_EDGE ( 'NONE', *, *, #38456, .T. ) ;
#17295=CIRCLE ( 'NONE', #16647, 1.000000000000000000 ) ;
#17299=ORIENTED_EDGE ( 'NONE', *, *, #29729, .T. ) ;
#17308=CARTESIAN_POINT ( 'NONE',  ( 3.118671991557230516, 37.17221401100731981, 6.000000000000000000 ) ) ;
#17309=DIRECTION ( 'NONE',  ( 0.000000000000000000, 0.000000000000000000, 1.000000000000000000 ) ) ;
#17314=ORIENTED_EDGE ( 'NONE', *, *, #13603, .T. ) ;
#17323=CIRCLE ( 'NONE', #40001, 1.000000000000000888 ) ;
#17325=CARTESIAN_POINT ( 'NONE',  ( 13.01837422881150452, 21.26636931122159169, 13.00000000000000178 ) ) ;
#17327=DIRECTION ( 'NONE',  ( 0.000000000000000000, 0.000000000000000000, 1.000000000000000000 ) ) ;
#17330=CARTESIAN_POINT ( 'NONE',  ( -6.064571727552472424, 31.45661825943146894, 6.000000000000000000 ) ) ;
#17331=EDGE_CURVE ( 'NONE', #34177, #18996, #5703, .T. ) ;
#17345=ORIENTED_EDGE ( 'NONE', *, *, #12296, .T. ) ;
#17363=EDGE_CURVE ( 'NONE', #21424, #14474, #1798, .T. ) ;
#17371=ORIENTED_EDGE ( 'NONE', *, *, #16819, .F. ) ;
#17376=EDGE_CURVE ( 'NONE', #7792, #28710, #11503, .T. ) ;
#17377=CIRCLE ( 'NONE', #37454, 1.000000000000000000 ) ;
#17382=LINE ( 'NONE', #30159, #36692 ) ;
#17388=CIRCLE ( 'NONE', #27747, 1.000000000000000888 ) ;
#17389=DIRECTION ( 'NONE',  ( 0.000000000000000000, 0.000000000000000000, 1.000000000000000000 ) ) ;
#17393=EDGE_LOOP ( 'NONE', ( #10103, #5172, #9594, #31794 ) ) ;
#17403=CARTESIAN_POINT ( 'NONE',  ( -10.18324708981896087, 16.78440424842446532, 12.00000000000000000 ) ) ;
#17409=VERTEX_POINT ( 'NONE', #23687 ) ;
#17413=CYLINDRICAL_SURFACE ( 'NONE', #28387, 1.000000000000000000 ) ;
#17420=CYLINDRICAL_SURFACE ( 'NONE', #29100, 1.000000000000000000 ) ;
#17421=EDGE_CURVE ( 'NONE', #27843, #3881, #8854, .T. ) ;
#17425=VECTOR ( 'NONE', #28830, 1000.000000000000000 ) ;
#17431=CYLINDRICAL_SURFACE ( 'NONE', #37951, 1.000000000000000888 ) ;
#17433=DIRECTION ( 'NONE',  ( 1.000000000000000000, 0.000000000000000000, 0.000000000000000000 ) ) ;
#17438=DIRECTION ( 'NONE',  ( 0.000000000000000000, 0.000000000000000000, 1.000000000000000000 ) ) ;
#17447=AXIS2_PLACEMENT_3D ( 'NONE', #2617, #18064, #15206 ) ;
#17449=DIRECTION ( 'NONE',  ( 0.000000000000000000, 0.000000000000000000, 1.000000000000000000 ) ) ;
#17450=CIRCLE ( 'NONE', #26413, 1.000000000000000888 ) ;
#17458=ORIENTED_EDGE ( 'NONE', *, *, #18958, .F. ) ;
#17461=CARTESIAN_POINT ( 'NONE',  ( 0.2474667741973399226, 28.36888560440311480, 6.000000000000000000 ) ) ;
#17463=CARTESIAN_POINT ( 'NONE',  ( -6.082607396026893376, 23.58034083595207875, 6.000000000000000000 ) ) ;
#17464=ORIENTED_EDGE ( 'NONE', *, *, #22636, .T. ) ;
#17468=CIRCLE ( 'NONE', #11598, 1.000000000000000000 ) ;
#17473=VERTEX_POINT ( 'NONE', #38928 ) ;
#17479=ORIENTED_EDGE ( 'NONE', *, *, #10548, .F. ) ;
#17485=EDGE_LOOP ( 'NONE', ( #27333, #26528, #33116, #3006 ) ) ;
#17486=CYLINDRICAL_SURFACE ( 'NONE', #18375, 1.000000000000000888 ) ;
#17489=EDGE_CURVE ( 'NONE', #14625, #26936, #40059, .T. ) ;
#17491=DIRECTION ( 'NONE',  ( 1.000000000000000000, 0.000000000000000000, 0.000000000000000000 ) ) ;
#17501=AXIS2_PLACEMENT_3D ( 'NONE', #35145, #29251, #7298 ) ;
#17504=DIRECTION ( 'NONE',  ( 1.000000000000000000, 0.000000000000000000, 0.000000000000000000 ) ) ;
#17506=FACE_OUTER_BOUND ( 'NONE', #34242, .T. ) ;
#17511=CARTESIAN_POINT ( 'NONE',  ( 7.330070799514983193, 27.28854476845134513, 13.00000000000000178 ) ) ;
#17512=VERTEX_POINT ( 'NONE', #8454 ) ;
#17516=ORIENTED_EDGE ( 'NONE', *, *, #73, .F. ) ;
#17519=ORIENTED_EDGE ( 'NONE', *, *, #19699, .F. ) ;
#17533=EDGE_CURVE ( 'NONE', #36946, #12832, #14749, .T. ) ;
#17537=DIRECTION ( 'NONE',  ( 0.000000000000000000, 0.000000000000000000, 1.000000000000000000 ) ) ;
#17545=ORIENTED_EDGE ( 'NONE', *, *, #31114, .F. ) ;
#17549=DIRECTION ( 'NONE',  ( 0.000000000000000000, 0.000000000000000000, 1.000000000000000000 ) ) ;
#17553=EDGE_LOOP ( 'NONE', ( #3326, #33541, #28433, #31644 ) ) ;
#17560=DIRECTION ( 'NONE',  ( 1.000000000000000000, 0.000000000000000000, 0.000000000000000000 ) ) ;
#17568=ORIENTED_EDGE ( 'NONE', *, *, #370, .T. ) ;
#17573=AXIS2_PLACEMENT_3D ( 'NONE', #10209, #22592, #1072 ) ;
#17579=DIRECTION ( 'NONE',  ( 1.000000000000000000, 0.000000000000000000, 0.000000000000000000 ) ) ;
#17587=EDGE_CURVE ( 'NONE', #10001, #25752, #35549, .T. ) ;
#17589=DIRECTION ( 'NONE',  ( 0.000000000000000000, 0.000000000000000000, 1.000000000000000000 ) ) ;
#17596=CARTESIAN_POINT ( 'NONE',  ( 2.587660364795204782, 9.681887955242936883, 12.00000000000000000 ) ) ;
#17605=VECTOR ( 'NONE', #38847, 1000.000000000000000 ) ;
#17608=DIRECTION ( 'NONE',  ( 1.000000000000000000, 0.000000000000000000, 0.000000000000000000 ) ) ;
#17620=EDGE_CURVE ( 'NONE', #2436, #9639, #5039, .T. ) ;
#17621=DIRECTION ( 'NONE',  ( 1.000000000000000000, 0.000000000000000000, 0.000000000000000000 ) ) ;
#17628=ORIENTED_EDGE ( 'NONE', *, *, #468, .F. ) ;
#17629=DIRECTION ( 'NONE',  ( 0.000000000000000000, 0.000000000000000000, 1.000000000000000000 ) ) ;
#17630=AXIS2_PLACEMENT_3D ( 'NONE', #16875, #26400, #29254 ) ;
#17631=DIRECTION ( 'NONE',  ( 0.000000000000000000, 0.000000000000000000, 1.000000000000000000 ) ) ;
#17636=CARTESIAN_POINT ( 'NONE',  ( 11.41267482483262619, 26.20820393249957192, 13.00000000000000178 ) ) ;
#17648=CIRCLE ( 'NONE', #9184, 1.000000000000000888 ) ;
#17658=FACE_OUTER_BOUND ( 'NONE', #9971, .T. ) ;
#17659=VERTEX_POINT ( 'NONE', #21632 ) ;
#17661=ORIENTED_EDGE ( 'NONE', *, *, #17240, .T. ) ;
#17664=ORIENTED_EDGE ( 'NONE', *, *, #12103, .T. ) ;
#17665=EDGE_CURVE ( 'NONE', #25752, #34344, #6193, .T. ) ;
#17667=CARTESIAN_POINT ( 'NONE',  ( 11.14716901145161643, 12.46304090461738667, 12.00000000000000000 ) ) ;
#17668=VERTEX_POINT ( 'NONE', #105 ) ;
#17670=ORIENTED_EDGE ( 'NONE', *, *, #31486, .T. ) ;
#17675=VERTEX_POINT ( 'NONE', #24881 ) ;
#17680=ORIENTED_EDGE ( 'NONE', *, *, #1376, .F. ) ;
#17682=DIRECTION ( 'NONE',  ( 1.000000000000000000, 0.000000000000000000, 0.000000000000000000 ) ) ;
#17690=AXIS2_PLACEMENT_3D ( 'NONE', #22197, #31351, #34799 ) ;
#17692=EDGE_CURVE ( 'NONE', #18996, #34177, #27104, .T. ) ;
#17694=DIRECTION ( 'NONE',  ( 0.000000000000000000, 0.000000000000000000, 1.000000000000000000 ) ) ;
#17706=CIRCLE ( 'NONE', #8615, 1.000000000000000000 ) ;
#17711=DIRECTION ( 'NONE',  ( 1.000000000000000000, 0.000000000000000000, 0.000000000000000000 ) ) ;
#17716=ORIENTED_EDGE ( 'NONE', *, *, #17331, .F. ) ;
#17728=CARTESIAN_POINT ( 'NONE',  ( 11.77090408390491305, 15.39748370681878775, 12.00000000000000000 ) ) ;
#17729=CIRCLE ( 'NONE', #28744, 1.000000000000000000 ) ;
#17732=AXIS2_PLACEMENT_3D ( 'NONE', #14724, #32822, #20628 ) ;
#17735=EDGE_CURVE ( 'NONE', #8022, #25824, #7646, .T. ) ;
#17743=VERTEX_POINT ( 'NONE', #28524 ) ;
#17752=ORIENTED_EDGE ( 'NONE', *, *, #23913, .T. ) ;
#17766=ORIENTED_EDGE ( 'NONE', *, *, #27780, .T. ) ;
#17775=ADVANCED_FACE ( 'NONE', ( #4549 ), #35033, .F. ) ;
#17779=DIRECTION ( 'NONE',  ( 0.000000000000000000, 0.000000000000000000, 1.000000000000000000 ) ) ;
#17781=VECTOR ( 'NONE', #34701, 1000.000000000000000 ) ;
#17782=DIRECTION ( 'NONE',  ( 0.000000000000000000, 0.000000000000000000, 1.000000000000000000 ) ) ;
#17784=VERTEX_POINT ( 'NONE', #19996 ) ;
#17787=DIRECTION ( 'NONE',  ( 0.000000000000000000, 0.000000000000000000, 1.000000000000000000 ) ) ;
#17790=DIRECTION ( 'NONE',  ( 0.000000000000000000, 0.000000000000000000, 1.000000000000000000 ) ) ;
#17795=AXIS2_PLACEMENT_3D ( 'NONE', #38387, #22943, #7502 ) ;
#17800=EDGE_LOOP ( 'NONE', ( #5141, #6057, #13785, #16294 ) ) ;
#17804=CARTESIAN_POINT ( 'NONE',  ( 5.082600654608392610, 21.41965916404854298, 6.000000000000000000 ) ) ;
#17806=LINE ( 'NONE', #39716, #32127 ) ;
#17812=ORIENTED_EDGE ( 'NONE', *, *, #28935, .F. ) ;
#17817=EDGE_LOOP ( 'NONE', ( #3003, #34780 ) ) ;
#17821=DIRECTION ( 'NONE',  ( 0.000000000000000000, 0.000000000000000000, 1.000000000000000000 ) ) ;
#17824=EDGE_CURVE ( 'NONE', #39968, #28710, #19327, .T. ) ;
#17831=CARTESIAN_POINT ( 'NONE',  ( 8.183240348400453001, 28.21559575157615996, 12.00000000000000000 ) ) ;
#17836=EDGE_CURVE ( 'NONE', #1261, #12491, #26500, .T. ) ;
#17838=AXIS2_PLACEMENT_3D ( 'NONE', #11780, #2836, #12177 ) ;
#17845=EDGE_CURVE ( 'NONE', #13470, #2072, #31029, .T. ) ;
#17868=AXIS2_PLACEMENT_3D ( 'NONE', #8542, #10999, #23383 ) ;
#17871=ORIENTED_EDGE ( 'NONE', *, *, #37588, .T. ) ;
#17872=CARTESIAN_POINT ( 'NONE',  ( -3.724378136954612284, 12.76962061027129458, 6.000000000000000000 ) ) ;
#17875=AXIS2_PLACEMENT_3D ( 'NONE', #28918, #8190, #16942 ) ;
#17877=ORIENTED_EDGE ( 'NONE', *, *, #34223, .T. ) ;
#17885=ORIENTED_EDGE ( 'NONE', *, *, #16800, .F. ) ;
#17891=FACE_OUTER_BOUND ( 'NONE', #5490, .T. ) ;
#17898=ORIENTED_EDGE ( 'NONE', *, *, #7631, .T. ) ;
#17900=AXIS2_PLACEMENT_3D ( 'NONE', #11881, #36666, #8836 ) ;
#17902=CARTESIAN_POINT ( 'NONE',  ( 3.326583613081083968, 38.15036234293572193, 13.00000000000000178 ) ) ;
#17905=ORIENTED_EDGE ( 'NONE', *, *, #6024, .T. ) ;
#17907=CARTESIAN_POINT ( 'NONE',  ( -6.348113209407908464, 9.835177808069893501, 13.00000000000000178 ) ) ;
#17919=CARTESIAN_POINT ( 'NONE',  ( 6.348106467989403257, 35.16482219193073178, 13.00000000000000178 ) ) ;
#17921=CARTESIAN_POINT ( 'NONE',  ( -15.26585111513660209, 17.86474508437623143, 13.00000000000000178 ) ) ;
#17922=ORIENTED_EDGE ( 'NONE', *, *, #10295, .F. ) ;
#17935=DIRECTION ( 'NONE',  ( 0.000000000000000000, 0.000000000000000000, 1.000000000000000000 ) ) ;
#17943=ORIENTED_EDGE ( 'NONE', *, *, #11789, .T. ) ;
#17947=DIRECTION ( 'NONE',  ( 0.000000000000000000, 0.000000000000000000, 1.000000000000000000 ) ) ;
#17958=VERTEX_POINT ( 'NONE', #29131 ) ;
#17968=DIRECTION ( 'NONE',  ( 0.000000000000000000, 0.000000000000000000, 1.000000000000000000 ) ) ;
#17973=CARTESIAN_POINT ( 'NONE',  ( -8.917741276437942233, 30.52956727630665057, 6.000000000000000000 ) ) ;
#17980=DIRECTION ( 'NONE',  ( 0.000000000000000000, 0.000000000000000000, 1.000000000000000000 ) ) ;
#17982=CIRCLE ( 'NONE', #29630, 2.000000000000000000 ) ;
#17984=ORIENTED_EDGE ( 'NONE', *, *, #25674, .T. ) ;
#17988=ADVANCED_FACE ( 'NONE', ( #17160 ), #27289, .F. ) ;
#18021=AXIS2_PLACEMENT_3D ( 'NONE', #39329, #23889, #36293 ) ;
#18029=CARTESIAN_POINT ( 'NONE',  ( -11.89031881743725982, 33.20608791387860492, 12.00000000000000000 ) ) ;
#18035=DIRECTION ( 'NONE',  ( 0.000000000000000000, 0.000000000000000000, 1.000000000000000000 ) ) ;
#18036=DIRECTION ( 'NONE',  ( 0.000000000000000000, 0.000000000000000000, 1.000000000000000000 ) ) ;
#18041=EDGE_LOOP ( 'NONE', ( #13928, #31914, #27040, #13953 ) ) ;
#18052=CIRCLE ( 'NONE', #10917, 1.000000000000000000 ) ;
#18056=ORIENTED_EDGE ( 'NONE', *, *, #21043, .F. ) ;
#18060=EDGE_CURVE ( 'NONE', #7748, #2515, #24527, .T. ) ;
#18062=EDGE_CURVE ( 'NONE', #8408, #36861, #29717, .T. ) ;
#18064=DIRECTION ( 'NONE',  ( 0.000000000000000000, 0.000000000000000000, 1.000000000000000000 ) ) ;
#18067=LINE ( 'NONE', #14811, #9759 ) ;
#18069=AXIS2_PLACEMENT_3D ( 'NONE', #28723, #10851, #7385 ) ;
#18070=EDGE_CURVE ( 'NONE', #12849, #15047, #14493, .T. ) ;
#18075=VECTOR ( 'NONE', #32812, 1000.000000000000000 ) ;
#18083=CARTESIAN_POINT ( 'NONE',  ( 0.000000000000000000, 22.50000000000000355, 6.000000000000000000 ) ) ;
#18084=CARTESIAN_POINT ( 'NONE',  ( 2.853166178176219425, 23.42705098312512746, 12.00000000000000000 ) ) ;
#18086=DIRECTION ( 'NONE',  ( 0.000000000000000000, 0.000000000000000000, 1.000000000000000000 ) ) ;
#18090=ADVANCED_FACE ( 'NONE', ( #39674 ), #11849, .F. ) ;
#18095=ORIENTED_EDGE ( 'NONE', *, *, #32309, .F. ) ;
#18101=CIRCLE ( 'NONE', #7704, 1.000000000000000888 ) ;
#18106=DIRECTION ( 'NONE',  ( 0.000000000000000000, 0.000000000000000000, 1.000000000000000000 ) ) ;
#18121=CARTESIAN_POINT ( 'NONE',  ( 2.211395437248501850, 12.61633075744433796, 13.00000000000000178 ) ) ;
#18122=ORIENTED_EDGE ( 'NONE', *, *, #13451, .T. ) ;
#18124=DIRECTION ( 'NONE',  ( 0.000000000000000000, 0.000000000000000000, 1.000000000000000000 ) ) ;
#18132=CARTESIAN_POINT ( 'NONE',  ( -14.01838097023000707, 23.73363068877903359, 6.000000000000000000 ) ) ;
#18140=CARTESIAN_POINT ( 'NONE',  ( -13.39464589777671044, 26.66807349098043289, 12.00000000000000000 ) ) ;
#18142=EDGE_LOOP ( 'NONE', ( #26872, #32755, #17898, #29919 ) ) ;
#18156=DIRECTION ( 'NONE',  ( 0.000000000000000000, 0.000000000000000000, 1.000000000000000000 ) ) ;
#18170=DIRECTION ( 'NONE',  ( 1.000000000000000000, 0.000000000000000000, 0.000000000000000000 ) ) ;
#18174=DIRECTION ( 'NONE',  ( 0.000000000000000000, 0.000000000000000000, 1.000000000000000000 ) ) ;
#18180=CIRCLE ( 'NONE', #25296, 1.000000000000000888 ) ;
#18187=ORIENTED_EDGE ( 'NONE', *, *, #23839, .F. ) ;
#18190=ORIENTED_EDGE ( 'NONE', *, *, #26670, .F. ) ;
#18200=ORIENTED_EDGE ( 'NONE', *, *, #27265, .T. ) ;
#18203=CARTESIAN_POINT ( 'NONE',  ( -10.80698216227225394, 13.84996144622306247, 12.00000000000000000 ) ) ;
#18209=CARTESIAN_POINT ( 'NONE',  ( 0.000000000000000000, 22.50000000000000355, 13.00000000000000178 ) ) ;
#18216=AXIS2_PLACEMENT_3D ( 'NONE', #26401, #22952, #17075 ) ;
#18217=CARTESIAN_POINT ( 'NONE',  ( -5.348113209407908464, 9.835177808069893501, 6.000000000000000000 ) ) ;
#18221=DIRECTION ( 'NONE',  ( 1.000000000000000000, 0.000000000000000000, 0.000000000000000000 ) ) ;
#18228=CARTESIAN_POINT ( 'NONE',  ( -4.458872323573595864, 26.51478363815348160, 12.00000000000000000 ) ) ;
#18238=ORIENTED_EDGE ( 'NONE', *, *, #8552, .F. ) ;
#18247=CYLINDRICAL_SURFACE ( 'NONE', #10200, 1.000000000000000000 ) ;
#18249=AXIS2_PLACEMENT_3D ( 'NONE', #37945, #29000, #22494 ) ;
#18256=DIRECTION ( 'NONE',  ( 1.000000000000000000, 0.000000000000000000, 0.000000000000000000 ) ) ;
#18261=ORIENTED_EDGE ( 'NONE', *, *, #6760, .T. ) ;
#18265=EDGE_CURVE ( 'NONE', #29319, #20641, #37424, .T. ) ;
#18269=ORIENTED_EDGE ( 'NONE', *, *, #38920, .F. ) ;
#18281=CARTESIAN_POINT ( 'NONE',  ( -9.541476348891238857, 27.59512447410525127, 12.00000000000000000 ) ) ;
#18283=ADVANCED_FACE ( 'NONE', ( #15495 ), #6533, .F. ) ;
#18307=ORIENTED_EDGE ( 'NONE', *, *, #28043, .T. ) ;
#18324=EDGE_CURVE ( 'NONE', #19863, #26705, #14813, .T. ) ;
#18332=ORIENTED_EDGE ( 'NONE', *, *, #6024, .F. ) ;
#18333=ORIENTED_EDGE ( 'NONE', *, *, #39580, .T. ) ;
#18342=AXIS2_PLACEMENT_3D ( 'NONE', #26051, #6557, #9820 ) ;
#18344=VERTEX_POINT ( 'NONE', #16902 ) ;
#18350=ORIENTED_EDGE ( 'NONE', *, *, #14599, .F. ) ;
#18357=ADVANCED_FACE ( 'NONE', ( #28674 ), #7133, .F. ) ;
#18362=DIRECTION ( 'NONE',  ( 1.000000000000000000, 0.000000000000000000, 0.000000000000000000 ) ) ;
#18364=FACE_BOUND ( 'NONE', #24470, .T. ) ;
#18370=FACE_BOUND ( 'NONE', #35596, .T. ) ;
#18375=AXIS2_PLACEMENT_3D ( 'NONE', #35359, #35964, #7721 ) ;
#18379=EDGE_CURVE ( 'NONE', #12836, #38979, #6926, .T. ) ;
#18400=VERTEX_POINT ( 'NONE', #16695 ) ;
#18409=DIRECTION ( 'NONE',  ( 0.000000000000000000, 0.000000000000000000, 1.000000000000000000 ) ) ;
#18410=COLOUR_RGB ( '', 0.40784314, 0.44705882, 0.49803922) ;
#18414=CIRCLE ( 'NONE', #22955, 1.000000000000000888 ) ;
#18415=DIRECTION ( 'NONE',  ( 0.000000000000000000, 0.000000000000000000, 1.000000000000000000 ) ) ;
#18425=DIRECTION ( 'NONE',  ( 0.000000000000000000, 0.000000000000000000, 1.000000000000000000 ) ) ;
#18436=ORIENTED_EDGE ( 'NONE', *, *, #1768, .T. ) ;
#18437=CYLINDRICAL_SURFACE ( 'NONE', #39318, 1.000000000000000000 ) ;
#18445=CYLINDRICAL_SURFACE ( 'NONE', #32921, 16.99999999999999645 ) ;
#18446=ADVANCED_FACE ( 'NONE', ( #29079 ), #29284, .F. ) ;
#18451=VERTEX_POINT ( 'NONE', #37629 ) ;
#18457=ADVANCED_FACE ( 'NONE', ( #28475 ), #1053, .F. ) ;
#18463=AXIS2_PLACEMENT_3D ( 'NONE', #9335, #6275, #14554 ) ;
#18465=ORIENTED_EDGE ( 'NONE', *, *, #30713, .T. ) ;
#18466=EDGE_CURVE ( 'NONE', #27796, #34177, #4295, .T. ) ;
#18492=CYLINDRICAL_SURFACE ( 'NONE', #2960, 1.000000000000000000 ) ;
#18503=ORIENTED_EDGE ( 'NONE', *, *, #13854, .T. ) ;
#18505=CIRCLE ( 'NONE', #19802, 1.000000000000000000 ) ;
#18510=EDGE_CURVE ( 'NONE', #2072, #8671, #2063, .T. ) ;
#18515=DIRECTION ( 'NONE',  ( 1.000000000000000000, 0.000000000000000000, 0.000000000000000000 ) ) ;
#18520=CARTESIAN_POINT ( 'NONE',  ( 13.39463915635820790, 18.33192650902018883, 12.00000000000000000 ) ) ;
#18537=FACE_BOUND ( 'NONE', #23825, .T. ) ;
#18542=DIRECTION ( 'NONE',  ( 0.000000000000000000, 0.000000000000000000, 1.000000000000000000 ) ) ;
#18543=ORIENTED_EDGE ( 'NONE', *, *, #37588, .F. ) ;
#18545=CARTESIAN_POINT ( 'NONE',  ( -14.26585111513660031, 17.86474508437623143, 13.00000000000000178 ) ) ;
#18562=EDGE_CURVE ( 'NONE', #37305, #35978, #31054, .T. ) ;
#18563=AXIS2_PLACEMENT_3D ( 'NONE', #37756, #986, #34313 ) ;
#18564=DIRECTION ( 'NONE',  ( 0.000000000000000000, 0.000000000000000000, 1.000000000000000000 ) ) ;
#18566=DIRECTION ( 'NONE',  ( 1.000000000000000000, 0.000000000000000000, 0.000000000000000000 ) ) ;
#18569=DIRECTION ( 'NONE',  ( 0.000000000000000000, 0.000000000000000000, 1.000000000000000000 ) ) ;
#18570=LINE ( 'NONE', #13413, #1295 ) ;
#18579=ORIENTED_EDGE ( 'NONE', *, *, #2912, .T. ) ;
#18588=CARTESIAN_POINT ( 'NONE',  ( -1.981967702234832984, 30.37627742347970283, 13.00000000000000178 ) ) ;
#18589=EDGE_CURVE ( 'NONE', #26936, #14625, #40123, .T. ) ;
#18599=CARTESIAN_POINT ( 'NONE',  ( -7.688306800005769048, 28.52217545723006609, 6.000000000000000000 ) ) ;
#18602=ORIENTED_EDGE ( 'NONE', *, *, #26513, .T. ) ;
#18627=ORIENTED_EDGE ( 'NONE', *, *, #28252, .F. ) ;
#18630=DIRECTION ( 'NONE',  ( 0.000000000000000000, 0.000000000000000000, 1.000000000000000000 ) ) ;
#18636=CARTESIAN_POINT ( 'NONE',  ( -9.559512017365660697, 19.71884705062586107, 12.00000000000000000 ) ) ;
#18656=VECTOR ( 'NONE', #27756, 1000.000000000000000 ) ;
#18659=ORIENTED_EDGE ( 'NONE', *, *, #8863, .T. ) ;
#18662=CARTESIAN_POINT ( 'NONE',  ( -16.99999999999999645, 22.50000000000000355, 13.00000000000000178 ) ) ;
#18666=CARTESIAN_POINT ( 'NONE',  ( 7.064564986133971658, 13.54338174056915456, 13.00000000000000178 ) ) ;
#18670=CIRCLE ( 'NONE', #6986, 1.000000000000000000 ) ;
#18673=ORIENTED_EDGE ( 'NONE', *, *, #34472, .F. ) ;
#18681=AXIS2_PLACEMENT_3D ( 'NONE', #20754, #2655, #27433 ) ;
#18689=CARTESIAN_POINT ( 'NONE',  ( 4.835130509701799362, 15.55077355964573904, 12.00000000000000000 ) ) ;
#18690=DIRECTION ( 'NONE',  ( 0.000000000000000000, 0.000000000000000000, 1.000000000000000000 ) ) ;
#18692=ORIENTED_EDGE ( 'NONE', *, *, #30211, .F. ) ;
#18695=DIRECTION ( 'NONE',  ( 1.000000000000000000, 0.000000000000000000, 0.000000000000000000 ) ) ;
#18705=EDGE_LOOP ( 'NONE', ( #8154, #18332, #36197, #4269 ) ) ;
#18708=CARTESIAN_POINT ( 'NONE',  ( 5.688300058587269170, 16.47782454277055564, 6.000000000000000000 ) ) ;
#18709=CARTESIAN_POINT ( 'NONE',  ( 8.559505275947156377, 25.28115294937476065, 6.000000000000000000 ) ) ;
#18712=CARTESIAN_POINT ( 'NONE',  ( -3.370709253380788084E-06, 22.50000000000031264, 13.00000000000000178 ) ) ;
#18714=DIRECTION ( 'NONE',  ( 0.000000000000000000, 0.000000000000000000, 1.000000000000000000 ) ) ;
#18716=EDGE_CURVE ( 'NONE', #10782, #22096, #29101, .T. ) ;
#18717=CARTESIAN_POINT ( 'NONE',  ( -3.370709253380788084E-06, 22.50000000000031264, 12.00000000000000000 ) ) ;
#18727=VECTOR ( 'NONE', #16090, 1000.000000000000000 ) ;
#18731=ORIENTED_EDGE ( 'NONE', *, *, #8423, .F. ) ;
#18733=AXIS2_PLACEMENT_3D ( 'NONE', #8419, #11267, #29945 ) ;
#18737=FACE_BOUND ( 'NONE', #29290, .T. ) ;
#18741=CARTESIAN_POINT ( 'NONE',  ( 4.458865582155095986, 18.48521636184714012, 12.00000000000000000 ) ) ;
#18742=ORIENTED_EDGE ( 'NONE', *, *, #33004, .T. ) ;
#18747=ORIENTED_EDGE ( 'NONE', *, *, #27248, .F. ) ;
#18749=EDGE_LOOP ( 'NONE', ( #15581, #10608 ) ) ;
#18753=ORIENTED_EDGE ( 'NONE', *, *, #35614, .F. ) ;
#18757=CIRCLE ( 'NONE', #31082, 1.000000000000000888 ) ;
#18767=DIRECTION ( 'NONE',  ( 1.000000000000000000, 0.000000000000000000, 0.000000000000000000 ) ) ;
#18774=DIRECTION ( 'NONE',  ( 1.000000000000000000, 0.000000000000000000, 0.000000000000000000 ) ) ;
#18782=EDGE_CURVE ( 'NONE', #20347, #25619, #33015, .T. ) ;
#18783=FACE_OUTER_BOUND ( 'NONE', #37376, .T. ) ;
#18785=VERTEX_POINT ( 'NONE', #4428 ) ;
#18791=EDGE_CURVE ( 'NONE', #12667, #8118, #20078, .T. ) ;
#18806=ORIENTED_EDGE ( 'NONE', *, *, #9911, .F. ) ;
#18809=EDGE_CURVE ( 'NONE', #6441, #38979, #16792, .T. ) ;
#18814=CARTESIAN_POINT ( 'NONE',  ( 2.835130509701798918, 15.55077355964573904, 13.00000000000000178 ) ) ;
#18816=DIRECTION ( 'NONE',  ( 1.000000000000000000, 0.000000000000000000, 0.000000000000000000 ) ) ;
#18819=CARTESIAN_POINT ( 'NONE',  ( -2.211402178667006169, 32.38366924255629442, 12.00000000000000000 ) ) ;
#18820=DIRECTION ( 'NONE',  ( 0.000000000000000000, 0.000000000000000000, 1.000000000000000000 ) ) ;
#18822=DIRECTION ( 'NONE',  ( 0.000000000000000000, 0.000000000000000000, 1.000000000000000000 ) ) ;
#18831=ORIENTED_EDGE ( 'NONE', *, *, #28583, .F. ) ;
#18839=EDGE_CURVE ( 'NONE', #14121, #35424, #16224, .T. ) ;
#18859=CARTESIAN_POINT ( 'NONE',  ( -12.03641663870442713, 15.85735326529964873, 13.00000000000000178 ) ) ;
#18860=ORIENTED_EDGE ( 'NONE', *, *, #39192, .T. ) ;
#18863=DIRECTION ( 'NONE',  ( 1.000000000000000000, 0.000000000000000000, 0.000000000000000000 ) ) ;
#18864=DIRECTION ( 'NONE',  ( 0.000000000000000000, 0.000000000000000000, 1.000000000000000000 ) ) ;
#18866=CARTESIAN_POINT ( 'NONE',  ( 3.476901250629512941, 26.36149378532653031, 13.00000000000000178 ) ) ;
#18871=CARTESIAN_POINT ( 'NONE',  ( 7.935770203493858865, 22.34671014717335780, 13.00000000000000178 ) ) ;
#18873=DIRECTION ( 'NONE',  ( 0.000000000000000000, 0.000000000000000000, 1.000000000000000000 ) ) ;
#18874=CIRCLE ( 'NONE', #1361, 1.000000000000000000 ) ;
#18885=ORIENTED_EDGE ( 'NONE', *, *, #31009, .F. ) ;
#18888=DIRECTION ( 'NONE',  ( 1.000000000000000000, 0.000000000000000000, 0.000000000000000000 ) ) ;
#18890=ORIENTED_EDGE ( 'NONE', *, *, #29947, .T. ) ;
#18896=CARTESIAN_POINT ( 'NONE',  ( -13.26585111513660031, 17.86474508437623143, 12.00000000000000000 ) ) ;
#18899=EDGE_LOOP ( 'NONE', ( #17752, #35389 ) ) ;
#18908=EDGE_CURVE ( 'NONE', #28710, #39968, #18101, .T. ) ;
#18911=EDGE_CURVE ( 'NONE', #36946, #14129, #30427, .T. ) ;
#18916=CIRCLE ( 'NONE', #35129, 2.000000000000001776 ) ;
#18921=EDGE_LOOP ( 'NONE', ( #6294, #31803 ) ) ;
#18931=FACE_BOUND ( 'NONE', #5134, .T. ) ;
#18935=DIRECTION ( 'NONE',  ( 0.000000000000000000, 0.000000000000000000, 1.000000000000000000 ) ) ;
#18936=EDGE_LOOP ( 'NONE', ( #17545, #9952, #17293, #23560 ) ) ;
#18947=ORIENTED_EDGE ( 'NONE', *, *, #34399, .T. ) ;
#18949=DIRECTION ( 'NONE',  ( 1.000000000000000000, 0.000000000000000000, 0.000000000000000000 ) ) ;
#18952=EDGE_CURVE ( 'NONE', #37992, #2950, #5124, .T. ) ;
#18953=AXIS2_PLACEMENT_3D ( 'NONE', #5209, #29992, #17621 ) ;
#18956=CIRCLE ( 'NONE', #34539, 1.000000000000000000 ) ;
#18958=EDGE_CURVE ( 'NONE', #7705, #33301, #20713, .T. ) ;
#18961=DIRECTION ( 'NONE',  ( 0.000000000000000000, 0.000000000000000000, 1.000000000000000000 ) ) ;
#18970=CARTESIAN_POINT ( 'NONE',  ( -7.917741276437941345, 30.52956727630665057, 6.000000000000000000 ) ) ;
#18994=CIRCLE ( 'NONE', #34562, 1.000000000000000888 ) ;
#18996=VERTEX_POINT ( 'NONE', #36119 ) ;
#18998=FACE_OUTER_BOUND ( 'NONE', #17143, .T. ) ;
#18999=ORIENTED_EDGE ( 'NONE', *, *, #13876, .F. ) ;
#19002=AXIS2_PLACEMENT_3D ( 'NONE', #27109, #36058, #8218 ) ;
#19006=DIRECTION ( 'NONE',  ( 1.000000000000000000, 0.000000000000000000, 0.000000000000000000 ) ) ;
#19009=DIRECTION ( 'NONE',  ( 0.000000000000000000, 0.000000000000000000, 1.000000000000000000 ) ) ;
#19012=DIRECTION ( 'NONE',  ( 1.000000000000000000, 0.000000000000000000, 0.000000000000000000 ) ) ;
#19015=ORIENTED_EDGE ( 'NONE', *, *, #7165, .T. ) ;
#19016=CIRCLE ( 'NONE', #17732, 1.000000000000000000 ) ;
#19024=ORIENTED_EDGE ( 'NONE', *, *, #2418, .T. ) ;
#19037=ORIENTED_EDGE ( 'NONE', *, *, #20767, .T. ) ;
#19042=EDGE_LOOP ( 'NONE', ( #23131, #16471, #10033, #16268 ) ) ;
#19051=DIRECTION ( 'NONE',  ( 0.000000000000000000, 0.000000000000000000, 1.000000000000000000 ) ) ;
#19053=EDGE_CURVE ( 'NONE', #24243, #16522, #25244, .T. ) ;
#19054=DIRECTION ( 'NONE',  ( 1.000000000000000000, 0.000000000000000000, 0.000000000000000000 ) ) ;
#19061=DIRECTION ( 'NONE',  ( 0.000000000000000000, 0.000000000000000000, 1.000000000000000000 ) ) ;
#19086=AXIS2_PLACEMENT_3D ( 'NONE', #17330, #1275, #29305 ) ;
#19087=DIRECTION ( 'NONE',  ( 1.000000000000000000, 0.000000000000000000, 0.000000000000000000 ) ) ;
#19095=VERTEX_POINT ( 'NONE', #3376 ) ;
#19104=AXIS2_PLACEMENT_3D ( 'NONE', #17728, #19595, #11421 ) ;
#19107=EDGE_CURVE ( 'NONE', #31085, #34024, #7079, .T. ) ;
#19114=ORIENTED_EDGE ( 'NONE', *, *, #37687, .T. ) ;
#19116=DIRECTION ( 'NONE',  ( 1.000000000000000000, 0.000000000000000000, 0.000000000000000000 ) ) ;
#19124=EDGE_LOOP ( 'NONE', ( #418, #24937, #16675, #2863 ) ) ;
#19129=FACE_BOUND ( 'NONE', #5330, .T. ) ;
#19141=ORIENTED_EDGE ( 'NONE', *, *, #20727, .T. ) ;
#19152=VECTOR ( 'NONE', #7534, 1000.000000000000000 ) ;
#19157=DIRECTION ( 'NONE',  ( 0.000000000000000000, 0.000000000000000000, 1.000000000000000000 ) ) ;
#19164=EDGE_LOOP ( 'NONE', ( #37854, #28284 ) ) ;
#19166=EDGE_LOOP ( 'NONE', ( #7217, #26688, #20701, #776, #38916, #26219, #313 ) ) ;
#19168=DIRECTION ( 'NONE',  ( 1.000000000000000000, 0.000000000000000000, 0.000000000000000000 ) ) ;
#19178=ADVANCED_FACE ( 'NONE', ( #22063 ), #36914, .F. ) ;
#19183=CIRCLE ( 'NONE', #11423, 1.000000000000000000 ) ;
#19187=AXIS2_PLACEMENT_3D ( 'NONE', #23857, #24060, #33424 ) ;
#19192=EDGE_CURVE ( 'NONE', #15391, #16334, #3841, .T. ) ;
#19196=CARTESIAN_POINT ( 'NONE',  ( -6.348113209407908464, 9.835177808069893501, 6.000000000000000000 ) ) ;
#19197=CYLINDRICAL_SURFACE ( 'NONE', #25303, 1.000000000000000888 ) ;
#19202=CARTESIAN_POINT ( 'NONE',  ( 10.41267482483262619, 26.20820393249957192, 13.00000000000000178 ) ) ;
#19206=CARTESIAN_POINT ( 'NONE',  ( -6.312041872459064784, 25.58773265502866678, 6.000000000000000000 ) ) ;
#19207=DIRECTION ( 'NONE',  ( 1.000000000000000000, 0.000000000000000000, 0.000000000000000000 ) ) ;
#19212=AXIS2_PLACEMENT_3D ( 'NONE', #12283, #22020, #6569 ) ;
#19227=ORIENTED_EDGE ( 'NONE', *, *, #3800, .F. ) ;
#19244=FACE_OUTER_BOUND ( 'NONE', #3506, .T. ) ;
#19257=EDGE_LOOP ( 'NONE', ( #28206, #6173, #18122, #39736 ) ) ;
#19262=CARTESIAN_POINT ( 'NONE',  ( -6.706342468480190000, 20.64589803375067945, 13.00000000000000178 ) ) ;
#19266=AXIS2_PLACEMENT_3D ( 'NONE', #10905, #35686, #7841 ) ;
#19278=AXIS2_PLACEMENT_3D ( 'NONE', #327, #31400, #12708 ) ;
#19285=ORIENTED_EDGE ( 'NONE', *, *, #10616, .T. ) ;
#19293=FACE_OUTER_BOUND ( 'NONE', #13486, .T. ) ;
#19296=AXIS2_PLACEMENT_3D ( 'NONE', #5154, #18156, #17560 ) ;
#19300=CARTESIAN_POINT ( 'NONE',  ( 0.9999966292907466192, 22.50000000000031264, 6.000000000000000000 ) ) ;
#19306=EDGE_CURVE ( 'NONE', #7015, #6898, #34331, .T. ) ;
#19314=VERTEX_POINT ( 'NONE', #8675 ) ;
#19319=EDGE_LOOP ( 'NONE', ( #32613, #8823 ) ) ;
#19320=ORIENTED_EDGE ( 'NONE', *, *, #2821, .F. ) ;
#19325=FACE_BOUND ( 'NONE', #23659, .T. ) ;
#19326=CIRCLE ( 'NONE', #38121, 1.000000000000000000 ) ;
#19327=CIRCLE ( 'NONE', #36888, 1.000000000000000888 ) ;
#19332=EDGE_CURVE ( 'NONE', #36663, #20274, #12258, .T. ) ;
#19333=CARTESIAN_POINT ( 'NONE',  ( 13.64210930126480115, 24.20081211342298744, 6.000000000000000000 ) ) ;
#19334=FACE_OUTER_BOUND ( 'NONE', #34022, .T. ) ;
#19335=AXIS2_PLACEMENT_3D ( 'NONE', #23551, #8102, #20513 ) ;
#19349=DIRECTION ( 'NONE',  ( 1.000000000000000000, 0.000000000000000000, 0.000000000000000000 ) ) ;
#19352=FACE_BOUND ( 'NONE', #9663, .T. ) ;
#19369=CARTESIAN_POINT ( 'NONE',  ( -8.294006203984645609, 33.46401007850805343, 12.00000000000000000 ) ) ;
#19382=ORIENTED_EDGE ( 'NONE', *, *, #21885, .T. ) ;
#19392=VERTEX_POINT ( 'NONE', #30009 ) ;
#19393=CARTESIAN_POINT ( 'NONE',  ( 0.7344908159097338629, 8.754836972118123839, 6.000000000000000000 ) ) ;
#19406=DIRECTION ( 'NONE',  ( 0.000000000000000000, 0.000000000000000000, 1.000000000000000000 ) ) ;
#19409=CARTESIAN_POINT ( 'NONE',  ( 10.78893975237932956, 23.27376113029817617, 13.00000000000000178 ) ) ;
#19416=ORIENTED_EDGE ( 'NONE', *, *, #30110, .T. ) ;
#19422=CYLINDRICAL_SURFACE ( 'NONE', #7556, 1.000000000000000000 ) ;
#19436=CARTESIAN_POINT ( 'NONE',  ( -9.294006203984645609, 33.46401007850805343, 13.00000000000000178 ) ) ;
#19444=AXIS2_PLACEMENT_3D ( 'NONE', #5266, #29848, #36351 ) ;
#19445=CYLINDRICAL_SURFACE ( 'NONE', #3474, 1.000000000000000000 ) ;
#19447=DIRECTION ( 'NONE',  ( 1.000000000000000000, 0.000000000000000000, 0.000000000000000000 ) ) ;
#19451=DIRECTION ( 'NONE',  ( 1.000000000000000000, 0.000000000000000000, 0.000000000000000000 ) ) ;
#19457=CARTESIAN_POINT ( 'NONE',  ( 4.476901250629513385, 26.36149378532653031, 12.00000000000000000 ) ) ;
#19458=EDGE_LOOP ( 'NONE', ( #20731, #9657, #22805, #10961 ) ) ;
#19468=DIRECTION ( 'NONE',  ( 1.000000000000000000, 0.000000000000000000, 0.000000000000000000 ) ) ;
#19474=CARTESIAN_POINT ( 'NONE',  ( 7.917734535019441466, 14.47043272369397116, 13.00000000000000178 ) ) ;
#19485=VERTEX_POINT ( 'NONE', #15166 ) ;
#19487=DIRECTION ( 'NONE',  ( 0.000000000000000000, 0.000000000000000000, 1.000000000000000000 ) ) ;
#19490=AXIS2_PLACEMENT_3D ( 'NONE', #6551, #16512, #9416 ) ;
#19492=EDGE_LOOP ( 'NONE', ( #36640, #7088, #27067, #19998 ) ) ;
#19502=DIRECTION ( 'NONE',  ( 0.000000000000000000, 0.000000000000000000, 1.000000000000000000 ) ) ;
#19503=CIRCLE ( 'NONE', #2013, 1.000000000000000000 ) ;
#19509=CARTESIAN_POINT ( 'NONE',  ( 10.14716901145161465, 12.46304090461738667, 12.00000000000000000 ) ) ;
#19512=ADVANCED_FACE ( 'NONE', ( #20677 ), #30212, .F. ) ;
#19528=FACE_OUTER_BOUND ( 'NONE', #10837, .T. ) ;
#19529=EDGE_LOOP ( 'NONE', ( #14763, #28511, #14802, #20994 ) ) ;
#19534=ORIENTED_EDGE ( 'NONE', *, *, #3268, .T. ) ;
#19537=ORIENTED_EDGE ( 'NONE', *, *, #31938, .F. ) ;
#19544=DIRECTION ( 'NONE',  ( 0.000000000000000000, 0.000000000000000000, 1.000000000000000000 ) ) ;
#19546=CIRCLE ( 'NONE', #16980, 1.000000000000000888 ) ;
#19547=FACE_OUTER_BOUND ( 'NONE', #4177, .T. ) ;
#19550=EDGE_CURVE ( 'NONE', #33546, #35323, #601, .T. ) ;
#19551=PLANE ( 'NONE',  #39155 ) ;
#19555=AXIS2_PLACEMENT_3D ( 'NONE', #26427, #32740, #14036 ) ;
#19569=EDGE_LOOP ( 'NONE', ( #25382, #37579 ) ) ;
#19573=CARTESIAN_POINT ( 'NONE',  ( 9.806975420853749625, 31.15003855377755571, 6.000000000000000000 ) ) ;
#19580=EDGE_LOOP ( 'NONE', ( #24377, #539, #10677, #6884 ) ) ;
#19584=EDGE_LOOP ( 'NONE', ( #17871, #16960 ) ) ;
#19591=AXIS2_PLACEMENT_3D ( 'NONE', #8303, #23134, #2016 ) ;
#19595=DIRECTION ( 'NONE',  ( 0.000000000000000000, 0.000000000000000000, 1.000000000000000000 ) ) ;
#19598=DIRECTION ( 'NONE',  ( 0.000000000000000000, 0.000000000000000000, 1.000000000000000000 ) ) ;
#19605=CARTESIAN_POINT ( 'NONE',  ( -3.476907992048017260, 18.63850621467409496, 12.00000000000000000 ) ) ;
#19607=CYLINDRICAL_SURFACE ( 'NONE', #23846, 1.000000000000000000 ) ;
#19611=VERTEX_POINT ( 'NONE', #21852 ) ;
#19619=VERTEX_POINT ( 'NONE', #16162 ) ;
#19633=ORIENTED_EDGE ( 'NONE', *, *, #23709, .F. ) ;
#19642=ORIENTED_EDGE ( 'NONE', *, *, #37398, .T. ) ;
#19643=VECTOR ( 'NONE', #18714, 1000.000000000000000 ) ;
#19644=ORIENTED_EDGE ( 'NONE', *, *, #867, .T. ) ;
#19645=FACE_OUTER_BOUND ( 'NONE', #30125, .T. ) ;
#19648=CARTESIAN_POINT ( 'NONE',  ( -7.577547685840081648, 11.84256962714647798, 6.000000000000000000 ) ) ;
#19649=ORIENTED_EDGE ( 'NONE', *, *, #38567, .T. ) ;
#19659=ORIENTED_EDGE ( 'NONE', *, *, #5773, .F. ) ;
#19676=CARTESIAN_POINT ( 'NONE',  ( 4.458865582155095986, 18.48521636184714012, 6.000000000000000000 ) ) ;
#19679=EDGE_LOOP ( 'NONE', ( #14984, #8244 ) ) ;
#19685=ADVANCED_FACE ( 'NONE', ( #16362 ), #9472, .F. ) ;
#19686=DIRECTION ( 'NONE',  ( 1.000000000000000000, 0.000000000000000000, 0.000000000000000000 ) ) ;
#19690=CARTESIAN_POINT ( 'NONE',  ( -10.78894649379783388, 21.72623886970244911, 6.000000000000000000 ) ) ;
#19699=EDGE_CURVE ( 'NONE', #33109, #1261, #15760, .T. ) ;
#19709=DIRECTION ( 'NONE',  ( 0.000000000000000000, 0.000000000000000000, 1.000000000000000000 ) ) ;
#19715=EDGE_CURVE ( 'NONE', #7574, #36335, #14907, .T. ) ;
#19724=CIRCLE ( 'NONE', #35973, 1.000000000000000000 ) ;
#19731=CARTESIAN_POINT ( 'NONE',  ( -8.935776944912362296, 22.65328985282726393, 6.000000000000000000 ) ) ;
#19732=CARTESIAN_POINT ( 'NONE',  ( 0.000000000000000000, 22.50000000000000355, 13.00000000000000178 ) ) ;
#19744=VERTEX_POINT ( 'NONE', #22052 ) ;
#19749=EDGE_LOOP ( 'NONE', ( #7182, #13144 ) ) ;
#19753=CYLINDRICAL_SURFACE ( 'NONE', #5129, 1.000000000000000000 ) ;
#19757=FACE_BOUND ( 'NONE', #23368, .T. ) ;
#19760=ADVANCED_FACE ( 'NONE', ( #25302 ), #6600, .F. ) ;
#19762=VECTOR ( 'NONE', #21858, 1000.000000000000000 ) ;
#19765=VERTEX_POINT ( 'NONE', #34648 ) ;
#19767=VERTEX_POINT ( 'NONE', #31592 ) ;
#19771=LINE ( 'NONE', #18970, #32185 ) ;
#19775=FACE_OUTER_BOUND ( 'NONE', #26825, .T. ) ;
#19780=CARTESIAN_POINT ( 'NONE',  ( 14.26584437371809777, 27.13525491562438319, 13.00000000000000178 ) ) ;
#19784=DIRECTION ( 'NONE',  ( 1.000000000000000000, 0.000000000000000000, 0.000000000000000000 ) ) ;
#19786=ORIENTED_EDGE ( 'NONE', *, *, #36332, .T. ) ;
#19789=DIRECTION ( 'NONE',  ( 0.000000000000000000, 0.000000000000000000, 1.000000000000000000 ) ) ;
#19790=VERTEX_POINT ( 'NONE', #3761 ) ;
#19793=AXIS2_PLACEMENT_3D ( 'NONE', #20690, #23523, #35312 ) ;
#19795=EDGE_CURVE ( 'NONE', #29833, #29063, #2577, .T. ) ;
#19797=ORIENTED_EDGE ( 'NONE', *, *, #25637, .T. ) ;
#19798=EDGE_CURVE ( 'NONE', #3673, #21859, #16566, .T. ) ;
#19799=CIRCLE ( 'NONE', #14639, 1.000000000000000000 ) ;
#19802=AXIS2_PLACEMENT_3D ( 'NONE', #31450, #13354, #18863 ) ;
#19805=DIRECTION ( 'NONE',  ( 1.000000000000000000, 0.000000000000000000, 0.000000000000000000 ) ) ;
#19806=CARTESIAN_POINT ( 'NONE',  ( -5.348113209407908464, 9.835177808069893501, 12.00000000000000000 ) ) ;
#19809=FACE_OUTER_BOUND ( 'NONE', #35638, .T. ) ;
#19810=VERTEX_POINT ( 'NONE', #14113 ) ;
#19811=FACE_OUTER_BOUND ( 'NONE', #14523, .T. ) ;
#19812=CYLINDRICAL_SURFACE ( 'NONE', #27222, 1.000000000000000000 ) ;
#19816=DIRECTION ( 'NONE',  ( 1.000000000000000000, 0.000000000000000000, 0.000000000000000000 ) ) ;
#19821=( NAMED_UNIT ( * ) PLANE_ANGLE_UNIT ( ) SI_UNIT ( $, .RADIAN. ) );
#19828=ORIENTED_EDGE ( 'NONE', *, *, #34478, .T. ) ;
#19830=EDGE_LOOP ( 'NONE', ( #4708, #1758, #20912, #33149 ) ) ;
#19836=CIRCLE ( 'NONE', #23077, 1.000000000000000888 ) ;
#19843=DIRECTION ( 'NONE',  ( 1.000000000000000000, 0.000000000000000000, 0.000000000000000000 ) ) ;
#19845=EDGE_LOOP ( 'NONE', ( #36463, #26485 ) ) ;
#19847=ADVANCED_FACE ( 'NONE', ( #38902 ), #11078, .F. ) ;
#19850=EDGE_CURVE ( 'NONE', #7138, #7015, #35854, .T. ) ;
#19858=VECTOR ( 'NONE', #32780, 1000.000000000000000 ) ;
#19860=AXIS2_PLACEMENT_3D ( 'NONE', #22701, #775, #24408 ) ;
#19863=VERTEX_POINT ( 'NONE', #23462 ) ;
#19866=VECTOR ( 'NONE', #14978, 1000.000000000000000 ) ;
#19867=CARTESIAN_POINT ( 'NONE',  ( -10.41268156625113228, 18.79179606750104981, 6.000000000000000000 ) ) ;
#19881=DIRECTION ( 'NONE',  ( 0.000000000000000000, 0.000000000000000000, 1.000000000000000000 ) ) ;
#19888=ORIENTED_EDGE ( 'NONE', *, *, #23709, .T. ) ;
#19893=DIRECTION ( 'NONE',  ( 1.000000000000000000, 0.000000000000000000, 0.000000000000000000 ) ) ;
#19898=ORIENTED_EDGE ( 'NONE', *, *, #12103, .F. ) ;
#19913=DIRECTION ( 'NONE',  ( 0.000000000000000000, 0.000000000000000000, 1.000000000000000000 ) ) ;
#19915=AXIS2_PLACEMENT_3D ( 'NONE', #29788, #39526, #2753 ) ;
#19918=ORIENTED_EDGE ( 'NONE', *, *, #15922, .F. ) ;
#19919=FACE_OUTER_BOUND ( 'NONE', #9556, .T. ) ;
#19924=DIRECTION ( 'NONE',  ( 0.000000000000000000, 0.000000000000000000, 1.000000000000000000 ) ) ;
#19933=ORIENTED_EDGE ( 'NONE', *, *, #12220, .F. ) ;
#19934=VERTEX_POINT ( 'NONE', #38495 ) ;
#19943=CARTESIAN_POINT ( 'NONE',  ( -7.294006203984644721, 33.46401007850805343, 13.00000000000000178 ) ) ;
#19944=ORIENTED_EDGE ( 'NONE', *, *, #23794, .F. ) ;
#19953=EDGE_CURVE ( 'NONE', #12151, #7227, #39540, .T. ) ;
#19956=ADVANCED_FACE ( 'NONE', ( #38293 ), #19812, .F. ) ;
#19958=DIRECTION ( 'NONE',  ( 0.000000000000000000, 0.000000000000000000, 1.000000000000000000 ) ) ;
#19960=AXIS2_PLACEMENT_3D ( 'NONE', #3740, #28129, #7939 ) ;
#19963=DIRECTION ( 'NONE',  ( 1.000000000000000000, 0.000000000000000000, 0.000000000000000000 ) ) ;
#19967=CIRCLE ( 'NONE', #30359, 1.000000000000000000 ) ;
#19972=AXIS2_PLACEMENT_3D ( 'NONE', #34731, #22934, #19686 ) ;
#19988=CIRCLE ( 'NONE', #19960, 1.000000000000000888 ) ;
#19994=ORIENTED_EDGE ( 'NONE', *, *, #36102, .T. ) ;
#19996=CARTESIAN_POINT ( 'NONE',  ( 9.788939752379329562, 23.27376113029817617, 13.00000000000000178 ) ) ;
#19998=ORIENTED_EDGE ( 'NONE', *, *, #12462, .F. ) ;
#20008=AXIS2_PLACEMENT_3D ( 'NONE', #15144, #39916, #12096 ) ;
#20009=CARTESIAN_POINT ( 'NONE',  ( -1.981967702234832984, 30.37627742347970283, 12.00000000000000000 ) ) ;
#20013=CARTESIAN_POINT ( 'NONE',  ( -1.605702774688126722, 27.44183462127829642, 13.00000000000000178 ) ) ;
#20014=CYLINDRICAL_SURFACE ( 'NONE', #2959, 1.000000000000000000 ) ;
#20046=FACE_OUTER_BOUND ( 'NONE', #18041, .T. ) ;
#20049=ORIENTED_EDGE ( 'NONE', *, *, #2821, .T. ) ;
#20058=EDGE_CURVE ( 'NONE', #20274, #36663, #29831, .T. ) ;
#20065=CARTESIAN_POINT ( 'NONE',  ( -11.14717575287011542, 32.53695909538323860, 12.00000000000000000 ) ) ;
#20078=LINE ( 'NONE', #25755, #8348 ) ;
#20080=EDGE_CURVE ( 'NONE', #34024, #13841, #24456, .T. ) ;
#20094=ORIENTED_EDGE ( 'NONE', *, *, #37842, .F. ) ;
#20095=AXIS2_PLACEMENT_3D ( 'NONE', #19605, #1735, #38701 ) ;
#20096=CARTESIAN_POINT ( 'NONE',  ( -2.476907992048017260, 18.63850621467409496, 13.00000000000000178 ) ) ;
#20101=ORIENTED_EDGE ( 'NONE', *, *, #32069, .F. ) ;
#20107=ORIENTED_EDGE ( 'NONE', *, *, #32878, .T. ) ;
#20111=DIRECTION ( 'NONE',  ( 1.000000000000000000, 0.000000000000000000, 0.000000000000000000 ) ) ;
#20118=CARTESIAN_POINT ( 'NONE',  ( -6.064571727552472424, 31.45661825943146894, 13.00000000000000178 ) ) ;
#20122=AXIS2_PLACEMENT_3D ( 'NONE', #27507, #39096, #33623 ) ;
#20126=EDGE_CURVE ( 'NONE', #30574, #23393, #10341, .T. ) ;
#20140=FACE_BOUND ( 'NONE', #21788, .T. ) ;
#20141=VECTOR ( 'NONE', #11567, 1000.000000000000000 ) ;
#20157=ADVANCED_FACE ( 'NONE', ( #18370, #26708 ), #5372, .F. ) ;
#20163=ORIENTED_EDGE ( 'NONE', *, *, #18809, .F. ) ;
#20165=ADVANCED_FACE ( 'NONE', ( #8827 ), #21213, .F. ) ;
#20173=DIRECTION ( 'NONE',  ( 1.000000000000000000, 0.000000000000000000, 0.000000000000000000 ) ) ;
#20174=ORIENTED_EDGE ( 'NONE', *, *, #28630, .T. ) ;
#20180=DIRECTION ( 'NONE',  ( 1.000000000000000000, 0.000000000000000000, 0.000000000000000000 ) ) ;
#20184=VECTOR ( 'NONE', #37553, 1000.000000000000000 ) ;
#20185=ORIENTED_EDGE ( 'NONE', *, *, #29148, .T. ) ;
#20189=FACE_OUTER_BOUND ( 'NONE', #15450, .T. ) ;
#20197=CARTESIAN_POINT ( 'NONE',  ( 1.605696033269625955, 17.55816537872232530, 6.000000000000000000 ) ) ;
#20199=EDGE_LOOP ( 'NONE', ( #28445, #27518, #4497, #18692 ) ) ;
#20206=ORIENTED_EDGE ( 'NONE', *, *, #1223, .F. ) ;
#20211=ADVANCED_FACE ( 'NONE', ( #15314 ), #37251, .F. ) ;
#20213=CARTESIAN_POINT ( 'NONE',  ( 0.6237317017440463518, 25.43444280220171194, 6.000000000000000000 ) ) ;
#20216=ORIENTED_EDGE ( 'NONE', *, *, #39284, .T. ) ;
#20224=( NAMED_UNIT ( * ) SI_UNIT ( $, .STERADIAN. ) SOLID_ANGLE_UNIT ( ) );
#20230=EDGE_CURVE ( 'NONE', #16334, #33648, #13615, .T. ) ;
#20233=LINE ( 'NONE', #7825, #12658 ) ;
#20245=ORIENTED_EDGE ( 'NONE', *, *, #22187, .T. ) ;
#20256=EDGE_CURVE ( 'NONE', #6396, #33348, #28855, .T. ) ;
#20264=EDGE_LOOP ( 'NONE', ( #25128, #37146, #27440, #4046 ) ) ;
#20269=CARTESIAN_POINT ( 'NONE',  ( 13.64210930126480115, 24.20081211342298744, 13.00000000000000178 ) ) ;
#20270=CARTESIAN_POINT ( 'NONE',  ( -9.917741276437942233, 30.52956727630665057, 6.000000000000000000 ) ) ;
#20271=CARTESIAN_POINT ( 'NONE',  ( -3.587667106213709101, 35.31811204475769728, 13.00000000000000178 ) ) ;
#20274=VERTEX_POINT ( 'NONE', #4271 ) ;
#20277=CARTESIAN_POINT ( 'NONE',  ( -10.78894649379783388, 21.72623886970244911, 12.00000000000000000 ) ) ;
#20284=EDGE_CURVE ( 'NONE', #20274, #1646, #18570, .T. ) ;
#20286=CIRCLE ( 'NONE', #17690, 1.000000000000000888 ) ;
#20291=ORIENTED_EDGE ( 'NONE', *, *, #31121, .F. ) ;
#20294=CIRCLE ( 'NONE', #12506, 1.000000000000000888 ) ;
#20295=CARTESIAN_POINT ( 'NONE',  ( -11.77091082532341204, 29.60251629318183575, 13.00000000000000178 ) ) ;
#20296=ORIENTED_EDGE ( 'NONE', *, *, #33374, .F. ) ;
#20298=CIRCLE ( 'NONE', #33274, 1.000000000000000000 ) ;
#20302=EDGE_CURVE ( 'NONE', #19765, #32281, #31156, .T. ) ;
#20305=AXIS2_PLACEMENT_3D ( 'NONE', #8140, #14435, #29280 ) ;
#20310=DIRECTION ( 'NONE',  ( 0.000000000000000000, 0.000000000000000000, 1.000000000000000000 ) ) ;
#20312=AXIS2_PLACEMENT_3D ( 'NONE', #30422, #35711, #7865 ) ;
#20317=CARTESIAN_POINT ( 'NONE',  ( 6.064564986133971658, 13.54338174056915456, 12.00000000000000000 ) ) ;
#20319=DIRECTION ( 'NONE',  ( 0.000000000000000000, 0.000000000000000000, 1.000000000000000000 ) ) ;
#20330=EDGE_CURVE ( 'NONE', #35813, #32704, #18180, .T. ) ;
#20339=VERTEX_POINT ( 'NONE', #19509 ) ;
#20340=EDGE_LOOP ( 'NONE', ( #20296, #13482, #16617, #3703 ) ) ;
#20344=FACE_BOUND ( 'NONE', #6912, .T. ) ;
#20347=VERTEX_POINT ( 'NONE', #37450 ) ;
#20350=DIRECTION ( 'NONE',  ( 0.000000000000000000, 0.000000000000000000, 1.000000000000000000 ) ) ;
#20356=ORIENTED_EDGE ( 'NONE', *, *, #38437, .T. ) ;
#20361=VERTEX_POINT ( 'NONE', #31902 ) ;
#20366=DIRECTION ( 'NONE',  ( 0.000000000000000000, 0.000000000000000000, 1.000000000000000000 ) ) ;
#20369=DIRECTION ( 'NONE',  ( 0.000000000000000000, 0.000000000000000000, 1.000000000000000000 ) ) ;
#20377=DIRECTION ( 'NONE',  ( 0.000000000000000000, 0.000000000000000000, 1.000000000000000000 ) ) ;
#20379=CARTESIAN_POINT ( 'NONE',  ( -11.78894649379783388, 21.72623886970244911, 12.00000000000000000 ) ) ;
#20387=EDGE_LOOP ( 'NONE', ( #12163, #13444, #30645, #15252, #29730, #13794, #20946, #23581 ) ) ;
#20390=ORIENTED_EDGE ( 'NONE', *, *, #23510, .F. ) ;
#20392=CARTESIAN_POINT ( 'NONE',  ( -2.853172919594720192, 21.57294901687549427, 6.000000000000000000 ) ) ;
#20394=CARTESIAN_POINT ( 'NONE',  ( -5.706342468480190000, 20.64589803375067945, 13.00000000000000178 ) ) ;
#20396=ORIENTED_EDGE ( 'NONE', *, *, #10139, .F. ) ;
#20399=DIRECTION ( 'NONE',  ( 0.000000000000000000, 0.000000000000000000, 1.000000000000000000 ) ) ;
#20415=DIRECTION ( 'NONE',  ( 1.000000000000000000, 0.000000000000000000, 0.000000000000000000 ) ) ;
#20419=CYLINDRICAL_SURFACE ( 'NONE', #39288, 1.000000000000000888 ) ;
#20425=DIRECTION ( 'NONE',  ( 1.000000000000000000, 0.000000000000000000, 0.000000000000000000 ) ) ;
#20464=EDGE_CURVE ( 'NONE', #20641, #15085, #11681, .T. ) ;
#20467=DIRECTION ( 'NONE',  ( 1.000000000000000000, 0.000000000000000000, 0.000000000000000000 ) ) ;
#20470=DIRECTION ( 'NONE',  ( 1.000000000000000000, 0.000000000000000000, 0.000000000000000000 ) ) ;
#20474=AXIS2_PLACEMENT_3D ( 'NONE', #9230, #2933, #15721 ) ;
#20483=AXIS2_PLACEMENT_3D ( 'NONE', #404, #18690, #18888 ) ;
#20496=DIRECTION ( 'NONE',  ( 0.000000000000000000, 0.000000000000000000, 1.000000000000000000 ) ) ;
#20502=LINE ( 'NONE', #17461, #25200 ) ;
#20503=CARTESIAN_POINT ( 'NONE',  ( 5.330070799514983193, 27.28854476845134513, 6.000000000000000000 ) ) ;
#20510=AXIS2_PLACEMENT_3D ( 'NONE', #31418, #2791, #34470 ) ;
#20511=AXIS2_PLACEMENT_3D ( 'NONE', #11581, #32317, #39604 ) ;
#20513=DIRECTION ( 'NONE',  ( 1.000000000000000000, 0.000000000000000000, 0.000000000000000000 ) ) ;
#20514=VERTEX_POINT ( 'NONE', #29261 ) ;
#20517=DIRECTION ( 'NONE',  ( 1.224646799147353207E-16, 1.000000000000000000, -0.000000000000000000 ) ) ;
#20520=DIRECTION ( 'NONE',  ( 1.000000000000000000, 0.000000000000000000, 0.000000000000000000 ) ) ;
#20521=CARTESIAN_POINT ( 'NONE',  ( -3.370709253380788084E-06, 22.50000000000031264, 13.00000000000000178 ) ) ;
#20525=ORIENTED_EDGE ( 'NONE', *, *, #12742, .F. ) ;
#20526=DIRECTION ( 'NONE',  ( 0.000000000000000000, 0.000000000000000000, 1.000000000000000000 ) ) ;
#20529=DIRECTION ( 'NONE',  ( 0.000000000000000000, 0.000000000000000000, 1.000000000000000000 ) ) ;
#20534=AXIS2_PLACEMENT_3D ( 'NONE', #39514, #14534, #21034 ) ;
#20551=DIRECTION ( 'NONE',  ( 0.000000000000000000, 0.000000000000000000, 1.000000000000000000 ) ) ;
#20561=ADVANCED_FACE ( 'NONE', ( #17288 ), #29661, .F. ) ;
#20567=AXIS2_PLACEMENT_3D ( 'NONE', #9053, #23888, #11900 ) ;
#20568=AXIS2_PLACEMENT_3D ( 'NONE', #4741, #14076, #35823 ) ;
#20571=CARTESIAN_POINT ( 'NONE',  ( -9.806982162272253944, 13.84996144622306247, 6.000000000000000000 ) ) ;
#20579=DIRECTION ( 'NONE',  ( 0.000000000000000000, 0.000000000000000000, 1.000000000000000000 ) ) ;
#20584=VERTEX_POINT ( 'NONE', #10775 ) ;
#20587=ADVANCED_FACE ( 'NONE', ( #11382 ), #27017, .F. ) ;
#20588=CARTESIAN_POINT ( 'NONE',  ( 12.03640989728592459, 29.14264673470096767, 6.000000000000000000 ) ) ;
#20594=LINE ( 'NONE', #5143, #37433 ) ;
#20596=DIRECTION ( 'NONE',  ( 1.000000000000000000, 0.000000000000000000, 0.000000000000000000 ) ) ;
#20598=ORIENTED_EDGE ( 'NONE', *, *, #29827, .F. ) ;
#20628=DIRECTION ( 'NONE',  ( 1.000000000000000000, 0.000000000000000000, 0.000000000000000000 ) ) ;
#20633=ORIENTED_EDGE ( 'NONE', *, *, #17533, .F. ) ;
#20636=EDGE_CURVE ( 'NONE', #29833, #10872, #15022, .T. ) ;
#20641=VERTEX_POINT ( 'NONE', #33328 ) ;
#20653=LINE ( 'NONE', #14346, #38740 ) ;
#20667=VECTOR ( 'NONE', #14648, 1000.000000000000000 ) ;
#20670=DIRECTION ( 'NONE',  ( 1.000000000000000000, 0.000000000000000000, 0.000000000000000000 ) ) ;
#20672=EDGE_LOOP ( 'NONE', ( #1821, #20291, #33197, #20781 ) ) ;
#20676=EDGE_CURVE ( 'NONE', #39686, #37976, #27000, .T. ) ;
#20677=FACE_OUTER_BOUND ( 'NONE', #14657, .T. ) ;
#20680=CARTESIAN_POINT ( 'NONE',  ( 8.917734535019441466, 14.47043272369397116, 12.00000000000000000 ) ) ;
#20690=CARTESIAN_POINT ( 'NONE',  ( 1.871201846650637046, 31.30332840660451765, 12.00000000000000000 ) ) ;
#20699=DIRECTION ( 'NONE',  ( 1.000000000000000000, 0.000000000000000000, 0.000000000000000000 ) ) ;
#20701=ORIENTED_EDGE ( 'NONE', *, *, #35230, .T. ) ;
#20703=ORIENTED_EDGE ( 'NONE', *, *, #8610, .T. ) ;
#20706=DIRECTION ( 'NONE',  ( 1.000000000000000000, 0.000000000000000000, 0.000000000000000000 ) ) ;
#20713=CIRCLE ( 'NONE', #16170, 1.000000000000000888 ) ;
#20714=ORIENTED_EDGE ( 'NONE', *, *, #22401, .T. ) ;
#20723=VERTEX_POINT ( 'NONE', #39996 ) ;
#20724=SURFACE_SIDE_STYLE ('',( #11374 ) ) ;
#20727=EDGE_CURVE ( 'NONE', #6144, #18451, #6272, .T. ) ;
#20731=ORIENTED_EDGE ( 'NONE', *, *, #35845, .F. ) ;
#20739=AXIS2_PLACEMENT_3D ( 'NONE', #15564, #25102, #525 ) ;
#20746=VERTEX_POINT ( 'NONE', #25354 ) ;
#20747=CIRCLE ( 'NONE', #33714, 1.000000000000000888 ) ;
#20751=CARTESIAN_POINT ( 'NONE',  ( -3.211402178667006169, 32.38366924255629442, 12.00000000000000000 ) ) ;
#20754=CARTESIAN_POINT ( 'NONE',  ( 6.064564986133971658, 13.54338174056915456, 13.00000000000000178 ) ) ;
#20756=CARTESIAN_POINT ( 'NONE',  ( 10.16520467992603294, 20.33931832809677331, 13.00000000000000178 ) ) ;
#20760=ORIENTED_EDGE ( 'NONE', *, *, #37842, .T. ) ;
#20767=EDGE_CURVE ( 'NONE', #839, #36138, #36087, .T. ) ;
#20770=DIRECTION ( 'NONE',  ( 0.000000000000000000, 0.000000000000000000, 1.000000000000000000 ) ) ;
#20781=ORIENTED_EDGE ( 'NONE', *, *, #29494, .T. ) ;
#20794=LINE ( 'NONE', #11840, #37345 ) ;
#20795=EDGE_CURVE ( 'NONE', #26036, #22756, #23105, .T. ) ;
#20803=DIRECTION ( 'NONE',  ( 0.000000000000000000, 0.000000000000000000, 1.000000000000000000 ) ) ;
#20811=CARTESIAN_POINT ( 'NONE',  ( 1.247466774197339978, 28.36888560440311480, 13.00000000000000178 ) ) ;
#20818=DIRECTION ( 'NONE',  ( 1.000000000000000000, 0.000000000000000000, 0.000000000000000000 ) ) ;
#20823=DIRECTION ( 'NONE',  ( 1.000000000000000000, 0.000000000000000000, 0.000000000000000000 ) ) ;
#20827=DIRECTION ( 'NONE',  ( 0.000000000000000000, 0.000000000000000000, 1.000000000000000000 ) ) ;
#20840=CARTESIAN_POINT ( 'NONE',  ( -4.440836655099179353, 34.39106106163288246, 13.00000000000000178 ) ) ;
#20843=DIRECTION ( 'NONE',  ( 1.000000000000000000, 0.000000000000000000, 0.000000000000000000 ) ) ;
#20854=FACE_OUTER_BOUND ( 'NONE', #4690, .T. ) ;
#20855=CARTESIAN_POINT ( 'NONE',  ( -7.312041872459064784, 25.58773265502866678, 13.00000000000000178 ) ) ;
#20861=AXIS2_PLACEMENT_3D ( 'NONE', #29404, #10720, #13965 ) ;
#20866=ORIENTED_EDGE ( 'NONE', *, *, #10413, .T. ) ;
#20868=CIRCLE ( 'NONE', #2048, 1.000000000000000000 ) ;
#20869=DIRECTION ( 'NONE',  ( 0.000000000000000000, 0.000000000000000000, 1.000000000000000000 ) ) ;
#20870=ORIENTED_EDGE ( 'NONE', *, *, #15975, .F. ) ;
#20880=ORIENTED_EDGE ( 'NONE', *, *, #9132, .F. ) ;
#20889=LINE ( 'NONE', #2792, #600 ) ;
#20895=EDGE_CURVE ( 'NONE', #23748, #33425, #15974, .T. ) ;
#20898=CARTESIAN_POINT ( 'NONE',  ( -5.953812613386785912, 14.77701242934787906, 12.00000000000000000 ) ) ;
#20907=EDGE_LOOP ( 'NONE', ( #15207, #10175 ) ) ;
#20910=AXIS2_PLACEMENT_3D ( 'NONE', #3734, #38471, #28719 ) ;
#20912=ORIENTED_EDGE ( 'NONE', *, *, #12408, .T. ) ;
#20915=EDGE_CURVE ( 'NONE', #7288, #32493, #4927, .T. ) ;
#20919=VERTEX_POINT ( 'NONE', #13768 ) ;
#20930=EDGE_CURVE ( 'NONE', #1258, #29599, #38961, .T. ) ;
#20945=EDGE_CURVE ( 'NONE', #40046, #7967, #37379, .T. ) ;
#20946=ORIENTED_EDGE ( 'NONE', *, *, #24265, .F. ) ;
#20948=DIRECTION ( 'NONE',  ( 1.000000000000000000, 0.000000000000000000, 0.000000000000000000 ) ) ;
#20954=DIRECTION ( 'NONE',  ( -1.000000000000000000, 0.000000000000000000, 0.000000000000000000 ) ) ;
#20958=CARTESIAN_POINT ( 'NONE',  ( -12.39464589777671044, 26.66807349098043289, 13.00000000000000178 ) ) ;
#20960=DIRECTION ( 'NONE',  ( 0.000000000000000000, 0.000000000000000000, 1.000000000000000000 ) ) ;
#20961=EDGE_CURVE ( 'NONE', #17675, #36412, #13974, .T. ) ;
#20962=VECTOR ( 'NONE', #28048, 1000.000000000000000 ) ;
#20964=EDGE_CURVE ( 'NONE', #12988, #22962, #23747, .T. ) ;
#20967=DIRECTION ( 'NONE',  ( 1.000000000000000000, 0.000000000000000000, 0.000000000000000000 ) ) ;
#20971=LINE ( 'NONE', #15069, #6632 ) ;
#20972=CARTESIAN_POINT ( 'NONE',  ( -5.706342468480190000, 20.64589803375067945, 13.00000000000000178 ) ) ;
#20976=ORIENTED_EDGE ( 'NONE', *, *, #18839, .T. ) ;
#20983=EDGE_LOOP ( 'NONE', ( #25133, #36689 ) ) ;
#20985=CARTESIAN_POINT ( 'NONE',  ( 7.293999462566144842, 11.53598992149257008, 13.00000000000000178 ) ) ;
#20994=ORIENTED_EDGE ( 'NONE', *, *, #35569, .F. ) ;
#20999=EDGE_LOOP ( 'NONE', ( #27074, #12032 ) ) ;
#21005=EDGE_LOOP ( 'NONE', ( #30803, #18885 ) ) ;
#21008=CARTESIAN_POINT ( 'NONE',  ( -9.806982162272253944, 13.84996144622306247, 6.000000000000000000 ) ) ;
#21011=CARTESIAN_POINT ( 'NONE',  ( 8.293999462566144842, 11.53598992149257008, 12.00000000000000000 ) ) ;
#21013=AXIS2_PLACEMENT_3D ( 'NONE', #8274, #8069, #7669 ) ;
#21014=FACE_BOUND ( 'NONE', #8743, .T. ) ;
#21019=CARTESIAN_POINT ( 'NONE',  ( -0.2655091840902661926, 8.754836972118123839, 13.00000000000000178 ) ) ;
#21030=ORIENTED_EDGE ( 'NONE', *, *, #35387, .T. ) ;
#21034=DIRECTION ( 'NONE',  ( 1.000000000000000000, 0.000000000000000000, 0.000000000000000000 ) ) ;
#21042=VERTEX_POINT ( 'NONE', #24322 ) ;
#21043=EDGE_CURVE ( 'NONE', #24994, #14246, #2987, .T. ) ;
#21048=ORIENTED_EDGE ( 'NONE', *, *, #2137, .T. ) ;
#21050=CIRCLE ( 'NONE', #24294, 1.000000000000000888 ) ;
#21062=EDGE_CURVE ( 'NONE', #8150, #15766, #9083, .T. ) ;
#21066=CARTESIAN_POINT ( 'NONE',  ( -4.724378136954611840, 12.76962061027129458, 12.00000000000000000 ) ) ;
#21068=DIRECTION ( 'NONE',  ( 0.000000000000000000, 0.000000000000000000, 1.000000000000000000 ) ) ;
#21070=DIRECTION ( 'NONE',  ( 0.000000000000000000, 0.000000000000000000, 1.000000000000000000 ) ) ;
#21072=AXIS2_PLACEMENT_3D ( 'NONE', #33920, #36765, #24168 ) ;
#21074=CARTESIAN_POINT ( 'NONE',  ( 2.494936919103933448, 34.23777120880591696, 12.00000000000000000 ) ) ;
#21075=VERTEX_POINT ( 'NONE', #5627 ) ;
#21082=ORIENTED_EDGE ( 'NONE', *, *, #10390, .T. ) ;
#21084=DIRECTION ( 'NONE',  ( 0.000000000000000000, 0.000000000000000000, 1.000000000000000000 ) ) ;
#21085=EDGE_CURVE ( 'NONE', #6918, #36141, #15374, .T. ) ;
#21094=VERTEX_POINT ( 'NONE', #5833 ) ;
#21096=ORIENTED_EDGE ( 'NONE', *, *, #4707, .T. ) ;
#21098=CARTESIAN_POINT ( 'NONE',  ( -9.788946493797832105, 21.72623886970244911, 13.00000000000000178 ) ) ;
#21101=CIRCLE ( 'NONE', #39909, 1.000000000000000888 ) ;
#21105=ORIENTED_EDGE ( 'NONE', *, *, #29866, .F. ) ;
#21108=DIRECTION ( 'NONE',  ( 1.000000000000000000, 0.000000000000000000, 0.000000000000000000 ) ) ;
#21112=ORIENTED_EDGE ( 'NONE', *, *, #9858, .T. ) ;
#21113=CYLINDRICAL_SURFACE ( 'NONE', #15886, 1.000000000000000888 ) ;
#21121=CARTESIAN_POINT ( 'NONE',  ( -8.577547685840080760, 11.84256962714647798, 12.00000000000000000 ) ) ;
#21129=CARTESIAN_POINT ( 'NONE',  ( 4.082600654608392610, 21.41965916404854298, 12.00000000000000000 ) ) ;
#21133=CIRCLE ( 'NONE', #34130, 1.000000000000000000 ) ;
#21134=DIRECTION ( 'NONE',  ( 1.000000000000000000, 0.000000000000000000, 0.000000000000000000 ) ) ;
#21139=ORIENTED_EDGE ( 'NONE', *, *, #2616, .F. ) ;
#21152=CYLINDRICAL_SURFACE ( 'NONE', #28628, 1.000000000000000000 ) ;
#21154=CARTESIAN_POINT ( 'NONE',  ( 5.082600654608392610, 21.41965916404854298, 13.00000000000000178 ) ) ;
#21161=CIRCLE ( 'NONE', #20534, 1.000000000000000888 ) ;
#21162=FACE_OUTER_BOUND ( 'NONE', #37093, .T. ) ;
#21163=EDGE_CURVE ( 'NONE', #21833, #12134, #40152, .T. ) ;
#21166=EDGE_CURVE ( 'NONE', #15751, #33185, #30250, .T. ) ;
#21171=ORIENTED_EDGE ( 'NONE', *, *, #14892, .F. ) ;
#21186=VERTEX_POINT ( 'NONE', #26972 ) ;
#21208=FACE_BOUND ( 'NONE', #26422, .T. ) ;
#21213=CYLINDRICAL_SURFACE ( 'NONE', #20122, 1.000000000000000888 ) ;
#21225=EDGE_LOOP ( 'NONE', ( #37347, #32747 ) ) ;
#21231=CARTESIAN_POINT ( 'NONE',  ( -3.118678732975735279, 7.827785988993307242, 6.000000000000000000 ) ) ;
#21232=AXIS2_PLACEMENT_3D ( 'NONE', #5428, #8271, #17433 ) ;
#21241=DIRECTION ( 'NONE',  ( 0.000000000000000000, 0.000000000000000000, 1.000000000000000000 ) ) ;
#21251=AXIS2_PLACEMENT_3D ( 'NONE', #10241, #23032, #14091 ) ;
#21253=EDGE_LOOP ( 'NONE', ( #28368, #1149, #22641, #11045 ) ) ;
#21256=ADVANCED_FACE ( 'NONE', ( #12525 ), #6610, .F. ) ;
#21266=DIRECTION ( 'NONE',  ( 1.000000000000000000, 0.000000000000000000, 0.000000000000000000 ) ) ;
#21278=ORIENTED_EDGE ( 'NONE', *, *, #17215, .F. ) ;
#21287=CARTESIAN_POINT ( 'NONE',  ( 10.80697542085375140, 31.15003855377755571, 13.00000000000000178 ) ) ;
#21296=ORIENTED_EDGE ( 'NONE', *, *, #31835, .F. ) ;
#21301=EDGE_LOOP ( 'NONE', ( #16178, #13554 ) ) ;
#21308=AXIS2_PLACEMENT_3D ( 'NONE', #6249, #12548, #15794 ) ;
#21337=CARTESIAN_POINT ( 'NONE',  ( 10.16520467992603294, 20.33931832809677331, 13.00000000000000178 ) ) ;
#21339=VECTOR ( 'NONE', #10705, 1000.000000000000000 ) ;
#21345=CARTESIAN_POINT ( 'NONE',  ( -2.247473515615844075, 16.63111439559750693, 13.00000000000000178 ) ) ;
#21346=AXIS2_PLACEMENT_3D ( 'NONE', #5118, #39637, #23607 ) ;
#21349=CARTESIAN_POINT ( 'NONE',  ( -6.953812613386785912, 14.77701242934787906, 6.000000000000000000 ) ) ;
#21362=VECTOR ( 'NONE', #5723, 1000.000000000000000 ) ;
#21370=CARTESIAN_POINT ( 'NONE',  ( 0.2655024426717602637, 36.24516302788250499, 13.00000000000000178 ) ) ;
#21377=ORIENTED_EDGE ( 'NONE', *, *, #5810, .F. ) ;
#21379=CARTESIAN_POINT ( 'NONE',  ( 3.835130509701798918, 15.55077355964573904, 6.000000000000000000 ) ) ;
#21386=EDGE_LOOP ( 'NONE', ( #16388, #20356 ) ) ;
#21390=ADVANCED_FACE ( 'NONE', ( #4580 ), #38302, .F. ) ;
#21395=AXIS2_PLACEMENT_3D ( 'NONE', #31998, #25695, #25895 ) ;
#21402=DIRECTION ( 'NONE',  ( 1.000000000000000000, 0.000000000000000000, 0.000000000000000000 ) ) ;
#21411=DIRECTION ( 'NONE',  ( 0.000000000000000000, 0.000000000000000000, 1.000000000000000000 ) ) ;
#21415=VECTOR ( 'NONE', #22006, 1000.000000000000000 ) ;
#21422=DIRECTION ( 'NONE',  ( 0.000000000000000000, 0.000000000000000000, 1.000000000000000000 ) ) ;
#21423=AXIS2_PLACEMENT_3D ( 'NONE', #35652, #29755, #20818 ) ;
#21424=VERTEX_POINT ( 'NONE', #18588 ) ;
#21439=ORIENTED_EDGE ( 'NONE', *, *, #17587, .T. ) ;
#21441=EDGE_CURVE ( 'NONE', #2121, #30551, #39516, .T. ) ;
#21452=LINE ( 'NONE', #6008, #24042 ) ;
#21458=EDGE_CURVE ( 'NONE', #27468, #20584, #17806, .T. ) ;
#21465=ORIENTED_EDGE ( 'NONE', *, *, #13287, .F. ) ;
#21468=CARTESIAN_POINT ( 'NONE',  ( -4.440836655099179353, 34.39106106163288246, 6.000000000000000000 ) ) ;
#21485=ORIENTED_EDGE ( 'NONE', *, *, #16613, .F. ) ;
#21499=DIRECTION ( 'NONE',  ( 0.000000000000000000, 0.000000000000000000, 1.000000000000000000 ) ) ;
#21513=ORIENTED_EDGE ( 'NONE', *, *, #18911, .F. ) ;
#21521=APPLICATION_CONTEXT ( 'automotive_design' ) ;
#21528=ADVANCED_FACE ( 'NONE', ( #39908 ), #33643, .F. ) ;
#21537=ORIENTED_EDGE ( 'NONE', *, *, #23296, .F. ) ;
#21550=CIRCLE ( 'NONE', #9227, 16.00000000000000000 ) ;
#21554=EDGE_CURVE ( 'NONE', #39380, #19863, #30181, .T. ) ;
#21557=EDGE_CURVE ( 'NONE', #26271, #37740, #25707, .T. ) ;
#21575=EDGE_CURVE ( 'NONE', #5290, #5502, #31172, .T. ) ;
#21576=DIRECTION ( 'NONE',  ( 1.000000000000000000, 0.000000000000000000, 0.000000000000000000 ) ) ;
#21587=ORIENTED_EDGE ( 'NONE', *, *, #16116, .T. ) ;
#21596=CYLINDRICAL_SURFACE ( 'NONE', #27784, 1.000000000000000000 ) ;
#21598=CARTESIAN_POINT ( 'NONE',  ( 0.000000000000000000, 22.50000000000000355, 13.00000000000000178 ) ) ;
#21600=VECTOR ( 'NONE', #15762, 1000.000000000000000 ) ;
#21601=FACE_BOUND ( 'NONE', #19845, .T. ) ;
#21603=ORIENTED_EDGE ( 'NONE', *, *, #31342, .F. ) ;
#21606=DIRECTION ( 'NONE',  ( 0.000000000000000000, 0.000000000000000000, 1.000000000000000000 ) ) ;
#21618=DIRECTION ( 'NONE',  ( 1.000000000000000000, 0.000000000000000000, 0.000000000000000000 ) ) ;
#21619=VERTEX_POINT ( 'NONE', #22212 ) ;
#21632=CARTESIAN_POINT ( 'NONE',  ( -2.211402178667006169, 32.38366924255629442, 13.00000000000000178 ) ) ;
#21633=DIRECTION ( 'NONE',  ( -1.000000000000000000, 0.000000000000000000, 0.000000000000000000 ) ) ;
#21637=AXIS2_PLACEMENT_3D ( 'NONE', #14117, #11678, #29354 ) ;
#21642=EDGE_LOOP ( 'NONE', ( #18627, #23500, #22186, #29471 ) ) ;
#21660=ORIENTED_EDGE ( 'NONE', *, *, #4916, .T. ) ;
#21665=CARTESIAN_POINT ( 'NONE',  ( 1.623731701744046241, 25.43444280220171194, 6.000000000000000000 ) ) ;
#21667=EDGE_CURVE ( 'NONE', #3856, #2749, #348, .T. ) ;
#21688=ORIENTED_EDGE ( 'NONE', *, *, #17692, .T. ) ;
#21691=DIRECTION ( 'NONE',  ( 1.000000000000000000, 0.000000000000000000, 0.000000000000000000 ) ) ;
#21692=ADVANCED_FACE ( 'NONE', ( #18783 ), #893, .F. ) ;
#21695=AXIS2_PLACEMENT_3D ( 'NONE', #2483, #34506, #37946 ) ;
#21697=DIRECTION ( 'NONE',  ( 1.000000000000000000, 0.000000000000000000, 0.000000000000000000 ) ) ;
#21698=ORIENTED_EDGE ( 'NONE', *, *, #13303, .T. ) ;
#21707=EDGE_CURVE ( 'NONE', #7, #12173, #3534, .T. ) ;
#21723=ORIENTED_EDGE ( 'NONE', *, *, #37893, .T. ) ;
#21726=DIRECTION ( 'NONE',  ( 0.000000000000000000, 0.000000000000000000, 1.000000000000000000 ) ) ;
#21733=ORIENTED_EDGE ( 'NONE', *, *, #14080, .T. ) ;
#21736=ORIENTED_EDGE ( 'NONE', *, *, #24916, .T. ) ;
#21738=AXIS2_PLACEMENT_3D ( 'NONE', #23507, #22895, #28998 ) ;
#21742=LINE ( 'NONE', #18708, #30073 ) ;
#21746=VERTEX_POINT ( 'NONE', #34422 ) ;
#21750=CARTESIAN_POINT ( 'NONE',  ( 11.03640989728592281, 29.14264673470096767, 6.000000000000000000 ) ) ;
#21751=ADVANCED_FACE ( 'NONE', ( #3729 ), #16132, .F. ) ;
#21759=ORIENTED_EDGE ( 'NONE', *, *, #34725, .T. ) ;
#21776=ORIENTED_EDGE ( 'NONE', *, *, #11156, .T. ) ;
#21788=EDGE_LOOP ( 'NONE', ( #11198, #37021 ) ) ;
#21795=VECTOR ( 'NONE', #35917, 1000.000000000000000 ) ;
#21821=AXIS2_PLACEMENT_3D ( 'NONE', #24871, #37265, #31170 ) ;
#21822=VERTEX_POINT ( 'NONE', #4335 ) ;
#21827=ORIENTED_EDGE ( 'NONE', *, *, #1889, .T. ) ;
#21832=DIRECTION ( 'NONE',  ( 1.000000000000000000, 0.000000000000000000, 0.000000000000000000 ) ) ;
#21833=VERTEX_POINT ( 'NONE', #35825 ) ;
#21835=ADVANCED_FACE ( 'NONE', ( #20189 ), #4540, .F. ) ;
#21839=ORIENTED_EDGE ( 'NONE', *, *, #1523, .T. ) ;
#21842=ORIENTED_EDGE ( 'NONE', *, *, #29360, .F. ) ;
#21852=CARTESIAN_POINT ( 'NONE',  ( 8.577540944421576441, 33.15743037285414374, 13.00000000000000178 ) ) ;
#21856=DIRECTION ( 'NONE',  ( 0.000000000000000000, 0.000000000000000000, 1.000000000000000000 ) ) ;
#21858=DIRECTION ( 'NONE',  ( 0.000000000000000000, 0.000000000000000000, 1.000000000000000000 ) ) ;
#21859=VERTEX_POINT ( 'NONE', #11244 ) ;
#21876=ORIENTED_EDGE ( 'NONE', *, *, #26893, .T. ) ;
#21885=EDGE_CURVE ( 'NONE', #25935, #5003, #35379, .T. ) ;
#21886=AXIS2_PLACEMENT_3D ( 'NONE', #31581, #10454, #10053 ) ;
#21896=CARTESIAN_POINT ( 'NONE',  ( 3.494936919103933448, 34.23777120880591696, 12.00000000000000000 ) ) ;
#21897=ORIENTED_EDGE ( 'NONE', *, *, #33979, .F. ) ;
#21906=ORIENTED_EDGE ( 'NONE', *, *, #19798, .T. ) ;
#21915=DIRECTION ( 'NONE',  ( 1.000000000000000000, 0.000000000000000000, 0.000000000000000000 ) ) ;
#21937=ORIENTED_EDGE ( 'NONE', *, *, #6314, .T. ) ;
#21941=EDGE_CURVE ( 'NONE', #9948, #20919, #6254, .T. ) ;
#21951=ORIENTED_EDGE ( 'NONE', *, *, #28700, .F. ) ;
#21962=DIRECTION ( 'NONE',  ( 0.000000000000000000, 0.000000000000000000, 1.000000000000000000 ) ) ;
#21975=FACE_BOUND ( 'NONE', #5498, .T. ) ;
#21984=ORIENTED_EDGE ( 'NONE', *, *, #17735, .F. ) ;
#21995=DIRECTION ( 'NONE',  ( 0.000000000000000000, 0.000000000000000000, 1.000000000000000000 ) ) ;
#22000=VECTOR ( 'NONE', #35954, 1000.000000000000000 ) ;
#22002=FACE_BOUND ( 'NONE', #29245, .T. ) ;
#22006=DIRECTION ( 'NONE',  ( 0.000000000000000000, 0.000000000000000000, 1.000000000000000000 ) ) ;
#22008=CARTESIAN_POINT ( 'NONE',  ( -5.458872323573595864, 26.51478363815348160, 13.00000000000000178 ) ) ;
#22016=EDGE_LOOP ( 'NONE', ( #22550, #21698, #12033, #30091 ) ) ;
#22020=DIRECTION ( 'NONE',  ( 0.000000000000000000, 0.000000000000000000, 1.000000000000000000 ) ) ;
#22032=CARTESIAN_POINT ( 'NONE',  ( -11.16521142134453726, 24.66068167190384841, 13.00000000000000178 ) ) ;
#22052=CARTESIAN_POINT ( 'NONE',  ( -14.01838097023000707, 23.73363068877903359, 13.00000000000000178 ) ) ;
#22054=EDGE_CURVE ( 'NONE', #15741, #10198, #11399, .T. ) ;
#22063=FACE_OUTER_BOUND ( 'NONE', #33639, .T. ) ;
#22069=ORIENTED_EDGE ( 'NONE', *, *, #4519, .F. ) ;
#22073=CIRCLE ( 'NONE', #2622, 1.000000000000000000 ) ;
#22082=ORIENTED_EDGE ( 'NONE', *, *, #35406, .T. ) ;
#22087=EDGE_CURVE ( 'NONE', #32396, #39920, #36236, .T. ) ;
#22096=VERTEX_POINT ( 'NONE', #8398 ) ;
#22102=AXIS2_PLACEMENT_3D ( 'NONE', #23106, #1175, #19451 ) ;
#22109=ORIENTED_EDGE ( 'NONE', *, *, #37398, .F. ) ;
#22113=LINE ( 'NONE', #25758, #6155 ) ;
#22114=EDGE_CURVE ( 'NONE', #6485, #24101, #20794, .T. ) ;
#22135=ORIENTED_EDGE ( 'NONE', *, *, #8143, .T. ) ;
#22137=DIRECTION ( 'NONE',  ( 0.000000000000000000, 0.000000000000000000, 1.000000000000000000 ) ) ;
#22140=ORIENTED_EDGE ( 'NONE', *, *, #38040, .T. ) ;
#22146=ORIENTED_EDGE ( 'NONE', *, *, #5916, .F. ) ;
#22154=VECTOR ( 'NONE', #37597, 1000.000000000000000 ) ;
#22158=CARTESIAN_POINT ( 'NONE',  ( -2.605702774688126500, 27.44183462127829642, 12.00000000000000000 ) ) ;
#22159=ORIENTED_EDGE ( 'NONE', *, *, #17587, .F. ) ;
#22166=ADVANCED_FACE ( 'NONE', ( #19129, #37417, #12829, #6526, #28069, #6921, #22567, #22365, #9391, #3885, #19325, #9591, #37623, #34176, #30928, #3091, #3686, #25225, #3488, #6132, #28669, #27873, #28469, #31721, #247, #844, #12431, #25023, #34570, #3289, #12634, #15681, #18537, #16081, #34772, #21975, #13223, #9791, #6720, #34376, #18931, #25615, #38015, #15487, #37814, #24823, #37221, #6326, #18737, #644, #31126, #31319, #15885, #31523, #13025, #25416, #35780, #11194, #11000, #38221, #32737, #7933, #32540, #31917, #1857, #16690, #4694, #7737, #13632, #23384, #16487, #22768, #28873, #17099, #20344, #14236, #29072, #29474, #20140, #26019, #4893, #7127, #25821, #14034, #38618, #39017 ), #1651, .T. ) ;
#22168=EDGE_LOOP ( 'NONE', ( #5525, #11168 ) ) ;
#22177=DIRECTION ( 'NONE',  ( 1.000000000000000000, 0.000000000000000000, 0.000000000000000000 ) ) ;
#22178=LINE ( 'NONE', #31134, #15394 ) ;
#22185=EDGE_CURVE ( 'NONE', #2515, #9387, #26425, .T. ) ;
#22186=ORIENTED_EDGE ( 'NONE', *, *, #31257, .T. ) ;
#22187=EDGE_CURVE ( 'NONE', #23393, #30574, #15276, .T. ) ;
#22191=DIRECTION ( 'NONE',  ( 0.000000000000000000, 0.000000000000000000, 1.000000000000000000 ) ) ;
#22197=CARTESIAN_POINT ( 'NONE',  ( -10.16521142134453548, 24.66068167190384841, 12.00000000000000000 ) ) ;
#22207=CARTESIAN_POINT ( 'NONE',  ( 11.39463915635820612, 18.33192650902018883, 13.00000000000000178 ) ) ;
#22212=CARTESIAN_POINT ( 'NONE',  ( 18.00000000000000000, 22.50000000000000711, 6.000000000000000000 ) ) ;
#22229=ORIENTED_EDGE ( 'NONE', *, *, #5019, .F. ) ;
#22234=ORIENTED_EDGE ( 'NONE', *, *, #11141, .F. ) ;
#22242=AXIS2_PLACEMENT_3D ( 'NONE', #10027, #35418, #38461 ) ;
#22244=FACE_OUTER_BOUND ( 'NONE', #4293, .T. ) ;
#22246=EDGE_CURVE ( 'NONE', #36663, #15234, #34977, .T. ) ;
#22261=DIRECTION ( 'NONE',  ( 1.000000000000000000, 0.000000000000000000, 0.000000000000000000 ) ) ;
#22278=CARTESIAN_POINT ( 'NONE',  ( -11.41268156625113406, 18.79179606750104981, 6.000000000000000000 ) ) ;
#22287=CIRCLE ( 'NONE', #8669, 1.000000000000000000 ) ;
#22288=EDGE_LOOP ( 'NONE', ( #10310, #1409 ) ) ;
#22289=ORIENTED_EDGE ( 'NONE', *, *, #9993, .F. ) ;
#22292=DIRECTION ( 'NONE',  ( 1.000000000000000000, 0.000000000000000000, 0.000000000000000000 ) ) ;
#22293=VERTEX_POINT ( 'NONE', #17902 ) ;
#22294=AXIS2_PLACEMENT_3D ( 'NONE', #39292, #1933, #29347 ) ;
#22299=CARTESIAN_POINT ( 'NONE',  ( 6.706335727061685681, 24.35410196624994583, 12.00000000000000000 ) ) ;
#22300=EDGE_CURVE ( 'NONE', #36787, #4871, #31490, .T. ) ;
#22301=CARTESIAN_POINT ( 'NONE',  ( -4.082607396026893376, 23.58034083595207875, 6.000000000000000000 ) ) ;
#22302=CIRCLE ( 'NONE', #21013, 1.000000000000000000 ) ;
#22307=DIRECTION ( 'NONE',  ( 1.000000000000000000, 0.000000000000000000, 0.000000000000000000 ) ) ;
#22311=DIRECTION ( 'NONE',  ( 0.000000000000000000, 0.000000000000000000, 1.000000000000000000 ) ) ;
#22322=ORIENTED_EDGE ( 'NONE', *, *, #12742, .T. ) ;
#22325=ORIENTED_EDGE ( 'NONE', *, *, #25141, .T. ) ;
#22327=DIRECTION ( 'NONE',  ( 1.000000000000000000, 0.000000000000000000, 0.000000000000000000 ) ) ;
#22329=VERTEX_POINT ( 'NONE', #24179 ) ;
#22331=DIRECTION ( 'NONE',  ( 0.000000000000000000, 0.000000000000000000, 1.000000000000000000 ) ) ;
#22341=DIRECTION ( 'NONE',  ( 1.000000000000000000, 0.000000000000000000, 0.000000000000000000 ) ) ;
#22346=CARTESIAN_POINT ( 'NONE',  ( -8.806982162272252168, 13.84996144622306247, 13.00000000000000178 ) ) ;
#22362=AXIS2_PLACEMENT_3D ( 'NONE', #34858, #19406, #3966 ) ;
#22365=FACE_BOUND ( 'NONE', #13329, .T. ) ;
#22373=VERTEX_POINT ( 'NONE', #39218 ) ;
#22375=ORIENTED_EDGE ( 'NONE', *, *, #21667, .T. ) ;
#22390=VECTOR ( 'NONE', #12510, 1000.000000000000000 ) ;
#22391=VECTOR ( 'NONE', #1251, 1000.000000000000000 ) ;
#22392=FACE_BOUND ( 'NONE', #23978, .T. ) ;
#22393=CYLINDRICAL_SURFACE ( 'NONE', #28931, 1.000000000000000000 ) ;
#22401=EDGE_CURVE ( 'NONE', #30063, #28113, #2649, .T. ) ;
#22402=DIRECTION ( 'NONE',  ( 0.000000000000000000, 0.000000000000000000, 1.000000000000000000 ) ) ;
#22404=VERTEX_POINT ( 'NONE', #14433 ) ;
#22417=EDGE_LOOP ( 'NONE', ( #21171, #11549, #1307, #38047 ) ) ;
#22426=VECTOR ( 'NONE', #27372, 1000.000000000000000 ) ;
#22430=ADVANCED_FACE ( 'NONE', ( #39814 ), #23585, .F. ) ;
#22434=EDGE_CURVE ( 'NONE', #14560, #23343, #3588, .T. ) ;
#22441=DIRECTION ( 'NONE',  ( 0.000000000000000000, 0.000000000000000000, 1.000000000000000000 ) ) ;
#22445=DIRECTION ( 'NONE',  ( 0.000000000000000000, 0.000000000000000000, 1.000000000000000000 ) ) ;
#22452=CIRCLE ( 'NONE', #432, 1.000000000000000888 ) ;
#22455=AXIS2_PLACEMENT_3D ( 'NONE', #19780, #1495, #20596 ) ;
#22456=EDGE_CURVE ( 'NONE', #16724, #4132, #19836, .T. ) ;
#22474=ORIENTED_EDGE ( 'NONE', *, *, #32151, .F. ) ;
#22480=EDGE_CURVE ( 'NONE', #15244, #31324, #35402, .T. ) ;
#22483=AXIS2_PLACEMENT_3D ( 'NONE', #27230, #24178, #21134 ) ;
#22484=CIRCLE ( 'NONE', #27685, 1.000000000000000000 ) ;
#22489=DIRECTION ( 'NONE',  ( -0.000000000000000000, -0.000000000000000000, -1.000000000000000000 ) ) ;
#22490=EDGE_LOOP ( 'NONE', ( #39972, #34088, #19024, #25400 ) ) ;
#22492=CARTESIAN_POINT ( 'NONE',  ( -7.935776944912362296, 22.65328985282726393, 6.000000000000000000 ) ) ;
#22494=DIRECTION ( 'NONE',  ( 1.000000000000000000, 0.000000000000000000, 0.000000000000000000 ) ) ;
#22495=DIRECTION ( 'NONE',  ( 0.000000000000000000, 0.000000000000000000, 1.000000000000000000 ) ) ;
#22501=CARTESIAN_POINT ( 'NONE',  ( 0.000000000000000000, 22.50000000000000355, 6.000000000000000000 ) ) ;
#22526=CARTESIAN_POINT ( 'NONE',  ( -11.41268156625113406, 18.79179606750104981, 13.00000000000000178 ) ) ;
#22538=AXIS2_PLACEMENT_3D ( 'NONE', #9450, #25280, #34430 ) ;
#22550=ORIENTED_EDGE ( 'NONE', *, *, #1768, .F. ) ;
#22561=DIRECTION ( 'NONE',  ( 1.000000000000000000, 0.000000000000000000, 0.000000000000000000 ) ) ;
#22562=EDGE_LOOP ( 'NONE', ( #16707, #27030, #11116, #32142 ) ) ;
#22567=FACE_BOUND ( 'NONE', #21225, .T. ) ;
#22575=CARTESIAN_POINT ( 'NONE',  ( 1.358225888363031819, 11.68927977431952137, 13.00000000000000178 ) ) ;
#22586=EDGE_CURVE ( 'NONE', #14121, #4988, #32811, .T. ) ;
#22589=CARTESIAN_POINT ( 'NONE',  ( 2.494936919103933448, 34.23777120880591696, 6.000000000000000000 ) ) ;
#22592=DIRECTION ( 'NONE',  ( 0.000000000000000000, 0.000000000000000000, 1.000000000000000000 ) ) ;
#22593=AXIS2_PLACEMENT_3D ( 'NONE', #15399, #11754, #18256 ) ;
#22595=FACE_BOUND ( 'NONE', #1612, .T. ) ;
#22600=CARTESIAN_POINT ( 'NONE',  ( 4.348106467989403257, 35.16482219193073178, 13.00000000000000178 ) ) ;
#22603=AXIS2_PLACEMENT_3D ( 'NONE', #22278, #34683, #26133 ) ;
#22611=ADVANCED_FACE ( 'NONE', ( #24582 ), #18492, .F. ) ;
#22613=ORIENTED_EDGE ( 'NONE', *, *, #15719, .T. ) ;
#22618=ORIENTED_EDGE ( 'NONE', *, *, #28935, .T. ) ;
#22626=DIRECTION ( 'NONE',  ( 0.000000000000000000, 0.000000000000000000, 1.000000000000000000 ) ) ;
#22636=EDGE_CURVE ( 'NONE', #37407, #2419, #25641, .T. ) ;
#22637=LINE ( 'NONE', #19393, #35349 ) ;
#22641=ORIENTED_EDGE ( 'NONE', *, *, #26286, .T. ) ;
#22642=DIRECTION ( 'NONE',  ( 1.000000000000000000, 0.000000000000000000, 0.000000000000000000 ) ) ;
#22648=CARTESIAN_POINT ( 'NONE',  ( -6.064571727552472424, 31.45661825943146894, 13.00000000000000178 ) ) ;
#22649=AXIS2_PLACEMENT_3D ( 'NONE', #28548, #31796, #18816 ) ;
#22659=AXIS2_PLACEMENT_3D ( 'NONE', #24199, #20770, #33164 ) ;
#22661=EDGE_LOOP ( 'NONE', ( #2224, #20094, #8277, #35591 ) ) ;
#22681=CARTESIAN_POINT ( 'NONE',  ( 10.14716901145161465, 12.46304090461738667, 6.000000000000000000 ) ) ;
#22686=ADVANCED_FACE ( 'NONE', ( #36091 ), #17413, .F. ) ;
#22690=CARTESIAN_POINT ( 'NONE',  ( 10.78893975237932956, 23.27376113029817617, 12.00000000000000000 ) ) ;
#22693=ORIENTED_EDGE ( 'NONE', *, *, #3800, .T. ) ;
#22701=CARTESIAN_POINT ( 'NONE',  ( 1.605696033269625955, 17.55816537872232530, 12.00000000000000000 ) ) ;
#22718=EDGE_LOOP ( 'NONE', ( #35079, #20866, #25460, #26716 ) ) ;
#22723=ORIENTED_EDGE ( 'NONE', *, *, #20058, .F. ) ;
#22727=ORIENTED_EDGE ( 'NONE', *, *, #40040, .F. ) ;
#22739=EDGE_CURVE ( 'NONE', #40053, #17409, #12813, .T. ) ;
#22741=CYLINDRICAL_SURFACE ( 'NONE', #17501, 1.000000000000000000 ) ;
#22749=EDGE_LOOP ( 'NONE', ( #27264, #3822, #11393, #39654, #5466, #10287 ) ) ;
#22754=CARTESIAN_POINT ( 'NONE',  ( 12.39463915635820612, 18.33192650902018883, 13.00000000000000178 ) ) ;
#22756=VERTEX_POINT ( 'NONE', #17207 ) ;
#22758=AXIS2_PLACEMENT_3D ( 'NONE', #27853, #19502, #624 ) ;
#22765=VERTEX_POINT ( 'NONE', #7641 ) ;
#22768=FACE_BOUND ( 'NONE', #19164, .T. ) ;
#22769=EDGE_CURVE ( 'NONE', #24692, #21186, #39438, .T. ) ;
#22782=CARTESIAN_POINT ( 'NONE',  ( -1.587667106213708879, 35.31811204475769728, 12.00000000000000000 ) ) ;
#22787=EDGE_CURVE ( 'NONE', #33978, #32396, #10884, .T. ) ;
#22793=DIRECTION ( 'NONE',  ( 0.000000000000000000, 0.000000000000000000, 1.000000000000000000 ) ) ;
#22796=FACE_BOUND ( 'NONE', #33000, .T. ) ;
#22803=EDGE_CURVE ( 'NONE', #3779, #32505, #5050, .T. ) ;
#22805=ORIENTED_EDGE ( 'NONE', *, *, #14308, .T. ) ;
#22809=LINE ( 'NONE', #3720, #32835 ) ;
#22814=CARTESIAN_POINT ( 'NONE',  ( -10.80698216227225394, 13.84996144622306247, 13.00000000000000178 ) ) ;
#22821=ORIENTED_EDGE ( 'NONE', *, *, #29947, .F. ) ;
#22826=ORIENTED_EDGE ( 'NONE', *, *, #10476, .T. ) ;
#22829=CYLINDRICAL_SURFACE ( 'NONE', #21251, 1.000000000000000000 ) ;
#22834=VERTEX_POINT ( 'NONE', #2367 ) ;
#22839=DIRECTION ( 'NONE',  ( 0.000000000000000000, 0.000000000000000000, 1.000000000000000000 ) ) ;
#22842=DIRECTION ( 'NONE',  ( 0.000000000000000000, 0.000000000000000000, 1.000000000000000000 ) ) ;
#22849=CARTESIAN_POINT ( 'NONE',  ( -13.03641663870442891, 15.85735326529964873, 13.00000000000000178 ) ) ;
#22852=SURFACE_STYLE_USAGE ( .BOTH. , #26313 ) ;
#22871=EDGE_LOOP ( 'NONE', ( #34097, #18753 ) ) ;
#22883=CIRCLE ( 'NONE', #5377, 1.000000000000000000 ) ;
#22890=CIRCLE ( 'NONE', #13177, 1.000000000000000000 ) ;
#22895=DIRECTION ( 'NONE',  ( 0.000000000000000000, 0.000000000000000000, 1.000000000000000000 ) ) ;
#22923=FACE_OUTER_BOUND ( 'NONE', #3255, .T. ) ;
#22924=EDGE_CURVE ( 'NONE', #15493, #27371, #34252, .T. ) ;
#22929=CIRCLE ( 'NONE', #14525, 1.000000000000000000 ) ;
#22934=DIRECTION ( 'NONE',  ( 0.000000000000000000, 0.000000000000000000, 1.000000000000000000 ) ) ;
#22939=AXIS2_PLACEMENT_3D ( 'NONE', #20013, #23856, #8214 ) ;
#22943=DIRECTION ( 'NONE',  ( 0.000000000000000000, 0.000000000000000000, 1.000000000000000000 ) ) ;
#22945=EDGE_CURVE ( 'NONE', #15085, #20641, #26447, .T. ) ;
#22950=DIRECTION ( 'NONE',  ( 0.000000000000000000, 0.000000000000000000, 1.000000000000000000 ) ) ;
#22952=DIRECTION ( 'NONE',  ( 0.000000000000000000, 0.000000000000000000, 1.000000000000000000 ) ) ;
#22955=AXIS2_PLACEMENT_3D ( 'NONE', #2815, #8317, #36544 ) ;
#22962=VERTEX_POINT ( 'NONE', #15146 ) ;
#22964=AXIS2_PLACEMENT_3D ( 'NONE', #14671, #39446, #3419 ) ;
#22981=ORIENTED_EDGE ( 'NONE', *, *, #7559, .T. ) ;
#22983=CARTESIAN_POINT ( 'NONE',  ( 0.2655024426717602637, 36.24516302788250499, 12.00000000000000000 ) ) ;
#23004=AXIS2_PLACEMENT_3D ( 'NONE', #36396, #8559, #20954 ) ;
#23008=ORIENTED_EDGE ( 'NONE', *, *, #6746, .F. ) ;
#23016=CARTESIAN_POINT ( 'NONE',  ( 1.587660364795204782, 9.681887955242936883, 12.00000000000000000 ) ) ;
#23027=CARTESIAN_POINT ( 'NONE',  ( 10.80697542085375140, 31.15003855377755571, 12.00000000000000000 ) ) ;
#23032=DIRECTION ( 'NONE',  ( 0.000000000000000000, 0.000000000000000000, 1.000000000000000000 ) ) ;
#23038=ORIENTED_EDGE ( 'NONE', *, *, #18265, .T. ) ;
#23042=EDGE_CURVE ( 'NONE', #19485, #15842, #9607, .T. ) ;
#23043=DIRECTION ( 'NONE',  ( 1.000000000000000000, 0.000000000000000000, 0.000000000000000000 ) ) ;
#23045=AXIS2_PLACEMENT_3D ( 'NONE', #14893, #27080, #33588 ) ;
#23051=CYLINDRICAL_SURFACE ( 'NONE', #4254, 1.000000000000000888 ) ;
#23054=CARTESIAN_POINT ( 'NONE',  ( -4.458872323573595864, 26.51478363815348160, 6.000000000000000000 ) ) ;
#23056=CARTESIAN_POINT ( 'NONE',  ( -0.6417741116369681809, 11.68927977431952137, 12.00000000000000000 ) ) ;
#23060=ORIENTED_EDGE ( 'NONE', *, *, #31114, .T. ) ;
#23068=EDGE_LOOP ( 'NONE', ( #19644, #5415 ) ) ;
#23071=DIRECTION ( 'NONE',  ( 0.000000000000000000, 0.000000000000000000, 1.000000000000000000 ) ) ;
#23077=AXIS2_PLACEMENT_3D ( 'NONE', #21337, #2849, #29872 ) ;
#23094=ADVANCED_FACE ( 'NONE', ( #6977 ), #4499, .F. ) ;
#23095=VERTEX_POINT ( 'NONE', #6583 ) ;
#23101=LINE ( 'NONE', #10309, #37612 ) ;
#23105=CIRCLE ( 'NONE', #8171, 1.000000000000000888 ) ;
#23106=CARTESIAN_POINT ( 'NONE',  ( -3.118678732975735279, 7.827785988993307242, 12.00000000000000000 ) ) ;
#23108=CARTESIAN_POINT ( 'NONE',  ( 7.293999462566144842, 11.53598992149257008, 6.000000000000000000 ) ) ;
#23126=DIRECTION ( 'NONE',  ( 0.000000000000000000, 0.000000000000000000, 1.000000000000000000 ) ) ;
#23131=ORIENTED_EDGE ( 'NONE', *, *, #17104, .F. ) ;
#23133=AXIS2_PLACEMENT_3D ( 'NONE', #36281, #4992, #7831 ) ;
#23134=DIRECTION ( 'NONE',  ( 0.000000000000000000, 0.000000000000000000, 1.000000000000000000 ) ) ;
#23139=EDGE_CURVE ( 'NONE', #31499, #9140, #19988, .T. ) ;
#23142=ORIENTED_EDGE ( 'NONE', *, *, #38037, .T. ) ;
#23154=EDGE_CURVE ( 'NONE', #21833, #8090, #2447, .T. ) ;
#23162=CARTESIAN_POINT ( 'NONE',  ( -0.6237384431625470071, 19.56555719779890978, 6.000000000000000000 ) ) ;
#23164=CYLINDRICAL_SURFACE ( 'NONE', #8070, 1.000000000000000000 ) ;
#23173=EDGE_LOOP ( 'NONE', ( #35821, #4904, #34560, #28029 ) ) ;
#23187=EDGE_CURVE ( 'NONE', #38979, #6441, #13476, .T. ) ;
#23216=CARTESIAN_POINT ( 'NONE',  ( -9.165211421344535481, 24.66068167190384841, 12.00000000000000000 ) ) ;
#23219=CIRCLE ( 'NONE', #25157, 1.000000000000000888 ) ;
#23226=EDGE_LOOP ( 'NONE', ( #1339, #18307 ) ) ;
#23228=ORIENTED_EDGE ( 'NONE', *, *, #4583, .F. ) ;
#23229=AXIS2_PLACEMENT_3D ( 'NONE', #24647, #24448, #36841 ) ;
#23244=CARTESIAN_POINT ( 'NONE',  ( 1.981960960816328887, 14.62372257652092422, 6.000000000000000000 ) ) ;
#23266=CARTESIAN_POINT ( 'NONE',  ( -0.2655091840902661926, 8.754836972118123839, 12.00000000000000000 ) ) ;
#23288=EDGE_LOOP ( 'NONE', ( #29638, #28580 ) ) ;
#23296=EDGE_CURVE ( 'NONE', #10818, #17668, #11403, .T. ) ;
#23300=DIRECTION ( 'NONE',  ( 0.000000000000000000, 0.000000000000000000, 1.000000000000000000 ) ) ;
#23304=ORIENTED_EDGE ( 'NONE', *, *, #16325, .F. ) ;
#23309=CIRCLE ( 'NONE', #36942, 1.000000000000000000 ) ;
#23310=AXIS2_PLACEMENT_3D ( 'NONE', #15363, #21068, #27755 ) ;
#23311=FACE_OUTER_BOUND ( 'NONE', #35470, .T. ) ;
#23316=CIRCLE ( 'NONE', #5803, 1.000000000000000000 ) ;
#23318=CARTESIAN_POINT ( 'NONE',  ( -5.458872323573595864, 26.51478363815348160, 12.00000000000000000 ) ) ;
#23319=DIRECTION ( 'NONE',  ( 0.000000000000000000, 0.000000000000000000, 1.000000000000000000 ) ) ;
#23330=DIRECTION ( 'NONE',  ( 0.000000000000000000, 0.000000000000000000, 1.000000000000000000 ) ) ;
#23342=DIRECTION ( 'NONE',  ( 0.000000000000000000, 0.000000000000000000, 1.000000000000000000 ) ) ;
#23343=VERTEX_POINT ( 'NONE', #17907 ) ;
#23357=FACE_OUTER_BOUND ( 'NONE', #11447, .T. ) ;
#23362=CARTESIAN_POINT ( 'NONE',  ( 5.440829913680675034, 10.60893893836775348, 6.000000000000000000 ) ) ;
#23368=EDGE_LOOP ( 'NONE', ( #15862, #23751 ) ) ;
#23369=CARTESIAN_POINT ( 'NONE',  ( 1.229431105722923023, 20.49260818092372460, 12.00000000000000000 ) ) ;
#23373=CIRCLE ( 'NONE', #14296, 1.000000000000000000 ) ;
#23381=ORIENTED_EDGE ( 'NONE', *, *, #867, .F. ) ;
#23383=DIRECTION ( 'NONE',  ( 1.000000000000000000, 0.000000000000000000, 0.000000000000000000 ) ) ;
#23384=FACE_BOUND ( 'NONE', #15011, .T. ) ;
#23387=CYLINDRICAL_SURFACE ( 'NONE', #2064, 1.000000000000000888 ) ;
#23393=VERTEX_POINT ( 'NONE', #33548 ) ;
#23401=VECTOR ( 'NONE', #7915, 1000.000000000000000 ) ;
#23403=DIRECTION ( 'NONE',  ( 1.000000000000000000, 0.000000000000000000, 0.000000000000000000 ) ) ;
#23407=ADVANCED_FACE ( 'NONE', ( #36780 ), #8951, .F. ) ;
#23408=CARTESIAN_POINT ( 'NONE',  ( 3.458865582155095986, 18.48521636184714012, 13.00000000000000178 ) ) ;
#23412=EDGE_CURVE ( 'NONE', #4988, #39486, #34286, .T. ) ;
#23419=DIRECTION ( 'NONE',  ( 0.000000000000000000, 0.000000000000000000, 1.000000000000000000 ) ) ;
#23424=DIRECTION ( 'NONE',  ( 1.000000000000000000, 0.000000000000000000, 0.000000000000000000 ) ) ;
#23434=ORIENTED_EDGE ( 'NONE', *, *, #35046, .F. ) ;
#23439=EDGE_LOOP ( 'NONE', ( #30945, #24627, #29007, #22375 ) ) ;
#23441=EDGE_CURVE ( 'NONE', #32004, #25935, #9554, .T. ) ;
#23442=DIRECTION ( 'NONE',  ( 0.000000000000000000, 0.000000000000000000, 1.000000000000000000 ) ) ;
#23449=CIRCLE ( 'NONE', #5920, 1.000000000000000000 ) ;
#23453=CARTESIAN_POINT ( 'NONE',  ( -5.440836655099179353, 34.39106106163288246, 13.00000000000000178 ) ) ;
#23454=DIRECTION ( 'NONE',  ( 0.000000000000000000, 0.000000000000000000, 1.000000000000000000 ) ) ;
#23455=EDGE_CURVE ( 'NONE', #3736, #6333, #3753, .T. ) ;
#23458=DIRECTION ( 'NONE',  ( 1.000000000000000000, 0.000000000000000000, 0.000000000000000000 ) ) ;
#23461=DIRECTION ( 'NONE',  ( 0.000000000000000000, 0.000000000000000000, 1.000000000000000000 ) ) ;
#23462=CARTESIAN_POINT ( 'NONE',  ( -13.26585111513660031, 17.86474508437623143, 13.00000000000000178 ) ) ;
#23464=DIRECTION ( 'NONE',  ( 0.000000000000000000, 0.000000000000000000, 1.000000000000000000 ) ) ;
#23467=ORIENTED_EDGE ( 'NONE', *, *, #2616, .T. ) ;
#23470=DIRECTION ( 'NONE',  ( 1.000000000000000000, 0.000000000000000000, 0.000000000000000000 ) ) ;
#23472=DIRECTION ( 'NONE',  ( 1.000000000000000000, 0.000000000000000000, 0.000000000000000000 ) ) ;
#23474=ORIENTED_EDGE ( 'NONE', *, *, #38334, .T. ) ;
#23475=FACE_OUTER_BOUND ( 'NONE', #8470, .T. ) ;
#23490=DIRECTION ( 'NONE',  ( 0.000000000000000000, 0.000000000000000000, 1.000000000000000000 ) ) ;
#23500=ORIENTED_EDGE ( 'NONE', *, *, #28583, .T. ) ;
#23507=CARTESIAN_POINT ( 'NONE',  ( 5.348106467989403257, 35.16482219193073178, 13.00000000000000178 ) ) ;
#23509=CIRCLE ( 'NONE', #26082, 1.000000000000000888 ) ;
#23510=EDGE_CURVE ( 'NONE', #7967, #27371, #24588, .T. ) ;
#23520=DIRECTION ( 'NONE',  ( 1.000000000000000000, 0.000000000000000000, 0.000000000000000000 ) ) ;
#23521=DIRECTION ( 'NONE',  ( 1.000000000000000000, 0.000000000000000000, 0.000000000000000000 ) ) ;
#23523=DIRECTION ( 'NONE',  ( 0.000000000000000000, 0.000000000000000000, 1.000000000000000000 ) ) ;
#23526=DIRECTION ( 'NONE',  ( 0.000000000000000000, 0.000000000000000000, 1.000000000000000000 ) ) ;
#23528=AXIS2_PLACEMENT_3D ( 'NONE', #38250, #10017, #28301 ) ;
#23536=ADVANCED_FACE ( 'NONE', ( #12392 ), #9, .F. ) ;
#23539=AXIS2_PLACEMENT_3D ( 'NONE', #12268, #18569, #30954 ) ;
#23541=ORIENTED_EDGE ( 'NONE', *, *, #21166, .T. ) ;
#23544=DIRECTION ( 'NONE',  ( 1.000000000000000000, 0.000000000000000000, 0.000000000000000000 ) ) ;
#23549=AXIS2_PLACEMENT_3D ( 'NONE', #4341, #6971, #28520 ) ;
#23550=ORIENTED_EDGE ( 'NONE', *, *, #23187, .F. ) ;
#23551=CARTESIAN_POINT ( 'NONE',  ( -6.953812613386785912, 14.77701242934787906, 6.000000000000000000 ) ) ;
#23560=ORIENTED_EDGE ( 'NONE', *, *, #13823, .F. ) ;
#23563=DIRECTION ( 'NONE',  ( 1.000000000000000000, 0.000000000000000000, 0.000000000000000000 ) ) ;
#23566=CIRCLE ( 'NONE', #857, 16.99999999999999645 ) ;
#23581=ORIENTED_EDGE ( 'NONE', *, *, #7637, .F. ) ;
#23584=AXIS2_PLACEMENT_3D ( 'NONE', #30166, #17589, #11281 ) ;
#23585=CYLINDRICAL_SURFACE ( 'NONE', #38621, 1.000000000000000888 ) ;
#23599=CIRCLE ( 'NONE', #25523, 1.000000000000000888 ) ;
#23606=VECTOR ( 'NONE', #21499, 1000.000000000000000 ) ;
#23607=DIRECTION ( 'NONE',  ( 1.000000000000000000, 0.000000000000000000, 0.000000000000000000 ) ) ;
#23609=EDGE_CURVE ( 'NONE', #35485, #2390, #28629, .T. ) ;
#23613=FACE_OUTER_BOUND ( 'NONE', #7956, .T. ) ;
#23614=CIRCLE ( 'NONE', #22294, 1.000000000000000888 ) ;
#23619=CARTESIAN_POINT ( 'NONE',  ( 4.458865582155095986, 18.48521636184714012, 13.00000000000000178 ) ) ;
#23622=ORIENTED_EDGE ( 'NONE', *, *, #27897, .T. ) ;
#23627=ORIENTED_EDGE ( 'NONE', *, *, #35344, .T. ) ;
#23631=CARTESIAN_POINT ( 'NONE',  ( -0.8712085880691411433, 13.69667159339610762, 12.00000000000000000 ) ) ;
#23635=VERTEX_POINT ( 'NONE', #13587 ) ;
#23642=FACE_OUTER_BOUND ( 'NONE', #10892, .T. ) ;
#23643=ORIENTED_EDGE ( 'NONE', *, *, #22185, .T. ) ;
#23646=VECTOR ( 'NONE', #14165, 1000.000000000000000 ) ;
#23649=EDGE_LOOP ( 'NONE', ( #1000, #609 ) ) ;
#23656=DIRECTION ( 'NONE',  ( 0.000000000000000000, 0.000000000000000000, 1.000000000000000000 ) ) ;
#23657=DIRECTION ( 'NONE',  ( 0.000000000000000000, 0.000000000000000000, 1.000000000000000000 ) ) ;
#23659=EDGE_LOOP ( 'NONE', ( #37980, #11203 ) ) ;
#23676=ORIENTED_EDGE ( 'NONE', *, *, #29294, .T. ) ;
#23678=DIRECTION ( 'NONE',  ( 0.000000000000000000, 0.000000000000000000, 1.000000000000000000 ) ) ;
#23681=AXIS2_PLACEMENT_3D ( 'NONE', #3188, #39956, #37117 ) ;
#23687=CARTESIAN_POINT ( 'NONE',  ( 3.587660364795204782, 9.681887955242936883, 12.00000000000000000 ) ) ;
#23688=CYLINDRICAL_SURFACE ( 'NONE', #30304, 1.000000000000000888 ) ;
#23691=VERTEX_POINT ( 'NONE', #4038 ) ;
#23706=CARTESIAN_POINT ( 'NONE',  ( 7.330070799514983193, 27.28854476845134513, 12.00000000000000000 ) ) ;
#23709=EDGE_CURVE ( 'NONE', #32281, #18451, #27151, .T. ) ;
#23712=AXIS2_PLACEMENT_3D ( 'NONE', #4378, #10076, #31605 ) ;
#23715=DIRECTION ( 'NONE',  ( 1.000000000000000000, 0.000000000000000000, 0.000000000000000000 ) ) ;
#23722=DIRECTION ( 'NONE',  ( 0.000000000000000000, 0.000000000000000000, 1.000000000000000000 ) ) ;
#23724=CARTESIAN_POINT ( 'NONE',  ( 7.577540944421576441, 33.15743037285414374, 13.00000000000000178 ) ) ;
#23732=LINE ( 'NONE', #27185, #10868 ) ;
#23738=ORIENTED_EDGE ( 'NONE', *, *, #9015, .F. ) ;
#23747=CIRCLE ( 'NONE', #10788, 1.000000000000000888 ) ;
#23748=VERTEX_POINT ( 'NONE', #10748 ) ;
#23751=ORIENTED_EDGE ( 'NONE', *, *, #28252, .T. ) ;
#23754=CARTESIAN_POINT ( 'NONE',  ( -4.211402178667006169, 32.38366924255629442, 13.00000000000000178 ) ) ;
#23757=CARTESIAN_POINT ( 'NONE',  ( 3.100636323082810009, 29.29593658752792962, 6.000000000000000000 ) ) ;
#23763=ORIENTED_EDGE ( 'NONE', *, *, #27671, .F. ) ;
#23767=CARTESIAN_POINT ( 'NONE',  ( 3.229431105722923245, 20.49260818092372460, 6.000000000000000000 ) ) ;
#23777=ORIENTED_EDGE ( 'NONE', *, *, #15452, .F. ) ;
#23782=DIRECTION ( 'NONE',  ( 0.000000000000000000, 0.000000000000000000, 1.000000000000000000 ) ) ;
#23789=ORIENTED_EDGE ( 'NONE', *, *, #38589, .F. ) ;
#23791=DIRECTION ( 'NONE',  ( 0.000000000000000000, 0.000000000000000000, 1.000000000000000000 ) ) ;
#23794=EDGE_CURVE ( 'NONE', #36540, #32987, #20502, .T. ) ;
#23801=CIRCLE ( 'NONE', #20567, 1.000000000000000000 ) ;
#23802=AXIS2_PLACEMENT_3D ( 'NONE', #21379, #38568, #35732 ) ;
#23805=DIRECTION ( 'NONE',  ( 0.000000000000000000, 0.000000000000000000, 1.000000000000000000 ) ) ;
#23806=CYLINDRICAL_SURFACE ( 'NONE', #27958, 1.000000000000000000 ) ;
#23810=DIRECTION ( 'NONE',  ( 0.000000000000000000, 0.000000000000000000, 1.000000000000000000 ) ) ;
#23813=CARTESIAN_POINT ( 'NONE',  ( -12.03641663870442713, 15.85735326529964873, 12.00000000000000000 ) ) ;
#23823=ORIENTED_EDGE ( 'NONE', *, *, #28735, .T. ) ;
#23825=EDGE_LOOP ( 'NONE', ( #33727, #39828 ) ) ;
#23833=ORIENTED_EDGE ( 'NONE', *, *, #15926, .T. ) ;
#23839=EDGE_CURVE ( 'NONE', #19392, #3779, #36895, .T. ) ;
#23840=DIRECTION ( 'NONE',  ( 0.000000000000000000, 0.000000000000000000, 1.000000000000000000 ) ) ;
#23846=AXIS2_PLACEMENT_3D ( 'NONE', #13708, #22445, #19816 ) ;
#23856=DIRECTION ( 'NONE',  ( 0.000000000000000000, 0.000000000000000000, 1.000000000000000000 ) ) ;
#23857=CARTESIAN_POINT ( 'NONE',  ( -2.494943660522439099, 10.76222879119470832, 6.000000000000000000 ) ) ;
#23863=EDGE_CURVE ( 'NONE', #13219, #36438, #5015, .T. ) ;
#23867=AXIS2_PLACEMENT_3D ( 'NONE', #26940, #10906, #1762 ) ;
#23876=ORIENTED_EDGE ( 'NONE', *, *, #40180, .F. ) ;
#23888=DIRECTION ( 'NONE',  ( 0.000000000000000000, 0.000000000000000000, 1.000000000000000000 ) ) ;
#23889=DIRECTION ( 'NONE',  ( 0.000000000000000000, 0.000000000000000000, 1.000000000000000000 ) ) ;
#23892=VECTOR ( 'NONE', #14400, 1000.000000000000000 ) ;
#23908=EDGE_CURVE ( 'NONE', #25824, #21424, #11356, .T. ) ;
#23909=DIRECTION ( 'NONE',  ( 0.000000000000000000, 0.000000000000000000, 1.000000000000000000 ) ) ;
#23913=EDGE_CURVE ( 'NONE', #26292, #24105, #17450, .T. ) ;
#23925=ADVANCED_FACE ( 'NONE', ( #8306 ), #8502, .F. ) ;
#23928=AXIS2_PLACEMENT_3D ( 'NONE', #30458, #5654, #27594 ) ;
#23935=DIRECTION ( 'NONE',  ( 1.000000000000000000, 0.000000000000000000, 0.000000000000000000 ) ) ;
#23936=ORIENTED_EDGE ( 'NONE', *, *, #31583, .T. ) ;
#23941=DIRECTION ( 'NONE',  ( 0.000000000000000000, 0.000000000000000000, 1.000000000000000000 ) ) ;
#23945=ORIENTED_EDGE ( 'NONE', *, *, #32250, .T. ) ;
#23948=VECTOR ( 'NONE', #23419, 1000.000000000000000 ) ;
#23954=AXIS2_PLACEMENT_3D ( 'NONE', #6743, #28091, #25048 ) ;
#23959=SURFACE_STYLE_USAGE ( .BOTH. , #20724 ) ;
#23961=CARTESIAN_POINT ( 'NONE',  ( 5.688300058587269170, 16.47782454277055564, 12.00000000000000000 ) ) ;
#23962=DIRECTION ( 'NONE',  ( 1.000000000000000000, 0.000000000000000000, 0.000000000000000000 ) ) ;
#23968=DIRECTION ( 'NONE',  ( 0.000000000000000000, 0.000000000000000000, 1.000000000000000000 ) ) ;
#23978=EDGE_LOOP ( 'NONE', ( #3851, #38671 ) ) ;
#23985=ORIENTED_EDGE ( 'NONE', *, *, #24789, .F. ) ;
#23996=ORIENTED_EDGE ( 'NONE', *, *, #34472, .T. ) ;
#24003=ORIENTED_EDGE ( 'NONE', *, *, #73, .T. ) ;
#24009=CYLINDRICAL_SURFACE ( 'NONE', #34031, 1.000000000000000888 ) ;
#24013=CARTESIAN_POINT ( 'NONE',  ( 2.853166178176219425, 23.42705098312512746, 13.00000000000000178 ) ) ;
#24014=CARTESIAN_POINT ( 'NONE',  ( -18.00000000000000000, 22.50000000000000355, 11.00000000000000178 ) ) ;
#24015=CARTESIAN_POINT ( 'NONE',  ( -4.835137251120299240, 29.44922644035488446, 6.000000000000000000 ) ) ;
#24021=EDGE_CURVE ( 'NONE', #23635, #14685, #12236, .T. ) ;
#24025=ORIENTED_EDGE ( 'NONE', *, *, #9858, .F. ) ;
#24034=UNCERTAINTY_MEASURE_WITH_UNIT (LENGTH_MEASURE( 1.000000000000000082E-05 ), #14816, 'distance_accuracy_value', 'NONE');
#24037=ORIENTED_EDGE ( 'NONE', *, *, #9132, .T. ) ;
#24039=CARTESIAN_POINT ( 'NONE',  ( 13.01837422881150452, 21.26636931122159169, 12.00000000000000000 ) ) ;
#24040=DIRECTION ( 'NONE',  ( 0.000000000000000000, 0.000000000000000000, 1.000000000000000000 ) ) ;
#24041=EDGE_CURVE ( 'NONE', #22404, #13041, #38837, .T. ) ;
#24042=VECTOR ( 'NONE', #18415, 1000.000000000000000 ) ;
#24043=ORIENTED_EDGE ( 'NONE', *, *, #14080, .F. ) ;
#24058=FACE_BOUND ( 'NONE', #30039, .T. ) ;
#24060=DIRECTION ( 'NONE',  ( 0.000000000000000000, 0.000000000000000000, 1.000000000000000000 ) ) ;
#24085=DIRECTION ( 'NONE',  ( 0.000000000000000000, 0.000000000000000000, 1.000000000000000000 ) ) ;
#24090=DIRECTION ( 'NONE',  ( 0.000000000000000000, 0.000000000000000000, 1.000000000000000000 ) ) ;
#24091=DIRECTION ( 'NONE',  ( 0.000000000000000000, 0.000000000000000000, -1.000000000000000000 ) ) ;
#24093=ORIENTED_EDGE ( 'NONE', *, *, #25970, .T. ) ;
#24101=VERTEX_POINT ( 'NONE', #12152 ) ;
#24103=CIRCLE ( 'NONE', #14363, 1.000000000000000000 ) ;
#24104=DIRECTION ( 'NONE',  ( 1.000000000000000000, 0.000000000000000000, 0.000000000000000000 ) ) ;
#24105=VERTEX_POINT ( 'NONE', #6247 ) ;
#24122=DIRECTION ( 'NONE',  ( 1.000000000000000000, 0.000000000000000000, 0.000000000000000000 ) ) ;
#24139=CARTESIAN_POINT ( 'NONE',  ( -5.100643064501314328, 15.70406341247269211, 12.00000000000000000 ) ) ;
#24153=( NAMED_UNIT ( * ) SI_UNIT ( $, .STERADIAN. ) SOLID_ANGLE_UNIT ( ) );
#24154=CARTESIAN_POINT ( 'NONE',  ( -10.41268156625113228, 18.79179606750104981, 12.00000000000000000 ) ) ;
#24160=ORIENTED_EDGE ( 'NONE', *, *, #40144, .T. ) ;
#24168=DIRECTION ( 'NONE',  ( 1.000000000000000000, 0.000000000000000000, 0.000000000000000000 ) ) ;
#24169=CARTESIAN_POINT ( 'NONE',  ( -5.100643064501314328, 15.70406341247269211, 13.00000000000000178 ) ) ;
#24173=AXIS2_PLACEMENT_3D ( 'NONE', #21349, #39627, #3257 ) ;
#24178=DIRECTION ( 'NONE',  ( 0.000000000000000000, 0.000000000000000000, 1.000000000000000000 ) ) ;
#24179=CARTESIAN_POINT ( 'NONE',  ( 10.54146960747273987, 17.40487552589537401, 12.00000000000000000 ) ) ;
#24180=AXIS2_PLACEMENT_3D ( 'NONE', #13429, #18935, #3887 ) ;
#24182=ORIENTED_EDGE ( 'NONE', *, *, #36830, .F. ) ;
#24189=CYLINDRICAL_SURFACE ( 'NONE', #35865, 1.000000000000000000 ) ;
#24198=VECTOR ( 'NONE', #26707, 1000.000000000000000 ) ;
#24199=CARTESIAN_POINT ( 'NONE',  ( 0.000000000000000000, 22.50000000000000355, 13.00000000000000178 ) ) ;
#24225=ORIENTED_EDGE ( 'NONE', *, *, #12866, .F. ) ;
#24238=AXIS2_PLACEMENT_3D ( 'NONE', #4469, #10767, #25593 ) ;
#24242=ADVANCED_FACE ( 'NONE', ( #6834 ), #10099, .F. ) ;
#24243=VERTEX_POINT ( 'NONE', #38329 ) ;
#24250=CARTESIAN_POINT ( 'NONE',  ( 0.000000000000000000, 22.50000000000000355, 11.00000000000000178 ) ) ;
#24252=CIRCLE ( 'NONE', #2194, 1.000000000000000000 ) ;
#24255=AXIS2_PLACEMENT_3D ( 'NONE', #39747, #5430, #21266 ) ;
#24256=FACE_BOUND ( 'NONE', #12039, .T. ) ;
#24260=DIRECTION ( 'NONE',  ( 0.000000000000000000, 0.000000000000000000, 1.000000000000000000 ) ) ;
#24261=CARTESIAN_POINT ( 'NONE',  ( 0.000000000000000000, 22.50000000000000355, 6.000000000000000000 ) ) ;
#24265=EDGE_CURVE ( 'NONE', #32832, #7299, #40132, .T. ) ;
#24268=ORIENTED_EDGE ( 'NONE', *, *, #16613, .T. ) ;
#24269=AXIS2_PLACEMENT_3D ( 'NONE', #14764, #26749, #20670 ) ;
#24274=VERTEX_POINT ( 'NONE', #19436 ) ;
#24282=VECTOR ( 'NONE', #4420, 1000.000000000000000 ) ;
#24286=ORIENTED_EDGE ( 'NONE', *, *, #18791, .F. ) ;
#24294=AXIS2_PLACEMENT_3D ( 'NONE', #12620, #12418, #25008 ) ;
#24301=CIRCLE ( 'NONE', #34077, 1.000000000000000000 ) ;
#24312=CYLINDRICAL_SURFACE ( 'NONE', #21232, 1.000000000000000888 ) ;
#24318=CARTESIAN_POINT ( 'NONE',  ( -10.78894649379783388, 21.72623886970244911, 13.00000000000000178 ) ) ;
#24322=CARTESIAN_POINT ( 'NONE',  ( 16.00000000000000000, 22.50000000000000355, 13.00000000000000178 ) ) ;
#24336=CYLINDRICAL_SURFACE ( 'NONE', #38765, 1.000000000000000000 ) ;
#24349=DIRECTION ( 'NONE',  ( -0.000000000000000000, -0.000000000000000000, -1.000000000000000000 ) ) ;
#24352=AXIS2_PLACEMENT_3D ( 'NONE', #17596, #29965, #36275 ) ;
#24356=DIRECTION ( 'NONE',  ( 0.000000000000000000, 0.000000000000000000, 1.000000000000000000 ) ) ;
#24364=EDGE_LOOP ( 'NONE', ( #6180, #8411, #36036, #23008 ) ) ;
#24366=CARTESIAN_POINT ( 'NONE',  ( -4.476907992048016816, 18.63850621467409496, 6.000000000000000000 ) ) ;
#24377=ORIENTED_EDGE ( 'NONE', *, *, #40127, .F. ) ;
#24381=DIRECTION ( 'NONE',  ( 1.000000000000000000, 0.000000000000000000, 0.000000000000000000 ) ) ;
#24382=AXIS2_PLACEMENT_3D ( 'NONE', #10724, #38754, #32261 ) ;
#24389=ORIENTED_EDGE ( 'NONE', *, *, #25141, .F. ) ;
#24392=ORIENTED_EDGE ( 'NONE', *, *, #4068, .F. ) ;
#24403=FACE_OUTER_BOUND ( 'NONE', #31385, .T. ) ;
#24408=DIRECTION ( 'NONE',  ( 1.000000000000000000, 0.000000000000000000, 0.000000000000000000 ) ) ;
#24414=CARTESIAN_POINT ( 'NONE',  ( 0.01803229776516698107, 30.37627742347970283, 13.00000000000000178 ) ) ;
#24421=CARTESIAN_POINT ( 'NONE',  ( 6.064564986133971658, 13.54338174056915456, 6.000000000000000000 ) ) ;
#24426=FACE_OUTER_BOUND ( 'NONE', #9461, .T. ) ;
#24433=EDGE_LOOP ( 'NONE', ( #28458, #32438 ) ) ;
#24439=ORIENTED_EDGE ( 'NONE', *, *, #370, .F. ) ;
#24441=AXIS2_PLACEMENT_3D ( 'NONE', #27078, #26676, #11242 ) ;
#24443=ADVANCED_FACE ( 'NONE', ( #11115 ), #8055, .F. ) ;
#24448=DIRECTION ( 'NONE',  ( 0.000000000000000000, 0.000000000000000000, 1.000000000000000000 ) ) ;
#24450=CARTESIAN_POINT ( 'NONE',  ( -8.935776944912362296, 22.65328985282726393, 12.00000000000000000 ) ) ;
#24456=LINE ( 'NONE', #33817, #5815 ) ;
#24469=DIRECTION ( 'NONE',  ( 0.000000000000000000, 0.000000000000000000, 1.000000000000000000 ) ) ;
#24470=EDGE_LOOP ( 'NONE', ( #32032, #13926 ) ) ;
#24486=ORIENTED_EDGE ( 'NONE', *, *, #24789, .T. ) ;
#24493=LINE ( 'NONE', #27546, #7613 ) ;
#24495=CIRCLE ( 'NONE', #16083, 1.000000000000000888 ) ;
#24497=LINE ( 'NONE', #11915, #14559 ) ;
#24501=CARTESIAN_POINT ( 'NONE',  ( -10.18324708981896087, 16.78440424842446532, 6.000000000000000000 ) ) ;
#24507=CARTESIAN_POINT ( 'NONE',  ( 7.064564986133971658, 13.54338174056915456, 6.000000000000000000 ) ) ;
#24527=CIRCLE ( 'NONE', #6987, 1.000000000000000888 ) ;
#24528=EDGE_CURVE ( 'NONE', #888, #21822, #24493, .T. ) ;
#24533=CYLINDRICAL_SURFACE ( 'NONE', #9567, 1.000000000000000888 ) ;
#24539=AXIS2_PLACEMENT_3D ( 'NONE', #30494, #605, #22327 ) ;
#24550=DIRECTION ( 'NONE',  ( 0.000000000000000000, 0.000000000000000000, 1.000000000000000000 ) ) ;
#24551=EDGE_LOOP ( 'NONE', ( #18831, #14323, #27733, #7323 ) ) ;
#24552=LINE ( 'NONE', #17872, #23606 ) ;
#24561=CIRCLE ( 'NONE', #13537, 1.000000000000000888 ) ;
#24564=ADVANCED_FACE ( 'NONE', ( #18998 ), #6593, .F. ) ;
#24570=EDGE_CURVE ( 'NONE', #15697, #20746, #6962, .T. ) ;
#24578=ORIENTED_EDGE ( 'NONE', *, *, #31412, .F. ) ;
#24582=FACE_OUTER_BOUND ( 'NONE', #318, .T. ) ;
#24588=LINE ( 'NONE', #25185, #37530 ) ;
#24590=CIRCLE ( 'NONE', #1248, 1.000000000000000000 ) ;
#24594=DIRECTION ( 'NONE',  ( 1.000000000000000000, 0.000000000000000000, 0.000000000000000000 ) ) ;
#24595=ORIENTED_EDGE ( 'NONE', *, *, #3320, .T. ) ;
#24603=DIRECTION ( 'NONE',  ( 0.000000000000000000, 0.000000000000000000, 1.000000000000000000 ) ) ;
#24604=EDGE_LOOP ( 'NONE', ( #31405, #15735 ) ) ;
#24606=CARTESIAN_POINT ( 'NONE',  ( 13.26584437371809777, 27.13525491562438319, 12.00000000000000000 ) ) ;
#24607=DIRECTION ( 'NONE',  ( 0.000000000000000000, 0.000000000000000000, 1.000000000000000000 ) ) ;
#24611=CYLINDRICAL_SURFACE ( 'NONE', #24382, 18.00000000000000000 ) ;
#24621=CARTESIAN_POINT ( 'NONE',  ( -3.494943660522439099, 10.76222879119470832, 12.00000000000000000 ) ) ;
#24627=ORIENTED_EDGE ( 'NONE', *, *, #8680, .F. ) ;
#24631=ORIENTED_EDGE ( 'NONE', *, *, #22434, .T. ) ;
#24635=ORIENTED_EDGE ( 'NONE', *, *, #22803, .F. ) ;
#24639=VECTOR ( 'NONE', #26096, 1000.000000000000000 ) ;
#24642=EDGE_CURVE ( 'NONE', #20723, #14246, #9573, .T. ) ;
#24643=ORIENTED_EDGE ( 'NONE', *, *, #11864, .F. ) ;
#24647=CARTESIAN_POINT ( 'NONE',  ( 7.577540944421576441, 33.15743037285414374, 12.00000000000000000 ) ) ;
#24648=DIRECTION ( 'NONE',  ( 0.000000000000000000, 0.000000000000000000, 1.000000000000000000 ) ) ;
#24649=EDGE_CURVE ( 'NONE', #29357, #25284, #17388, .T. ) ;
#24651=EDGE_CURVE ( 'NONE', #20746, #15697, #1127, .T. ) ;
#24652=FACE_BOUND ( 'NONE', #23068, .T. ) ;
#24656=CARTESIAN_POINT ( 'NONE',  ( 5.458865582155095986, 18.48521636184714012, 6.000000000000000000 ) ) ;
#24659=DIRECTION ( 'NONE',  ( 1.000000000000000000, 0.000000000000000000, 0.000000000000000000 ) ) ;
#24666=CARTESIAN_POINT ( 'NONE',  ( -16.99999999999999645, 22.50000000000000355, 11.00000000000000178 ) ) ;
#24668=ORIENTED_EDGE ( 'NONE', *, *, #25017, .F. ) ;
#24683=DIRECTION ( 'NONE',  ( 1.000000000000000000, 0.000000000000000000, 0.000000000000000000 ) ) ;
#24692=VERTEX_POINT ( 'NONE', #28734 ) ;
#24696=ORIENTED_EDGE ( 'NONE', *, *, #9154, .T. ) ;
#24715=EDGE_CURVE ( 'NONE', #880, #6684, #14115, .T. ) ;
#24757=VERTEX_POINT ( 'NONE', #1516 ) ;
#24762=DIRECTION ( 'NONE',  ( 1.000000000000000000, 0.000000000000000000, 0.000000000000000000 ) ) ;
#24780=CARTESIAN_POINT ( 'NONE',  ( -8.559512017365658920, 19.71884705062586107, 6.000000000000000000 ) ) ;
#24789=EDGE_CURVE ( 'NONE', #21042, #4736, #14765, .T. ) ;
#24791=EDGE_CURVE ( 'NONE', #29047, #36540, #28382, .T. ) ;
#24798=CARTESIAN_POINT ( 'NONE',  ( 7.935770203493858865, 22.34671014717335780, 6.000000000000000000 ) ) ;
#24804=CARTESIAN_POINT ( 'NONE',  ( -7.312041872459064784, 25.58773265502866678, 12.00000000000000000 ) ) ;
#24811=FACE_OUTER_BOUND ( 'NONE', #16347, .T. ) ;
#24820=VERTEX_POINT ( 'NONE', #28536 ) ;
#24823=FACE_BOUND ( 'NONE', #15988, .T. ) ;
#24833=CARTESIAN_POINT ( 'NONE',  ( -2.494943660522439099, 10.76222879119470832, 12.00000000000000000 ) ) ;
#24845=FACE_OUTER_BOUND ( 'NONE', #15677, .T. ) ;
#24850=CYLINDRICAL_SURFACE ( 'NONE', #10618, 1.000000000000000888 ) ;
#24854=CARTESIAN_POINT ( 'NONE',  ( 10.77090408390491127, 15.39748370681878775, 12.00000000000000000 ) ) ;
#24857=DIRECTION ( 'NONE',  ( 0.000000000000000000, 0.000000000000000000, 1.000000000000000000 ) ) ;
#24859=AXIS2_PLACEMENT_3D ( 'NONE', #7514, #20526, #32524 ) ;
#24860=EDGE_LOOP ( 'NONE', ( #31624, #34972, #9716, #6888 ) ) ;
#24867=ORIENTED_EDGE ( 'NONE', *, *, #22185, .F. ) ;
#24868=DIRECTION ( 'NONE',  ( 0.000000000000000000, 0.000000000000000000, 1.000000000000000000 ) ) ;
#24871=CARTESIAN_POINT ( 'NONE',  ( -3.211402178667006169, 32.38366924255629442, 6.000000000000000000 ) ) ;
#24873=CARTESIAN_POINT ( 'NONE',  ( 5.348106467989403257, 35.16482219193073178, 13.00000000000000178 ) ) ;
#24881=CARTESIAN_POINT ( 'NONE',  ( 8.312035131040566682, 19.41226734497195849, 12.00000000000000000 ) ) ;
#24883=ADVANCED_FACE ( 'NONE', ( #4354 ), #29145, .F. ) ;
#24889=AXIS2_PLACEMENT_3D ( 'NONE', #39091, #17782, #2128 ) ;
#24891=ORIENTED_EDGE ( 'NONE', *, *, #37458, .T. ) ;
#24894=AXIS2_PLACEMENT_3D ( 'NONE', #579, #15618, #10318 ) ;
#24899=AXIS2_PLACEMENT_3D ( 'NONE', #5063, #1621, #32708 ) ;
#24908=LINE ( 'NONE', #9476, #39191 ) ;
#24911=ORIENTED_EDGE ( 'NONE', *, *, #16815, .F. ) ;
#24913=DIRECTION ( 'NONE',  ( 1.000000000000000000, 0.000000000000000000, 0.000000000000000000 ) ) ;
#24916=EDGE_CURVE ( 'NONE', #23691, #16497, #26442, .T. ) ;
#24937=ORIENTED_EDGE ( 'NONE', *, *, #1727, .T. ) ;
#24945=CARTESIAN_POINT ( 'NONE',  ( 0.01803229776516698107, 30.37627742347970283, 6.000000000000000000 ) ) ;
#24946=VERTEX_POINT ( 'NONE', #33418 ) ;
#24948=DIRECTION ( 'NONE',  ( 0.000000000000000000, 0.000000000000000000, 1.000000000000000000 ) ) ;
#24950=CIRCLE ( 'NONE', #30151, 1.000000000000000888 ) ;
#24952=VERTEX_POINT ( 'NONE', #14713 ) ;
#24956=CIRCLE ( 'NONE', #26258, 1.000000000000000000 ) ;
#24975=DIRECTION ( 'NONE',  ( 0.000000000000000000, 0.000000000000000000, 1.000000000000000000 ) ) ;
#24978=DIRECTION ( 'NONE',  ( 0.000000000000000000, 0.000000000000000000, 1.000000000000000000 ) ) ;
#24982=EDGE_LOOP ( 'NONE', ( #10791, #24392 ) ) ;
#24994=VERTEX_POINT ( 'NONE', #17171 ) ;
#24998=ADVANCED_FACE ( 'NONE', ( #11069 ), #26498, .F. ) ;
#25001=ORIENTED_EDGE ( 'NONE', *, *, #31603, .F. ) ;
#25005=CARTESIAN_POINT ( 'NONE',  ( -2.587667106213709101, 35.31811204475769728, 6.000000000000000000 ) ) ;
#25008=DIRECTION ( 'NONE',  ( 1.000000000000000000, 0.000000000000000000, 0.000000000000000000 ) ) ;
#25017=EDGE_CURVE ( 'NONE', #11791, #15766, #18052, .T. ) ;
#25018=CARTESIAN_POINT ( 'NONE',  ( -4.458872323573595864, 26.51478363815348160, 6.000000000000000000 ) ) ;
#25023=FACE_BOUND ( 'NONE', #15660, .T. ) ;
#25048=DIRECTION ( 'NONE',  ( 1.000000000000000000, 0.000000000000000000, 0.000000000000000000 ) ) ;
#25051=FACE_BOUND ( 'NONE', #1358, .T. ) ;
#25057=CARTESIAN_POINT ( 'NONE',  ( -11.89031881743725805, 33.20608791387860492, 13.00000000000000178 ) ) ;
#25058=EDGE_CURVE ( 'NONE', #33648, #5046, #27112, .T. ) ;
#25060=ORIENTED_EDGE ( 'NONE', *, *, #34499, .F. ) ;
#25067=FACE_OUTER_BOUND ( 'NONE', #5257, .T. ) ;
#25072=DIRECTION ( 'NONE',  ( 1.000000000000000000, 0.000000000000000000, 0.000000000000000000 ) ) ;
#25082=CARTESIAN_POINT ( 'NONE',  ( 1.871201846650637046, 31.30332840660451765, 13.00000000000000178 ) ) ;
#25095=AXIS2_PLACEMENT_3D ( 'NONE', #12783, #29583, #19843 ) ;
#25101=DIRECTION ( 'NONE',  ( 1.000000000000000000, 0.000000000000000000, 0.000000000000000000 ) ) ;
#25102=DIRECTION ( 'NONE',  ( 0.000000000000000000, 0.000000000000000000, 1.000000000000000000 ) ) ;
#25108=AXIS2_PLACEMENT_3D ( 'NONE', #3963, #28948, #925 ) ;
#25118=ORIENTED_EDGE ( 'NONE', *, *, #4151, .F. ) ;
#25128=ORIENTED_EDGE ( 'NONE', *, *, #35344, .F. ) ;
#25133=ORIENTED_EDGE ( 'NONE', *, *, #26546, .F. ) ;
#25141=EDGE_CURVE ( 'NONE', #22096, #10782, #30370, .T. ) ;
#25155=DIRECTION ( 'NONE',  ( 1.000000000000000000, 0.000000000000000000, 0.000000000000000000 ) ) ;
#25157=AXIS2_PLACEMENT_3D ( 'NONE', #39820, #30888, #10 ) ;
#25177=ADVANCED_FACE ( 'NONE', ( #24845 ), #21596, .F. ) ;
#25183=ORIENTED_EDGE ( 'NONE', *, *, #36473, .F. ) ;
#25185=CARTESIAN_POINT ( 'NONE',  ( 1.229431105722923023, 20.49260818092372460, 6.000000000000000000 ) ) ;
#25196=CARTESIAN_POINT ( 'NONE',  ( -3.211402178667006169, 32.38366924255629442, 6.000000000000000000 ) ) ;
#25200=VECTOR ( 'NONE', #17258, 1000.000000000000000 ) ;
#25206=FACE_OUTER_BOUND ( 'NONE', #5554, .T. ) ;
#25213=VERTEX_POINT ( 'NONE', #2914 ) ;
#25225=FACE_BOUND ( 'NONE', #10954, .T. ) ;
#25228=CARTESIAN_POINT ( 'NONE',  ( -5.082607396026893376, 23.58034083595207875, 6.000000000000000000 ) ) ;
#25233=ORIENTED_EDGE ( 'NONE', *, *, #17076, .F. ) ;
#25235=VERTEX_POINT ( 'NONE', #6156 ) ;
#25244=CIRCLE ( 'NONE', #33708, 1.000000000000000000 ) ;
#25251=FACE_BOUND ( 'NONE', #29174, .T. ) ;
#25252=DIRECTION ( 'NONE',  ( 0.000000000000000000, 0.000000000000000000, 1.000000000000000000 ) ) ;
#25262=ORIENTED_EDGE ( 'NONE', *, *, #34900, .F. ) ;
#25265=ORIENTED_EDGE ( 'NONE', *, *, #22401, .F. ) ;
#25280=DIRECTION ( 'NONE',  ( 0.000000000000000000, 0.000000000000000000, 1.000000000000000000 ) ) ;
#25282=DIRECTION ( 'NONE',  ( 1.000000000000000000, 0.000000000000000000, 0.000000000000000000 ) ) ;
#25284=VERTEX_POINT ( 'NONE', #2225 ) ;
#25288=ORIENTED_EDGE ( 'NONE', *, *, #6049, .F. ) ;
#25290=ADVANCED_FACE ( 'NONE', ( #26391 ), #4856, .F. ) ;
#25296=AXIS2_PLACEMENT_3D ( 'NONE', #16472, #21606, #278 ) ;
#25297=DIRECTION ( 'NONE',  ( 1.000000000000000000, 0.000000000000000000, 0.000000000000000000 ) ) ;
#25302=FACE_OUTER_BOUND ( 'NONE', #22749, .T. ) ;
#25303=AXIS2_PLACEMENT_3D ( 'NONE', #31394, #25483, #25690 ) ;
#25313=CARTESIAN_POINT ( 'NONE',  ( 6.688300058587269170, 16.47782454277055564, 12.00000000000000000 ) ) ;
#25323=ORIENTED_EDGE ( 'NONE', *, *, #24528, .F. ) ;
#25337=VERTEX_POINT ( 'NONE', #33311 ) ;
#25338=VERTEX_POINT ( 'NONE', #17272 ) ;
#25341=AXIS2_PLACEMENT_3D ( 'NONE', #30561, #30358, #18362 ) ;
#25354=CARTESIAN_POINT ( 'NONE',  ( -7.064571727552472424, 31.45661825943146894, 12.00000000000000000 ) ) ;
#25357=VECTOR ( 'NONE', #28800, 1000.000000000000000 ) ;
#25365=EDGE_CURVE ( 'NONE', #12173, #33298, #33625, .T. ) ;
#25375=AXIS2_PLACEMENT_3D ( 'NONE', #1066, #20366, #26039 ) ;
#25382=ORIENTED_EDGE ( 'NONE', *, *, #14385, .F. ) ;
#25384=ORIENTED_EDGE ( 'NONE', *, *, #23839, .T. ) ;
#25386=DIRECTION ( 'NONE',  ( 0.000000000000000000, 0.000000000000000000, 1.000000000000000000 ) ) ;
#25390=ORIENTED_EDGE ( 'NONE', *, *, #35971, .T. ) ;
#25394=CYLINDRICAL_SURFACE ( 'NONE', #22758, 1.000000000000000000 ) ;
#25400=ORIENTED_EDGE ( 'NONE', *, *, #6887, .T. ) ;
#25404=CARTESIAN_POINT ( 'NONE',  ( -4.724378136954611840, 12.76962061027129458, 13.00000000000000178 ) ) ;
#25409=CIRCLE ( 'NONE', #7902, 1.000000000000000000 ) ;
#25410=CARTESIAN_POINT ( 'NONE',  ( 3.118671991557230516, 37.17221401100731981, 13.00000000000000178 ) ) ;
#25416=FACE_BOUND ( 'NONE', #27688, .T. ) ;
#25423=DIRECTION ( 'NONE',  ( 0.000000000000000000, 0.000000000000000000, 1.000000000000000000 ) ) ;
#25424=VERTEX_POINT ( 'NONE', #14408 ) ;
#25431=CARTESIAN_POINT ( 'NONE',  ( 7.559505275947156377, 25.28115294937476065, 12.00000000000000000 ) ) ;
#25434=ADVANCED_FACE ( 'NONE', ( #2421 ), #11162, .F. ) ;
#25438=FACE_BOUND ( 'NONE', #4362, .T. ) ;
#25446=AXIS2_PLACEMENT_3D ( 'NONE', #35408, #38654, #29910 ) ;
#25452=DIRECTION ( 'NONE',  ( 1.000000000000000000, 0.000000000000000000, 0.000000000000000000 ) ) ;
#25460=ORIENTED_EDGE ( 'NONE', *, *, #10388, .T. ) ;
#25468=AXIS2_PLACEMENT_3D ( 'NONE', #38631, #1871, #20948 ) ;
#25480=CYLINDRICAL_SURFACE ( 'NONE', #31393, 1.000000000000000888 ) ;
#25482=CIRCLE ( 'NONE', #17078, 1.000000000000000000 ) ;
#25483=DIRECTION ( 'NONE',  ( 0.000000000000000000, 0.000000000000000000, 1.000000000000000000 ) ) ;
#25493=CARTESIAN_POINT ( 'NONE',  ( -3.587667106213709101, 35.31811204475769728, 12.00000000000000000 ) ) ;
#25497=ORIENTED_EDGE ( 'NONE', *, *, #31412, .T. ) ;
#25500=DIRECTION ( 'NONE',  ( 0.000000000000000000, 0.000000000000000000, 1.000000000000000000 ) ) ;
#25511=CIRCLE ( 'NONE', #14505, 1.000000000000000000 ) ;
#25523=AXIS2_PLACEMENT_3D ( 'NONE', #4626, #17027, #10932 ) ;
#25533=ORIENTED_EDGE ( 'NONE', *, *, #35457, .T. ) ;
#25546=CARTESIAN_POINT ( 'NONE',  ( -11.03641663870442713, 15.85735326529964873, 13.00000000000000178 ) ) ;
#25561=EDGE_CURVE ( 'NONE', #26852, #5502, #4434, .T. ) ;
#25562=CIRCLE ( 'NONE', #38534, 1.000000000000000888 ) ;
#25576=DIRECTION ( 'NONE',  ( 0.000000000000000000, 0.000000000000000000, 1.000000000000000000 ) ) ;
#25580=CARTESIAN_POINT ( 'NONE',  ( -3.835137251120299684, 29.44922644035488446, 6.000000000000000000 ) ) ;
#25581=ORIENTED_EDGE ( 'NONE', *, *, #39973, .F. ) ;
#25584=ORIENTED_EDGE ( 'NONE', *, *, #38037, .F. ) ;
#25593=DIRECTION ( 'NONE',  ( 1.000000000000000000, 0.000000000000000000, 0.000000000000000000 ) ) ;
#25596=EDGE_CURVE ( 'NONE', #6257, #12049, #12158, .T. ) ;
#25603=CARTESIAN_POINT ( 'NONE',  ( -4.348113209407908464, 9.835177808069893501, 13.00000000000000178 ) ) ;
#25610=ORIENTED_EDGE ( 'NONE', *, *, #26514, .T. ) ;
#25615=FACE_BOUND ( 'NONE', #11659, .T. ) ;
#25619=VERTEX_POINT ( 'NONE', #31245 ) ;
#25626=CARTESIAN_POINT ( 'NONE',  ( 2.211395437248501850, 12.61633075744433796, 12.00000000000000000 ) ) ;
#25627=ORIENTED_EDGE ( 'NONE', *, *, #34721, .F. ) ;
#25637=EDGE_CURVE ( 'NONE', #19392, #35589, #2501, .T. ) ;
#25639=AXIS2_PLACEMENT_3D ( 'NONE', #27122, #11089, #8635 ) ;
#25641=CIRCLE ( 'NONE', #20483, 1.000000000000000000 ) ;
#25642=FACE_BOUND ( 'NONE', #33434, .T. ) ;
#25646=ADVANCED_FACE ( 'NONE', ( #27991 ), #28439, .T. ) ;
#25648=EDGE_CURVE ( 'NONE', #8022, #14474, #9514, .T. ) ;
#25651=EDGE_LOOP ( 'NONE', ( #29187, #29394 ) ) ;
#25654=DIRECTION ( 'NONE',  ( 0.000000000000000000, 0.000000000000000000, 1.000000000000000000 ) ) ;
#25656=ORIENTED_EDGE ( 'NONE', *, *, #33226, .F. ) ;
#25664=ORIENTED_EDGE ( 'NONE', *, *, #20964, .F. ) ;
#25667=CYLINDRICAL_SURFACE ( 'NONE', #23549, 1.000000000000000000 ) ;
#25671=DIRECTION ( 'NONE',  ( 1.000000000000000000, 0.000000000000000000, 0.000000000000000000 ) ) ;
#25674=EDGE_CURVE ( 'NONE', #17668, #33348, #37527, .T. ) ;
#25680=CIRCLE ( 'NONE', #28932, 16.00000000000000000 ) ;
#25683=ORIENTED_EDGE ( 'NONE', *, *, #12296, .F. ) ;
#25686=VERTEX_POINT ( 'NONE', #35651 ) ;
#25689=EDGE_CURVE ( 'NONE', #3455, #13041, #34495, .T. ) ;
#25690=DIRECTION ( 'NONE',  ( 1.000000000000000000, 0.000000000000000000, 0.000000000000000000 ) ) ;
#25691=CYLINDRICAL_SURFACE ( 'NONE', #9321, 1.000000000000000000 ) ;
#25692=DIRECTION ( 'NONE',  ( 1.000000000000000000, 0.000000000000000000, 0.000000000000000000 ) ) ;
#25694=DIRECTION ( 'NONE',  ( 0.000000000000000000, 0.000000000000000000, 1.000000000000000000 ) ) ;
#25695=DIRECTION ( 'NONE',  ( 0.000000000000000000, 0.000000000000000000, 1.000000000000000000 ) ) ;
#25702=ORIENTED_EDGE ( 'NONE', *, *, #15480, .T. ) ;
#25705=LINE ( 'NONE', #13309, #14223 ) ;
#25706=DIRECTION ( 'NONE',  ( 1.000000000000000000, 0.000000000000000000, 0.000000000000000000 ) ) ;
#25707=CIRCLE ( 'NONE', #433, 1.000000000000000888 ) ;
#25711=ORIENTED_EDGE ( 'NONE', *, *, #17836, .F. ) ;
#25728=EDGE_CURVE ( 'NONE', #14129, #24820, #16558, .T. ) ;
#25730=ORIENTED_EDGE ( 'NONE', *, *, #5546, .T. ) ;
#25732=CARTESIAN_POINT ( 'NONE',  ( -0.3582326297815359162, 33.31072022568110924, 6.000000000000000000 ) ) ;
#25737=ORIENTED_EDGE ( 'NONE', *, *, #9833, .F. ) ;
#25742=EDGE_LOOP ( 'NONE', ( #25118, #23381, #14192, #11310 ) ) ;
#25745=FACE_OUTER_BOUND ( 'NONE', #40064, .T. ) ;
#25748=CARTESIAN_POINT ( 'NONE',  ( -10.16521142134453548, 24.66068167190384841, 6.000000000000000000 ) ) ;
#25752=VERTEX_POINT ( 'NONE', #1518 ) ;
#25755=CARTESIAN_POINT ( 'NONE',  ( 0.3762615568374529929, 19.56555719779890978, 6.000000000000000000 ) ) ;
#25758=CARTESIAN_POINT ( 'NONE',  ( 10.54146960747273987, 17.40487552589537401, 6.000000000000000000 ) ) ;
#25761=CARTESIAN_POINT ( 'NONE',  ( 2.211395437248501850, 12.61633075744433796, 6.000000000000000000 ) ) ;
#25773=EDGE_CURVE ( 'NONE', #33038, #22329, #35588, .T. ) ;
#25774=ORIENTED_EDGE ( 'NONE', *, *, #13131, .T. ) ;
#25784=DIRECTION ( 'NONE',  ( 1.000000000000000000, 0.000000000000000000, 0.000000000000000000 ) ) ;
#25790=DIRECTION ( 'NONE',  ( 1.000000000000000000, 0.000000000000000000, 0.000000000000000000 ) ) ;
#25795=AXIS2_PLACEMENT_3D ( 'NONE', #16999, #7840, #13938 ) ;
#25798=EDGE_CURVE ( 'NONE', #26803, #8150, #36892, .T. ) ;
#25801=AXIS2_PLACEMENT_3D ( 'NONE', #27741, #18409, #28333 ) ;
#25802=CARTESIAN_POINT ( 'NONE',  ( -5.440836655099179353, 34.39106106163288246, 13.00000000000000178 ) ) ;
#25818=VERTEX_POINT ( 'NONE', #38693 ) ;
#25821=FACE_BOUND ( 'NONE', #22871, .T. ) ;
#25824=VERTEX_POINT ( 'NONE', #20009 ) ;
#25827=DIRECTION ( 'NONE',  ( 0.000000000000000000, 0.000000000000000000, 1.000000000000000000 ) ) ;
#25828=AXIS2_PLACEMENT_3D ( 'NONE', #14305, #13906, #38692 ) ;
#25829=EDGE_LOOP ( 'NONE', ( #19633, #15447 ) ) ;
#25831=CARTESIAN_POINT ( 'NONE',  ( 5.064564986133971658, 13.54338174056915456, 13.00000000000000178 ) ) ;
#25844=AXIS2_PLACEMENT_3D ( 'NONE', #27038, #20551, #32944 ) ;
#25845=FACE_BOUND ( 'NONE', #11655, .T. ) ;
#25852=ORIENTED_EDGE ( 'NONE', *, *, #15094, .T. ) ;
#25860=ORIENTED_EDGE ( 'NONE', *, *, #11618, .T. ) ;
#25872=EDGE_CURVE ( 'NONE', #21859, #16360, #10292, .T. ) ;
#25885=CARTESIAN_POINT ( 'NONE',  ( 0.000000000000000000, 22.50000000000000355, 13.00000000000000178 ) ) ;
#25894=EDGE_CURVE ( 'NONE', #20361, #3606, #38831, .T. ) ;
#25895=DIRECTION ( 'NONE',  ( 1.000000000000000000, 0.000000000000000000, 0.000000000000000000 ) ) ;
#25900=DIRECTION ( 'NONE',  ( 0.000000000000000000, 0.000000000000000000, 1.000000000000000000 ) ) ;
#25902=ORIENTED_EDGE ( 'NONE', *, *, #23794, .T. ) ;
#25908=ORIENTED_EDGE ( 'NONE', *, *, #28959, .T. ) ;
#25912=ORIENTED_EDGE ( 'NONE', *, *, #7716, .T. ) ;
#25935=VERTEX_POINT ( 'NONE', #14508 ) ;
#25937=AXIS2_PLACEMENT_3D ( 'NONE', #12162, #3220, #36752 ) ;
#25938=CARTESIAN_POINT ( 'NONE',  ( 12.03640989728592459, 29.14264673470096767, 13.00000000000000178 ) ) ;
#25947=DIRECTION ( 'NONE',  ( 0.000000000000000000, 0.000000000000000000, 1.000000000000000000 ) ) ;
#25950=FACE_OUTER_BOUND ( 'NONE', #5187, .T. ) ;
#25954=DIRECTION ( 'NONE',  ( 0.000000000000000000, 0.000000000000000000, 1.000000000000000000 ) ) ;
#25965=CARTESIAN_POINT ( 'NONE',  ( -7.953812613386786801, 14.77701242934787906, 13.00000000000000178 ) ) ;
#25970=EDGE_CURVE ( 'NONE', #39380, #11229, #24561, .T. ) ;
#25972=ORIENTED_EDGE ( 'NONE', *, *, #32494, .T. ) ;
#25978=ORIENTED_EDGE ( 'NONE', *, *, #22480, .T. ) ;
#25985=ORIENTED_EDGE ( 'NONE', *, *, #5517, .F. ) ;
#26003=DIRECTION ( 'NONE',  ( 0.000000000000000000, 0.000000000000000000, 1.000000000000000000 ) ) ;
#26009=AXIS2_PLACEMENT_3D ( 'NONE', #1675, #4920, #35803 ) ;
#26012=CIRCLE ( 'NONE', #27962, 1.000000000000000000 ) ;
#26015=ORIENTED_EDGE ( 'NONE', *, *, #22456, .T. ) ;
#26019=FACE_BOUND ( 'NONE', #14413, .T. ) ;
#26024=ADVANCED_FACE ( 'NONE', ( #2915 ), #15306, .F. ) ;
#26036=VERTEX_POINT ( 'NONE', #11669 ) ;
#26039=DIRECTION ( 'NONE',  ( 1.000000000000000000, 0.000000000000000000, 0.000000000000000000 ) ) ;
#26043=AXIS2_PLACEMENT_3D ( 'NONE', #29645, #32709, #29248 ) ;
#26045=EDGE_CURVE ( 'NONE', #10818, #6396, #1220, .T. ) ;
#26051=CARTESIAN_POINT ( 'NONE',  ( 9.806975420853749625, 31.15003855377755571, 12.00000000000000000 ) ) ;
#26061=FACE_OUTER_BOUND ( 'NONE', #2220, .T. ) ;
#26067=ORIENTED_EDGE ( 'NONE', *, *, #13339, .T. ) ;
#26070=CARTESIAN_POINT ( 'NONE',  ( -12.01838097023000529, 23.73363068877903359, 6.000000000000000000 ) ) ;
#26072=EDGE_LOOP ( 'NONE', ( #40022, #25262, #17670, #28791 ) ) ;
#26075=DIRECTION ( 'NONE',  ( 0.000000000000000000, 0.000000000000000000, 1.000000000000000000 ) ) ;
#26082=AXIS2_PLACEMENT_3D ( 'NONE', #27542, #17821, #27737 ) ;
#26090=DIRECTION ( 'NONE',  ( 1.000000000000000000, 0.000000000000000000, 0.000000000000000000 ) ) ;
#26096=DIRECTION ( 'NONE',  ( 0.000000000000000000, 0.000000000000000000, 1.000000000000000000 ) ) ;
#26108=EDGE_CURVE ( 'NONE', #29599, #21075, #24590, .T. ) ;
#26116=DIRECTION ( 'NONE',  ( 1.000000000000000000, 0.000000000000000000, 0.000000000000000000 ) ) ;
#26119=AXIS2_PLACEMENT_3D ( 'NONE', #33982, #5940, #39865 ) ;
#26132=EDGE_LOOP ( 'NONE', ( #23434, #63, #7495, #38839 ) ) ;
#26133=DIRECTION ( 'NONE',  ( 1.000000000000000000, 0.000000000000000000, 0.000000000000000000 ) ) ;
#26140=ORIENTED_EDGE ( 'NONE', *, *, #38418, .T. ) ;
#26142=CYLINDRICAL_SURFACE ( 'NONE', #33141, 1.000000000000000000 ) ;
#26143=AXIS2_PLACEMENT_3D ( 'NONE', #23266, #20827, #20425 ) ;
#26164=DIRECTION ( 'NONE',  ( 0.000000000000000000, 0.000000000000000000, 1.000000000000000000 ) ) ;
#26168=CIRCLE ( 'NONE', #24894, 1.000000000000000000 ) ;
#26175=ORIENTED_EDGE ( 'NONE', *, *, #1074, .T. ) ;
#26193=CARTESIAN_POINT ( 'NONE',  ( 13.01837422881150452, 21.26636931122159169, 13.00000000000000178 ) ) ;
#26208=CARTESIAN_POINT ( 'NONE',  ( -8.806982162272252168, 13.84996144622306247, 12.00000000000000000 ) ) ;
#26209=CARTESIAN_POINT ( 'NONE',  ( 4.100636323082810009, 29.29593658752792962, 13.00000000000000178 ) ) ;
#26215=CIRCLE ( 'NONE', #21695, 1.000000000000000000 ) ;
#26219=ORIENTED_EDGE ( 'NONE', *, *, #21554, .F. ) ;
#26224=AXIS2_PLACEMENT_3D ( 'NONE', #528, #28553, #19207 ) ;
#26226=DIRECTION ( 'NONE',  ( 1.000000000000000000, 0.000000000000000000, 0.000000000000000000 ) ) ;
#26236=ADVANCED_FACE ( 'NONE', ( #31745 ), #13045, .F. ) ;
#26238=VECTOR ( 'NONE', #8323, 1000.000000000000000 ) ;
#26249=ADVANCED_FACE ( 'NONE', ( #37834 ), #34001, .F. ) ;
#26258=AXIS2_PLACEMENT_3D ( 'NONE', #22648, #9868, #13306 ) ;
#26265=EDGE_CURVE ( 'NONE', #9140, #31499, #10968, .T. ) ;
#26271=VERTEX_POINT ( 'NONE', #26448 ) ;
#26284=FACE_OUTER_BOUND ( 'NONE', #17553, .T. ) ;
#26286=EDGE_CURVE ( 'NONE', #31324, #7177, #34999, .T. ) ;
#26292=VERTEX_POINT ( 'NONE', #14055 ) ;
#26301=ADVANCED_FACE ( 'NONE', ( #16714 ), #10208, .F. ) ;
#26307=DIRECTION ( 'NONE',  ( 0.000000000000000000, 0.000000000000000000, 1.000000000000000000 ) ) ;
#26313=SURFACE_SIDE_STYLE ('',( #13919 ) ) ;
#26314=ORIENTED_EDGE ( 'NONE', *, *, #12220, .T. ) ;
#26328=VECTOR ( 'NONE', #19924, 1000.000000000000000 ) ;
#26334=CARTESIAN_POINT ( 'NONE',  ( -15.21690460405485545, 17.55572914666943873, 12.00000000000000000 ) ) ;
#26337=EDGE_LOOP ( 'NONE', ( #32253, #13352 ) ) ;
#26350=CIRCLE ( 'NONE', #12746, 1.000000000000000000 ) ;
#26351=DIRECTION ( 'NONE',  ( 0.000000000000000000, 0.000000000000000000, 1.000000000000000000 ) ) ;
#26352=ORIENTED_EDGE ( 'NONE', *, *, #1425, .F. ) ;
#26355=VECTOR ( 'NONE', #27764, 1000.000000000000000 ) ;
#26364=CARTESIAN_POINT ( 'NONE',  ( 6.064564986133971658, 13.54338174056915456, 13.00000000000000178 ) ) ;
#26365=CARTESIAN_POINT ( 'NONE',  ( -9.183247089818959097, 16.78440424842446532, 13.00000000000000178 ) ) ;
#26367=DIRECTION ( 'NONE',  ( 0.000000000000000000, 0.000000000000000000, 1.000000000000000000 ) ) ;
#26370=CARTESIAN_POINT ( 'NONE',  ( -3.476907992048017260, 18.63850621467409496, 12.00000000000000000 ) ) ;
#26375=CARTESIAN_POINT ( 'NONE',  ( 11.78893975237933134, 23.27376113029817617, 12.00000000000000000 ) ) ;
#26376=ORIENTED_EDGE ( 'NONE', *, *, #30259, .F. ) ;
#26386=ORIENTED_EDGE ( 'NONE', *, *, #32408, .T. ) ;
#26388=ADVANCED_FACE ( 'NONE', ( #19547 ), #19753, .F. ) ;
#26391=FACE_OUTER_BOUND ( 'NONE', #10773, .T. ) ;
#26392=ORIENTED_EDGE ( 'NONE', *, *, #36830, .T. ) ;
#26400=DIRECTION ( 'NONE',  ( 0.000000000000000000, 0.000000000000000000, 1.000000000000000000 ) ) ;
#26401=CARTESIAN_POINT ( 'NONE',  ( -0.9819677022348329842, 30.37627742347970283, 13.00000000000000178 ) ) ;
#26413=AXIS2_PLACEMENT_3D ( 'NONE', #29834, #14602, #14399 ) ;
#26421=EDGE_LOOP ( 'NONE', ( #2066, #33698, #26015, #28754 ) ) ;
#26422=EDGE_LOOP ( 'NONE', ( #22135, #20049 ) ) ;
#26425=LINE ( 'NONE', #10591, #22391 ) ;
#26427=CARTESIAN_POINT ( 'NONE',  ( 3.476901250629512941, 26.36149378532653031, 6.000000000000000000 ) ) ;
#26428=ORIENTED_EDGE ( 'NONE', *, *, #39800, .F. ) ;
#26437=ORIENTED_EDGE ( 'NONE', *, *, #27423, .F. ) ;
#26442=CIRCLE ( 'NONE', #36831, 1.000000000000000888 ) ;
#26447=CIRCLE ( 'NONE', #29699, 1.000000000000000000 ) ;
#26448=CARTESIAN_POINT ( 'NONE',  ( -12.64211604268330724, 20.79918788657763429, 13.00000000000000178 ) ) ;
#26450=LINE ( 'NONE', #32966, #30587 ) ;
#26459=CARTESIAN_POINT ( 'NONE',  ( 4.724371395536106633, 32.23037938972932892, 13.00000000000000178 ) ) ;
#26485=ORIENTED_EDGE ( 'NONE', *, *, #10012, .T. ) ;
#26493=ADVANCED_FACE ( 'NONE', ( #1673 ), #35800, .F. ) ;
#26498=CYLINDRICAL_SURFACE ( 'NONE', #15453, 1.000000000000000000 ) ;
#26500=CIRCLE ( 'NONE', #27776, 1.000000000000000888 ) ;
#26502=DIRECTION ( 'NONE',  ( 0.000000000000000000, 0.000000000000000000, 1.000000000000000000 ) ) ;
#26503=AXIS2_PLACEMENT_3D ( 'NONE', #4355, #1116, #4968 ) ;
#26508=ORIENTED_EDGE ( 'NONE', *, *, #20767, .F. ) ;
#26513=EDGE_CURVE ( 'NONE', #9757, #17958, #34339, .T. ) ;
#26514=EDGE_CURVE ( 'NONE', #5201, #22834, #36921, .T. ) ;
#26516=DIRECTION ( 'NONE',  ( 1.000000000000000000, 0.000000000000000000, 0.000000000000000000 ) ) ;
#26517=EDGE_CURVE ( 'NONE', #15234, #1646, #8381, .T. ) ;
#26520=ORIENTED_EDGE ( 'NONE', *, *, #25773, .F. ) ;
#26526=ORIENTED_EDGE ( 'NONE', *, *, #20676, .F. ) ;
#26528=ORIENTED_EDGE ( 'NONE', *, *, #4352, .F. ) ;
#26533=VECTOR ( 'NONE', #858, 1000.000000000000000 ) ;
#26546=EDGE_CURVE ( 'NONE', #9387, #33664, #16802, .T. ) ;
#26556=CIRCLE ( 'NONE', #2462, 1.000000000000000000 ) ;
#26557=AXIS2_PLACEMENT_3D ( 'NONE', #9280, #6420, #24913 ) ;
#26571=DIRECTION ( 'NONE',  ( 1.000000000000000000, 0.000000000000000000, 0.000000000000000000 ) ) ;
#26582=ORIENTED_EDGE ( 'NONE', *, *, #39048, .F. ) ;
#26584=VERTEX_POINT ( 'NONE', #18121 ) ;
#26587=ORIENTED_EDGE ( 'NONE', *, *, #15267, .F. ) ;
#26599=DIRECTION ( 'NONE',  ( 0.000000000000000000, 0.000000000000000000, 1.000000000000000000 ) ) ;
#26603=CARTESIAN_POINT ( 'NONE',  ( -1.494943660522439099, 10.76222879119470832, 6.000000000000000000 ) ) ;
#26604=DIRECTION ( 'NONE',  ( 0.000000000000000000, 0.000000000000000000, 1.000000000000000000 ) ) ;
#26614=CIRCLE ( 'NONE', #4573, 1.000000000000000000 ) ;
#26629=DIRECTION ( 'NONE',  ( 0.000000000000000000, 0.000000000000000000, 1.000000000000000000 ) ) ;
#26657=TOROIDAL_SURFACE ( 'NONE', #31845, 16.00000000000000000, 2.000000000000000000 ) ;
#26659=CARTESIAN_POINT ( 'NONE',  ( 12.03640989728592459, 29.14264673470096767, 12.00000000000000000 ) ) ;
#26660=DIRECTION ( 'NONE',  ( 0.000000000000000000, 0.000000000000000000, 1.000000000000000000 ) ) ;
#26661=CYLINDRICAL_SURFACE ( 'NONE', #5791, 1.000000000000000888 ) ;
#26670=EDGE_CURVE ( 'NONE', #13041, #22404, #32368, .T. ) ;
#26671=ORIENTED_EDGE ( 'NONE', *, *, #18716, .T. ) ;
#26674=ORIENTED_EDGE ( 'NONE', *, *, #32462, .T. ) ;
#26676=DIRECTION ( 'NONE',  ( 0.000000000000000000, 0.000000000000000000, 1.000000000000000000 ) ) ;
#26688=ORIENTED_EDGE ( 'NONE', *, *, #16815, .T. ) ;
#26691=AXIS2_PLACEMENT_3D ( 'NONE', #23362, #35958, #38394 ) ;
#26694=EDGE_CURVE ( 'NONE', #5105, #30551, #20747, .T. ) ;
#26705=VERTEX_POINT ( 'NONE', #17921 ) ;
#26707=DIRECTION ( 'NONE',  ( 0.000000000000000000, 0.000000000000000000, 1.000000000000000000 ) ) ;
#26708=FACE_OUTER_BOUND ( 'NONE', #13754, .T. ) ;
#26716=ORIENTED_EDGE ( 'NONE', *, *, #30897, .F. ) ;
#26727=EDGE_CURVE ( 'NONE', #2950, #37992, #35648, .T. ) ;
#26733=ORIENTED_EDGE ( 'NONE', *, *, #20256, .T. ) ;
#26735=DIRECTION ( 'NONE',  ( 0.000000000000000000, 0.000000000000000000, 1.000000000000000000 ) ) ;
#26736=AXIS2_PLACEMENT_3D ( 'NONE', #9059, #12302, #39532 ) ;
#26745=EDGE_CURVE ( 'NONE', #7299, #880, #607, .T. ) ;
#26747=AXIS2_PLACEMENT_3D ( 'NONE', #5326, #10827, #38857 ) ;
#26748=ORIENTED_EDGE ( 'NONE', *, *, #5914, .T. ) ;
#26749=DIRECTION ( 'NONE',  ( 0.000000000000000000, 0.000000000000000000, 1.000000000000000000 ) ) ;
#26753=DIRECTION ( 'NONE',  ( 0.000000000000000000, 0.000000000000000000, 1.000000000000000000 ) ) ;
#26755=CIRCLE ( 'NONE', #31939, 1.000000000000000888 ) ;
#26758=EDGE_CURVE ( 'NONE', #7299, #19863, #14232, .T. ) ;
#26766=ADVANCED_FACE ( 'NONE', ( #28444 ), #37195, .F. ) ;
#26783=VERTEX_POINT ( 'NONE', #3065 ) ;
#26785=CIRCLE ( 'NONE', #13172, 1.000000000000000000 ) ;
#26786=CARTESIAN_POINT ( 'NONE',  ( -1.494943660522439099, 10.76222879119470832, 13.00000000000000178 ) ) ;
#26791=VERTEX_POINT ( 'NONE', #9369 ) ;
#26793=ADVANCED_FACE ( 'NONE', ( #31102 ), #31498, .F. ) ;
#26803=VERTEX_POINT ( 'NONE', #12210 ) ;
#26825=EDGE_LOOP ( 'NONE', ( #1051, #38714, #21906, #10542 ) ) ;
#26828=CIRCLE ( 'NONE', #9318, 1.000000000000000888 ) ;
#26839=ORIENTED_EDGE ( 'NONE', *, *, #25648, .T. ) ;
#26841=AXIS2_PLACEMENT_3D ( 'NONE', #13104, #27954, #19012 ) ;
#26843=EDGE_LOOP ( 'NONE', ( #27668, #22146, #23038, #29553 ) ) ;
#26852=VERTEX_POINT ( 'NONE', #27646 ) ;
#26857=CIRCLE ( 'NONE', #8711, 1.000000000000000000 ) ;
#26865=AXIS2_PLACEMENT_3D ( 'NONE', #24013, #20377, #39050 ) ;
#26872=ORIENTED_EDGE ( 'NONE', *, *, #21575, .F. ) ;
#26880=EDGE_LOOP ( 'NONE', ( #8591, #21897, #14252, #33840 ) ) ;
#26888=ORIENTED_EDGE ( 'NONE', *, *, #9621, .T. ) ;
#26893=EDGE_CURVE ( 'NONE', #32909, #14918, #23316, .T. ) ;
#26897=CIRCLE ( 'NONE', #9379, 16.00000000000000000 ) ;
#26900=EDGE_CURVE ( 'NONE', #24946, #33412, #16056, .T. ) ;
#26903=CIRCLE ( 'NONE', #16523, 1.000000000000000888 ) ;
#26904=FACE_OUTER_BOUND ( 'NONE', #27982, .T. ) ;
#26909=FACE_OUTER_BOUND ( 'NONE', #29367, .T. ) ;
#26931=VECTOR ( 'NONE', #1047, 1000.000000000000000 ) ;
#26936=VERTEX_POINT ( 'NONE', #13604 ) ;
#26938=DIRECTION ( 'NONE',  ( 0.000000000000000000, 0.000000000000000000, 1.000000000000000000 ) ) ;
#26940=CARTESIAN_POINT ( 'NONE',  ( 2.587660364795204782, 9.681887955242936883, 12.00000000000000000 ) ) ;
#26942=ORIENTED_EDGE ( 'NONE', *, *, #4519, .T. ) ;
#26950=DIRECTION ( 'NONE',  ( 1.000000000000000000, 0.000000000000000000, 0.000000000000000000 ) ) ;
#26962=DIRECTION ( 'NONE',  ( 0.000000000000000000, 0.000000000000000000, 1.000000000000000000 ) ) ;
#26964=DIRECTION ( 'NONE',  ( 1.000000000000000000, 0.000000000000000000, 0.000000000000000000 ) ) ;
#26968=VERTEX_POINT ( 'NONE', #4668 ) ;
#26970=AXIS2_PLACEMENT_3D ( 'NONE', #19732, #35170, #29278 ) ;
#26971=DIRECTION ( 'NONE',  ( 0.000000000000000000, 0.000000000000000000, 1.000000000000000000 ) ) ;
#26972=CARTESIAN_POINT ( 'NONE',  ( -6.312041872459064784, 25.58773265502866678, 13.00000000000000178 ) ) ;
#26983=CARTESIAN_POINT ( 'NONE',  ( -2.494943660522439099, 10.76222879119470832, 12.00000000000000000 ) ) ;
#26984=EDGE_LOOP ( 'NONE', ( #39067, #30375 ) ) ;
#26998=AXIS2_PLACEMENT_3D ( 'NONE', #344, #37516, #26116 ) ;
#27000=CIRCLE ( 'NONE', #6882, 1.000000000000000000 ) ;
#27002=DIRECTION ( 'NONE',  ( 0.000000000000000000, 0.000000000000000000, 1.000000000000000000 ) ) ;
#27005=LINE ( 'NONE', #39387, #20141 ) ;
#27007=CARTESIAN_POINT ( 'NONE',  ( -1.000003370709253492, 22.50000000000031264, 6.000000000000000000 ) ) ;
#27017=CYLINDRICAL_SURFACE ( 'NONE', #20511, 1.000000000000000000 ) ;
#27029=ORIENTED_EDGE ( 'NONE', *, *, #169, .T. ) ;
#27030=ORIENTED_EDGE ( 'NONE', *, *, #7889, .T. ) ;
#27035=EDGE_LOOP ( 'NONE', ( #31687, #33397 ) ) ;
#27038=CARTESIAN_POINT ( 'NONE',  ( -1.605702774688126722, 27.44183462127829642, 12.00000000000000000 ) ) ;
#27040=ORIENTED_EDGE ( 'NONE', *, *, #20230, .T. ) ;
#27048=EDGE_LOOP ( 'NONE', ( #28924, #2983, #24268, #26140 ) ) ;
#27054=CIRCLE ( 'NONE', #9538, 1.000000000000000000 ) ;
#27055=CIRCLE ( 'NONE', #7583, 1.000000000000000000 ) ;
#27067=ORIENTED_EDGE ( 'NONE', *, *, #10882, .T. ) ;
#27074=ORIENTED_EDGE ( 'NONE', *, *, #1313, .F. ) ;
#27078=CARTESIAN_POINT ( 'NONE',  ( -5.706342468480190000, 20.64589803375067945, 12.00000000000000000 ) ) ;
#27080=DIRECTION ( 'NONE',  ( 0.000000000000000000, 0.000000000000000000, 1.000000000000000000 ) ) ;
#27081=VECTOR ( 'NONE', #22626, 1000.000000000000000 ) ;
#27100=CARTESIAN_POINT ( 'NONE',  ( 2.229431105722923245, 20.49260818092372460, 6.000000000000000000 ) ) ;
#27103=AXIS2_PLACEMENT_3D ( 'NONE', #20756, #8752, #39025 ) ;
#27104=CIRCLE ( 'NONE', #32303, 1.000000000000000000 ) ;
#27105=LINE ( 'NONE', #38897, #30081 ) ;
#27106=CARTESIAN_POINT ( 'NONE',  ( -0.2474735156158440752, 16.63111439559750693, 6.000000000000000000 ) ) ;
#27109=CARTESIAN_POINT ( 'NONE',  ( 14.26584437371809777, 27.13525491562438319, 12.00000000000000000 ) ) ;
#27112=CIRCLE ( 'NONE', #25828, 1.000000000000000000 ) ;
#27113=LINE ( 'NONE', #11477, #28090 ) ;
#27114=DIRECTION ( 'NONE',  ( 1.000000000000000000, 0.000000000000000000, 0.000000000000000000 ) ) ;
#27122=CARTESIAN_POINT ( 'NONE',  ( -14.26585111513660031, 17.86474508437623143, 13.00000000000000178 ) ) ;
#27140=ADVANCED_FACE ( 'NONE', ( #10362 ), #22741, .F. ) ;
#27151=CIRCLE ( 'NONE', #32995, 1.000000000000000000 ) ;
#27156=CARTESIAN_POINT ( 'NONE',  ( 5.953805871968278929, 30.22298757065274444, 12.00000000000000000 ) ) ;
#27162=DIRECTION ( 'NONE',  ( 1.000000000000000000, 0.000000000000000000, 0.000000000000000000 ) ) ;
#27165=AXIS2_PLACEMENT_3D ( 'NONE', #9804, #13039, #34585 ) ;
#27168=AXIS2_PLACEMENT_3D ( 'NONE', #18545, #8805, #33597 ) ;
#27177=ORIENTED_EDGE ( 'NONE', *, *, #4151, .T. ) ;
#27185=CARTESIAN_POINT ( 'NONE',  ( -15.26585111513660209, 17.86474508437623143, 6.000000000000000000 ) ) ;
#27199=ORIENTED_EDGE ( 'NONE', *, *, #14758, .T. ) ;
#27214=CARTESIAN_POINT ( 'NONE',  ( -9.294006203984645609, 33.46401007850805343, 12.00000000000000000 ) ) ;
#27215=DIRECTION ( 'NONE',  ( 1.000000000000000000, 0.000000000000000000, 0.000000000000000000 ) ) ;
#27222=AXIS2_PLACEMENT_3D ( 'NONE', #23054, #7611, #1527 ) ;
#27230=CARTESIAN_POINT ( 'NONE',  ( -6.688306800005769048, 28.52217545723006609, 6.000000000000000000 ) ) ;
#27239=CARTESIAN_POINT ( 'NONE',  ( 7.935770203493858865, 22.34671014717335780, 12.00000000000000000 ) ) ;
#27243=ORIENTED_EDGE ( 'NONE', *, *, #4886, .T. ) ;
#27246=EDGE_CURVE ( 'NONE', #30103, #32913, #11764, .T. ) ;
#27247=DIRECTION ( 'NONE',  ( 1.000000000000000000, 0.000000000000000000, 0.000000000000000000 ) ) ;
#27248=EDGE_CURVE ( 'NONE', #17958, #14918, #14210, .T. ) ;
#27264=ORIENTED_EDGE ( 'NONE', *, *, #23441, .F. ) ;
#27265=EDGE_CURVE ( 'NONE', #34434, #1614, #32404, .T. ) ;
#27275=VERTEX_POINT ( 'NONE', #23754 ) ;
#27281=CARTESIAN_POINT ( 'NONE',  ( 11.39463915635820612, 18.33192650902018883, 6.000000000000000000 ) ) ;
#27282=ORIENTED_EDGE ( 'NONE', *, *, #28529, .T. ) ;
#27287=EDGE_LOOP ( 'NONE', ( #25060, #507, #24037, #35011 ) ) ;
#27289=CYLINDRICAL_SURFACE ( 'NONE', #29074, 1.000000000000000888 ) ;
#27290=CYLINDRICAL_SURFACE ( 'NONE', #36158, 1.000000000000000000 ) ;
#27304=CARTESIAN_POINT ( 'NONE',  ( 15.26584437371809955, 27.13525491562438319, 13.00000000000000178 ) ) ;
#27305=FACE_BOUND ( 'NONE', #1213, .T. ) ;
#27307=ORIENTED_EDGE ( 'NONE', *, *, #20330, .T. ) ;
#27309=DIRECTION ( 'NONE',  ( 0.000000000000000000, 0.000000000000000000, 1.000000000000000000 ) ) ;
#27328=AXIS2_PLACEMENT_3D ( 'NONE', #1472, #7351, #17125 ) ;
#27333=ORIENTED_EDGE ( 'NONE', *, *, #17421, .F. ) ;
#27336=CARTESIAN_POINT ( 'NONE',  ( -8.806982162272252168, 13.84996144622306247, 6.000000000000000000 ) ) ;
#27347=ADVANCED_FACE ( 'NONE', ( #30257 ), #5068, .F. ) ;
#27358=CARTESIAN_POINT ( 'NONE',  ( -3.211402178667006169, 32.38366924255629442, 13.00000000000000178 ) ) ;
#27371=VERTEX_POINT ( 'NONE', #39591 ) ;
#27372=DIRECTION ( 'NONE',  ( 0.000000000000000000, 0.000000000000000000, 1.000000000000000000 ) ) ;
#27378=DIRECTION ( 'NONE',  ( 1.000000000000000000, 0.000000000000000000, 0.000000000000000000 ) ) ;
#27413=CARTESIAN_POINT ( 'NONE',  ( -1.358232629781535916, 33.31072022568110924, 6.000000000000000000 ) ) ;
#27421=AXIS2_PLACEMENT_3D ( 'NONE', #14248, #36389, #7945 ) ;
#27423=EDGE_CURVE ( 'NONE', #30133, #1553, #3874, .T. ) ;
#27428=CARTESIAN_POINT ( 'NONE',  ( -0.6417741116369681809, 11.68927977431952137, 6.000000000000000000 ) ) ;
#27433=DIRECTION ( 'NONE',  ( 1.000000000000000000, 0.000000000000000000, 0.000000000000000000 ) ) ;
#27438=ORIENTED_EDGE ( 'NONE', *, *, #18791, .T. ) ;
#27440=ORIENTED_EDGE ( 'NONE', *, *, #20930, .T. ) ;
#27447=DIRECTION ( 'NONE',  ( 0.000000000000000000, 0.000000000000000000, 1.000000000000000000 ) ) ;
#27451=CYLINDRICAL_SURFACE ( 'NONE', #14337, 1.000000000000000888 ) ;
#27454=DIRECTION ( 'NONE',  ( 1.000000000000000000, 0.000000000000000000, 0.000000000000000000 ) ) ;
#27460=EDGE_LOOP ( 'NONE', ( #38328, #3724, #25384, #14429, #13897, #7827, #10828 ) ) ;
#27468=VERTEX_POINT ( 'NONE', #21896 ) ;
#27474=EDGE_CURVE ( 'NONE', #35589, #25619, #9117, .T. ) ;
#27475=CIRCLE ( 'NONE', #13872, 1.000000000000000000 ) ;
#27480=EDGE_LOOP ( 'NONE', ( #8369, #29170, #29512, #30169 ) ) ;
#27483=( GEOMETRIC_REPRESENTATION_CONTEXT ( 3 ) GLOBAL_UNCERTAINTY_ASSIGNED_CONTEXT ( ( #8593 ) ) GLOBAL_UNIT_ASSIGNED_CONTEXT ( ( #11767, #35956, #24153 ) ) REPRESENTATION_CONTEXT ( 'NONE', 'WORKASPACE' ) );
#27494=ADVANCED_FACE ( 'NONE', ( #376 ), #28194, .F. ) ;
#27500=AXIS2_PLACEMENT_3D ( 'NONE', #26659, #36409, #5519 ) ;
#27502=FACE_BOUND ( 'NONE', #34892, .T. ) ;
#27503=CARTESIAN_POINT ( 'NONE',  ( -11.41268156625113406, 18.79179606750104981, 6.000000000000000000 ) ) ;
#27506=CARTESIAN_POINT ( 'NONE',  ( -11.03641663870442713, 15.85735326529964873, 12.00000000000000000 ) ) ;
#27507=CARTESIAN_POINT ( 'NONE',  ( -13.01838097023000707, 23.73363068877903359, 6.000000000000000000 ) ) ;
#27509=CARTESIAN_POINT ( 'NONE',  ( -11.03641663870442713, 15.85735326529964873, 6.000000000000000000 ) ) ;
#27518=ORIENTED_EDGE ( 'NONE', *, *, #29360, .T. ) ;
#27523=CARTESIAN_POINT ( 'NONE',  ( -4.348113209407908464, 9.835177808069893501, 12.00000000000000000 ) ) ;
#27527=EDGE_CURVE ( 'NONE', #15652, #23393, #11964, .T. ) ;
#27536=DIRECTION ( 'NONE',  ( 0.000000000000000000, 0.000000000000000000, 1.000000000000000000 ) ) ;
#27540=AXIS2_PLACEMENT_3D ( 'NONE', #23813, #11226, #8380 ) ;
#27542=CARTESIAN_POINT ( 'NONE',  ( 11.41267482483262619, 26.20820393249957192, 12.00000000000000000 ) ) ;
#27546=CARTESIAN_POINT ( 'NONE',  ( 4.211395437248501850, 12.61633075744433796, 6.000000000000000000 ) ) ;
#27550=DIRECTION ( 'NONE',  ( 1.000000000000000000, 0.000000000000000000, 0.000000000000000000 ) ) ;
#27582=ADVANCED_FACE ( 'NONE', ( #34692 ), #569, .F. ) ;
#27594=DIRECTION ( 'NONE',  ( 1.000000000000000000, 0.000000000000000000, 0.000000000000000000 ) ) ;
#27599=AXIS2_PLACEMENT_3D ( 'NONE', #36309, #12118, #36902 ) ;
#27631=EDGE_CURVE ( 'NONE', #37992, #21619, #23101, .T. ) ;
#27646=CARTESIAN_POINT ( 'NONE',  ( 5.458865582155095986, 18.48521636184714012, 13.00000000000000178 ) ) ;
#27650=EDGE_CURVE ( 'NONE', #19611, #22765, #29836, .T. ) ;
#27651=FACE_OUTER_BOUND ( 'NONE', #38382, .T. ) ;
#27656=FACE_OUTER_BOUND ( 'NONE', #13227, .T. ) ;
#27660=DIRECTION ( 'NONE',  ( 0.000000000000000000, 0.000000000000000000, 1.000000000000000000 ) ) ;
#27666=CARTESIAN_POINT ( 'NONE',  ( 11.89031559783845005, 11.79390851039467236, 13.00000000000000178 ) ) ;
#27667=ORIENTED_EDGE ( 'NONE', *, *, #4197, .T. ) ;
#27668=ORIENTED_EDGE ( 'NONE', *, *, #32366, .F. ) ;
#27671=EDGE_CURVE ( 'NONE', #17473, #2121, #33743, .T. ) ;
#27681=ORIENTED_EDGE ( 'NONE', *, *, #24649, .F. ) ;
#27685=AXIS2_PLACEMENT_3D ( 'NONE', #38870, #17549, #1493 ) ;
#27688=EDGE_LOOP ( 'NONE', ( #19933, #5724 ) ) ;
#27693=CARTESIAN_POINT ( 'NONE',  ( -2.871208588069141143, 13.69667159339610762, 13.00000000000000178 ) ) ;
#27699=CARTESIAN_POINT ( 'NONE',  ( -6.330077540933487512, 17.71145523154927659, 13.00000000000000178 ) ) ;
#27704=CIRCLE ( 'NONE', #16054, 1.000000000000000888 ) ;
#27714=AXIS2_PLACEMENT_3D ( 'NONE', #33505, #11556, #38980 ) ;
#27726=ORIENTED_EDGE ( 'NONE', *, *, #13717, .T. ) ;
#27730=ADVANCED_FACE ( 'NONE', ( #17017 ), #28995, .F. ) ;
#27733=ORIENTED_EDGE ( 'NONE', *, *, #29289, .T. ) ;
#27737=DIRECTION ( 'NONE',  ( 1.000000000000000000, 0.000000000000000000, 0.000000000000000000 ) ) ;
#27741=CARTESIAN_POINT ( 'NONE',  ( -6.064571727552472424, 31.45661825943146894, 12.00000000000000000 ) ) ;
#27742=AXIS2_PLACEMENT_3D ( 'NONE', #31285, #18106, #9555 ) ;
#27747=AXIS2_PLACEMENT_3D ( 'NONE', #8864, #39930, #9463 ) ;
#27751=DIRECTION ( 'NONE',  ( 0.000000000000000000, 0.000000000000000000, 1.000000000000000000 ) ) ;
#27755=DIRECTION ( 'NONE',  ( 1.000000000000000000, 0.000000000000000000, 0.000000000000000000 ) ) ;
#27756=DIRECTION ( 'NONE',  ( 0.000000000000000000, 0.000000000000000000, 1.000000000000000000 ) ) ;
#27760=DIRECTION ( 'NONE',  ( 0.000000000000000000, 0.000000000000000000, 1.000000000000000000 ) ) ;
#27764=DIRECTION ( 'NONE',  ( 0.000000000000000000, 0.000000000000000000, 1.000000000000000000 ) ) ;
#27776=AXIS2_PLACEMENT_3D ( 'NONE', #6975, #26075, #37867 ) ;
#27780=EDGE_CURVE ( 'NONE', #33109, #4829, #3246, .T. ) ;
#27782=DIRECTION ( 'NONE',  ( 0.000000000000000000, 0.000000000000000000, 1.000000000000000000 ) ) ;
#27784=AXIS2_PLACEMENT_3D ( 'NONE', #33807, #21995, #21402 ) ;
#27796=VERTEX_POINT ( 'NONE', #32862 ) ;
#27799=EDGE_CURVE ( 'NONE', #37025, #14056, #2378, .T. ) ;
#27807=VECTOR ( 'NONE', #24550, 1000.000000000000000 ) ;
#27813=VERTEX_POINT ( 'NONE', #14767 ) ;
#27819=CARTESIAN_POINT ( 'NONE',  ( 7.935770203493858865, 22.34671014717335780, 6.000000000000000000 ) ) ;
#27829=AXIS2_PLACEMENT_3D ( 'NONE', #27819, #30873, #21915 ) ;
#27836=AXIS2_PLACEMENT_3D ( 'NONE', #17325, #29700, #1881 ) ;
#27843=VERTEX_POINT ( 'NONE', #27156 ) ;
#27850=CARTESIAN_POINT ( 'NONE',  ( 0.000000000000000000, 22.50000000000000355, 13.00000000000000178 ) ) ;
#27853=CARTESIAN_POINT ( 'NONE',  ( 5.082600654608392610, 21.41965916404854298, 6.000000000000000000 ) ) ;
#27854=DIRECTION ( 'NONE',  ( 0.000000000000000000, 0.000000000000000000, 1.000000000000000000 ) ) ;
#27862=DIRECTION ( 'NONE',  ( 1.000000000000000000, 0.000000000000000000, 0.000000000000000000 ) ) ;
#27863=DIRECTION ( 'NONE',  ( 1.000000000000000000, 0.000000000000000000, 0.000000000000000000 ) ) ;
#27864=ORIENTED_EDGE ( 'NONE', *, *, #20945, .F. ) ;
#27873=FACE_BOUND ( 'NONE', #13232, .T. ) ;
#27878=ORIENTED_EDGE ( 'NONE', *, *, #2893, .F. ) ;
#27880=DIRECTION ( 'NONE',  ( 1.000000000000000000, 0.000000000000000000, 0.000000000000000000 ) ) ;
#27885=ORIENTED_EDGE ( 'NONE', *, *, #5019, .T. ) ;
#27896=LINE ( 'NONE', #9016, #34437 ) ;
#27897=EDGE_CURVE ( 'NONE', #32004, #29377, #16914, .T. ) ;
#27898=FACE_BOUND ( 'NONE', #8044, .T. ) ;
#27902=ADVANCED_FACE ( 'NONE', ( #23311 ), #35705, .F. ) ;
#27903=DIRECTION ( 'NONE',  ( 0.000000000000000000, 0.000000000000000000, 1.000000000000000000 ) ) ;
#27918=DIRECTION ( 'NONE',  ( 0.000000000000000000, 0.000000000000000000, 1.000000000000000000 ) ) ;
#27920=DIRECTION ( 'NONE',  ( 0.000000000000000000, 0.000000000000000000, 1.000000000000000000 ) ) ;
#27932=DIRECTION ( 'NONE',  ( 1.000000000000000000, 0.000000000000000000, 0.000000000000000000 ) ) ;
#27945=EDGE_CURVE ( 'NONE', #36183, #13580, #11716, .T. ) ;
#27947=DIRECTION ( 'NONE',  ( 1.000000000000000000, 0.000000000000000000, 0.000000000000000000 ) ) ;
#27952=DIRECTION ( 'NONE',  ( 0.000000000000000000, 0.000000000000000000, 1.000000000000000000 ) ) ;
#27954=DIRECTION ( 'NONE',  ( 0.000000000000000000, 0.000000000000000000, 1.000000000000000000 ) ) ;
#27958=AXIS2_PLACEMENT_3D ( 'NONE', #30708, #5716, #8973 ) ;
#27962=AXIS2_PLACEMENT_3D ( 'NONE', #14051, #38842, #23403 ) ;
#27968=CARTESIAN_POINT ( 'NONE',  ( -10.80698216227225394, 13.84996144622306247, 6.000000000000000000 ) ) ;
#27976=CIRCLE ( 'NONE', #20861, 1.000000000000000000 ) ;
#27982=EDGE_LOOP ( 'NONE', ( #30655, #36716, #34747, #8415 ) ) ;
#27983=DIRECTION ( 'NONE',  ( 0.000000000000000000, 0.000000000000000000, 1.000000000000000000 ) ) ;
#27991=FACE_OUTER_BOUND ( 'NONE', #20387, .T. ) ;
#28001=CARTESIAN_POINT ( 'NONE',  ( -0.6237384431625470071, 19.56555719779890978, 13.00000000000000178 ) ) ;
#28002=CIRCLE ( 'NONE', #10492, 1.000000000000000888 ) ;
#28016=CIRCLE ( 'NONE', #31900, 1.000000000000000000 ) ;
#28029=ORIENTED_EDGE ( 'NONE', *, *, #7716, .F. ) ;
#28034=ORIENTED_EDGE ( 'NONE', *, *, #20915, .F. ) ;
#28036=DIRECTION ( 'NONE',  ( 1.000000000000000000, 0.000000000000000000, 0.000000000000000000 ) ) ;
#28039=VERTEX_POINT ( 'NONE', #31003 ) ;
#28043=EDGE_CURVE ( 'NONE', #7967, #40046, #26614, .T. ) ;
#28048=DIRECTION ( 'NONE',  ( 0.000000000000000000, 0.000000000000000000, 1.000000000000000000 ) ) ;
#28069=FACE_BOUND ( 'NONE', #1808, .T. ) ;
#28070=EDGE_LOOP ( 'NONE', ( #36533, #28565, #34144, #497 ) ) ;
#28074=VERTEX_POINT ( 'NONE', #8868 ) ;
#28079=ORIENTED_EDGE ( 'NONE', *, *, #2669, .F. ) ;
#28083=FACE_OUTER_BOUND ( 'NONE', #28070, .T. ) ;
#28086=CIRCLE ( 'NONE', #2144, 16.00000000000000000 ) ;
#28088=FACE_OUTER_BOUND ( 'NONE', #28996, .T. ) ;
#28090=VECTOR ( 'NONE', #17389, 1000.000000000000000 ) ;
#28091=DIRECTION ( 'NONE',  ( 0.000000000000000000, 0.000000000000000000, 1.000000000000000000 ) ) ;
#28093=CIRCLE ( 'NONE', #15779, 1.000000000000000000 ) ;
#28094=FACE_BOUND ( 'NONE', #581, .T. ) ;
#28113=VERTEX_POINT ( 'NONE', #36899 ) ;
#28126=EDGE_CURVE ( 'NONE', #15410, #13580, #21452, .T. ) ;
#28129=DIRECTION ( 'NONE',  ( 0.000000000000000000, 0.000000000000000000, 1.000000000000000000 ) ) ;
#28133=CIRCLE ( 'NONE', #3480, 1.000000000000000000 ) ;
#28145=CARTESIAN_POINT ( 'NONE',  ( -8.312041872459065672, 25.58773265502866678, 6.000000000000000000 ) ) ;
#28149=DIRECTION ( 'NONE',  ( 0.000000000000000000, 0.000000000000000000, 1.000000000000000000 ) ) ;
#28152=FACE_OUTER_BOUND ( 'NONE', #9707, .T. ) ;
#28153=CARTESIAN_POINT ( 'NONE',  ( 8.541469607472738090, 17.40487552589537401, 6.000000000000000000 ) ) ;
#28176=CARTESIAN_POINT ( 'NONE',  ( 0.000000000000000000, 22.50000000000000355, 13.00000000000000178 ) ) ;
#28189=CARTESIAN_POINT ( 'NONE',  ( 1.358225888363031819, 11.68927977431952137, 6.000000000000000000 ) ) ;
#28191=CARTESIAN_POINT ( 'NONE',  ( -3.835137251120299684, 29.44922644035488446, 12.00000000000000000 ) ) ;
#28193=CIRCLE ( 'NONE', #18463, 1.000000000000000000 ) ;
#28194=CYLINDRICAL_SURFACE ( 'NONE', #25937, 1.000000000000000000 ) ;
#28200=CIRCLE ( 'NONE', #6786, 1.000000000000000000 ) ;
#28201=CARTESIAN_POINT ( 'NONE',  ( 13.03640989728592459, 29.14264673470096767, 6.000000000000000000 ) ) ;
#28206=ORIENTED_EDGE ( 'NONE', *, *, #18839, .F. ) ;
#28220=ORIENTED_EDGE ( 'NONE', *, *, #24642, .T. ) ;
#28223=ADVANCED_FACE ( 'NONE', ( #16767 ), #19197, .F. ) ;
#28225=AXIS2_PLACEMENT_3D ( 'NONE', #15578, #36919, #24122 ) ;
#28233=ORIENTED_EDGE ( 'NONE', *, *, #13717, .F. ) ;
#28245=LINE ( 'NONE', #421, #22154 ) ;
#28247=DIRECTION ( 'NONE',  ( 0.000000000000000000, 0.000000000000000000, 1.000000000000000000 ) ) ;
#28249=LINE ( 'NONE', #19300, #20962 ) ;
#28252=EDGE_CURVE ( 'NONE', #25424, #10554, #16241, .T. ) ;
#28254=DIRECTION ( 'NONE',  ( 0.000000000000000000, 0.000000000000000000, 1.000000000000000000 ) ) ;
#28259=VECTOR ( 'NONE', #8789, 1000.000000000000000 ) ;
#28266=DIRECTION ( 'NONE',  ( 1.000000000000000000, 0.000000000000000000, 0.000000000000000000 ) ) ;
#28279=EDGE_CURVE ( 'NONE', #2419, #37407, #23373, .T. ) ;
#28284=ORIENTED_EDGE ( 'NONE', *, *, #17363, .F. ) ;
#28296=CARTESIAN_POINT ( 'NONE',  ( -13.39464589777671044, 26.66807349098043289, 13.00000000000000178 ) ) ;
#28297=FACE_BOUND ( 'NONE', #29259, .T. ) ;
#28301=DIRECTION ( 'NONE',  ( 1.000000000000000000, 0.000000000000000000, 0.000000000000000000 ) ) ;
#28303=ORIENTED_EDGE ( 'NONE', *, *, #39922, .T. ) ;
#28309=DIRECTION ( 'NONE',  ( 1.000000000000000000, 0.000000000000000000, 0.000000000000000000 ) ) ;
#28312=CARTESIAN_POINT ( 'NONE',  ( 5.440829913680675034, 10.60893893836775348, 13.00000000000000178 ) ) ;
#28324=DIRECTION ( 'NONE',  ( 0.000000000000000000, 0.000000000000000000, 1.000000000000000000 ) ) ;
#28325=DIRECTION ( 'NONE',  ( -0.000000000000000000, -0.000000000000000000, -1.000000000000000000 ) ) ;
#28331=ORIENTED_EDGE ( 'NONE', *, *, #28959, .F. ) ;
#28333=DIRECTION ( 'NONE',  ( 1.000000000000000000, 0.000000000000000000, 0.000000000000000000 ) ) ;
#28343=CARTESIAN_POINT ( 'NONE',  ( 0.000000000000000000, 22.50000000000000355, 11.00000000000000178 ) ) ;
#28346=DIRECTION ( 'NONE',  ( 0.000000000000000000, 0.000000000000000000, 1.000000000000000000 ) ) ;
#28349=AXIS2_PLACEMENT_3D ( 'NONE', #39942, #33672, #3568 ) ;
#28368=ORIENTED_EDGE ( 'NONE', *, *, #13515, .F. ) ;
#28377=ORIENTED_EDGE ( 'NONE', *, *, #14135, .T. ) ;
#28379=ADVANCED_FACE ( 'NONE', ( #17174 ), #29346, .F. ) ;
#28382=CIRCLE ( 'NONE', #21886, 1.000000000000000000 ) ;
#28387=AXIS2_PLACEMENT_3D ( 'NONE', #29382, #7843, #1557 ) ;
#28395=CYLINDRICAL_SURFACE ( 'NONE', #32777, 1.000000000000000000 ) ;
#28397=VECTOR ( 'NONE', #38158, 1000.000000000000000 ) ;
#28404=AXIS2_PLACEMENT_3D ( 'NONE', #33650, #26735, #14947 ) ;
#28409=DIRECTION ( 'NONE',  ( 1.000000000000000000, 0.000000000000000000, 0.000000000000000000 ) ) ;
#28427=ADVANCED_FACE ( 'NONE', ( #26904 ), #7810, .F. ) ;
#28432=CARTESIAN_POINT ( 'NONE',  ( -3.835137251120299684, 29.44922644035488446, 13.00000000000000178 ) ) ;
#28433=ORIENTED_EDGE ( 'NONE', *, *, #11517, .T. ) ;
#28437=ORIENTED_EDGE ( 'NONE', *, *, #26694, .T. ) ;
#28439=TOROIDAL_SURFACE ( 'NONE', #23928, 16.00000000000000000, 2.000000000000000000 ) ;
#28440=DIRECTION ( 'NONE',  ( 1.000000000000000000, 0.000000000000000000, 0.000000000000000000 ) ) ;
#28444=FACE_OUTER_BOUND ( 'NONE', #23173, .T. ) ;
#28445=ORIENTED_EDGE ( 'NONE', *, *, #8508, .F. ) ;
#28446=CARTESIAN_POINT ( 'NONE',  ( -3.370709253380788084E-06, 22.50000000000031264, 6.000000000000000000 ) ) ;
#28448=DIRECTION ( 'NONE',  ( 1.000000000000000000, 0.000000000000000000, 0.000000000000000000 ) ) ;
#28449=LINE ( 'NONE', #625, #5879 ) ;
#28457=AXIS2_PLACEMENT_3D ( 'NONE', #4810, #38530, #11315 ) ;
#28458=ORIENTED_EDGE ( 'NONE', *, *, #466, .T. ) ;
#28469=FACE_BOUND ( 'NONE', #19569, .T. ) ;
#28473=ORIENTED_EDGE ( 'NONE', *, *, #13131, .F. ) ;
#28475=FACE_OUTER_BOUND ( 'NONE', #19458, .T. ) ;
#28480=VERTEX_POINT ( 'NONE', #40036 ) ;
#28486=CARTESIAN_POINT ( 'NONE',  ( 1.265502442671760264, 36.24516302788250499, 13.00000000000000178 ) ) ;
#28488=AXIS2_PLACEMENT_3D ( 'NONE', #19409, #7966, #14064 ) ;
#28490=DIRECTION ( 'NONE',  ( -1.000000000000000000, 0.000000000000000000, 0.000000000000000000 ) ) ;
#28496=EDGE_CURVE ( 'NONE', #9639, #2436, #16264, .T. ) ;
#28511=ORIENTED_EDGE ( 'NONE', *, *, #17665, .T. ) ;
#28520=DIRECTION ( 'NONE',  ( 1.000000000000000000, 0.000000000000000000, 0.000000000000000000 ) ) ;
#28524=CARTESIAN_POINT ( 'NONE',  ( 12.14716901145161643, 12.46304090461738667, 13.00000000000000178 ) ) ;
#28527=VECTOR ( 'NONE', #24356, 1000.000000000000000 ) ;
#28529=EDGE_CURVE ( 'NONE', #16598, #32934, #2637, .T. ) ;
#28536=CARTESIAN_POINT ( 'NONE',  ( -11.78894649379783388, 21.72623886970244911, 13.00000000000000178 ) ) ;
#28542=CARTESIAN_POINT ( 'NONE',  ( -9.806982162272253944, 13.84996144622306247, 12.00000000000000000 ) ) ;
#28548=CARTESIAN_POINT ( 'NONE',  ( 9.183240348400453001, 28.21559575157615996, 6.000000000000000000 ) ) ;
#28553=DIRECTION ( 'NONE',  ( 0.000000000000000000, 0.000000000000000000, 1.000000000000000000 ) ) ;
#28565=ORIENTED_EDGE ( 'NONE', *, *, #33374, .T. ) ;
#28577=ORIENTED_EDGE ( 'NONE', *, *, #29376, .T. ) ;
#28580=ORIENTED_EDGE ( 'NONE', *, *, #2395, .F. ) ;
#28583=EDGE_CURVE ( 'NONE', #25424, #25284, #3668, .T. ) ;
#28591=DIRECTION ( 'NONE',  ( 0.000000000000000000, 0.000000000000000000, 1.000000000000000000 ) ) ;
#28593=CARTESIAN_POINT ( 'NONE',  ( 1.247466774197339978, 28.36888560440311480, 6.000000000000000000 ) ) ;
#28594=EDGE_LOOP ( 'NONE', ( #6204, #33847, #16806, #23876 ) ) ;
#28611=VECTOR ( 'NONE', #19061, 1000.000000000000000 ) ;
#28628=AXIS2_PLACEMENT_3D ( 'NONE', #33162, #8366, #27247 ) ;
#28629=LINE ( 'NONE', #7697, #17425 ) ;
#28630=EDGE_CURVE ( 'NONE', #22096, #19611, #28449, .T. ) ;
#28634=DIRECTION ( 'NONE',  ( 1.000000000000000000, 0.000000000000000000, 0.000000000000000000 ) ) ;
#28635=VERTEX_POINT ( 'NONE', #30907 ) ;
#28637=ADVANCED_FACE ( 'NONE', ( #25206 ), #9773, .F. ) ;
#28638=ORIENTED_EDGE ( 'NONE', *, *, #13515, .T. ) ;
#28643=CARTESIAN_POINT ( 'NONE',  ( 5.706335727061685681, 24.35410196624994583, 13.00000000000000178 ) ) ;
#28648=LINE ( 'NONE', #3470, #29904 ) ;
#28652=AXIS2_PLACEMENT_3D ( 'NONE', #32308, #8113, #16465 ) ;
#28653=ORIENTED_EDGE ( 'NONE', *, *, #36473, .T. ) ;
#28659=ORIENTED_EDGE ( 'NONE', *, *, #9911, .T. ) ;
#28664=CYLINDRICAL_SURFACE ( 'NONE', #8200, 1.000000000000000000 ) ;
#28666=ORIENTED_EDGE ( 'NONE', *, *, #13832, .T. ) ;
#28669=FACE_BOUND ( 'NONE', #24604, .T. ) ;
#28674=FACE_OUTER_BOUND ( 'NONE', #35452, .T. ) ;
#28680=ORIENTED_EDGE ( 'NONE', *, *, #16819, .T. ) ;
#28693=FACE_BOUND ( 'NONE', #18749, .T. ) ;
#28699=ORIENTED_EDGE ( 'NONE', *, *, #30211, .T. ) ;
#28700=EDGE_CURVE ( 'NONE', #13627, #33602, #18874, .T. ) ;
#28710=VERTEX_POINT ( 'NONE', #22346 ) ;
#28715=CIRCLE ( 'NONE', #15753, 1.000000000000000000 ) ;
#28716=ORIENTED_EDGE ( 'NONE', *, *, #34900, .T. ) ;
#28719=DIRECTION ( 'NONE',  ( 1.000000000000000000, 0.000000000000000000, 0.000000000000000000 ) ) ;
#28721=ORIENTED_EDGE ( 'NONE', *, *, #7146, .T. ) ;
#28723=CARTESIAN_POINT ( 'NONE',  ( -2.587667106213709101, 35.31811204475769728, 12.00000000000000000 ) ) ;
#28729=EDGE_CURVE ( 'NONE', #14474, #21424, #684, .T. ) ;
#28734=CARTESIAN_POINT ( 'NONE',  ( -8.312041872459065672, 25.58773265502866678, 13.00000000000000178 ) ) ;
#28735=EDGE_CURVE ( 'NONE', #19934, #20723, #29451, .T. ) ;
#28737=FACE_OUTER_BOUND ( 'NONE', #12864, .T. ) ;
#28738=VECTOR ( 'NONE', #29260, 1000.000000000000000 ) ;
#28741=DIRECTION ( 'NONE',  ( 0.000000000000000000, 0.000000000000000000, 1.000000000000000000 ) ) ;
#28742=ORIENTED_EDGE ( 'NONE', *, *, #14385, .T. ) ;
#28744=AXIS2_PLACEMENT_3D ( 'NONE', #1091, #4330, #16127 ) ;
#28751=ADVANCED_FACE ( 'NONE', ( #7107 ), #4266, .F. ) ;
#28754=ORIENTED_EDGE ( 'NONE', *, *, #36102, .F. ) ;
#28762=ORIENTED_EDGE ( 'NONE', *, *, #30757, .F. ) ;
#28764=EDGE_LOOP ( 'NONE', ( #16193, #13827, #28653, #31876 ) ) ;
#28768=VECTOR ( 'NONE', #2339, 1000.000000000000000 ) ;
#28783=ORIENTED_EDGE ( 'NONE', *, *, #1665, .T. ) ;
#28787=FACE_OUTER_BOUND ( 'NONE', #15293, .T. ) ;
#28791=ORIENTED_EDGE ( 'NONE', *, *, #24041, .T. ) ;
#28794=DIRECTION ( 'NONE',  ( 1.000000000000000000, 0.000000000000000000, 0.000000000000000000 ) ) ;
#28799=CARTESIAN_POINT ( 'NONE',  ( 1.494936919103933226, 34.23777120880591696, 12.00000000000000000 ) ) ;
#28800=DIRECTION ( 'NONE',  ( 0.000000000000000000, 0.000000000000000000, 1.000000000000000000 ) ) ;
#28817=AXIS2_PLACEMENT_3D ( 'NONE', #9262, #6208, #14260 ) ;
#28823=CARTESIAN_POINT ( 'NONE',  ( 6.348106467989403257, 35.16482219193073178, 6.000000000000000000 ) ) ;
#28830=DIRECTION ( 'NONE',  ( 0.000000000000000000, 0.000000000000000000, 1.000000000000000000 ) ) ;
#28834=FACE_OUTER_BOUND ( 'NONE', #20672, .T. ) ;
#28835=ORIENTED_EDGE ( 'NONE', *, *, #17489, .T. ) ;
#28853=ORIENTED_EDGE ( 'NONE', *, *, #14027, .T. ) ;
#28855=LINE ( 'NONE', #38203, #21415 ) ;
#28859=DIRECTION ( 'NONE',  ( 0.000000000000000000, 0.000000000000000000, 1.000000000000000000 ) ) ;
#28867=EDGE_CURVE ( 'NONE', #12667, #8857, #8497, .T. ) ;
#28868=ORIENTED_EDGE ( 'NONE', *, *, #10861, .T. ) ;
#28871=MECHANICAL_DESIGN_GEOMETRIC_PRESENTATION_REPRESENTATION('',(#976),#4217);
#28872=DIRECTION ( 'NONE',  ( 0.000000000000000000, 0.000000000000000000, 1.000000000000000000 ) ) ;
#28873=FACE_BOUND ( 'NONE', #37141, .T. ) ;
#28883=ORIENTED_EDGE ( 'NONE', *, *, #25970, .F. ) ;
#28891=FACE_OUTER_BOUND ( 'NONE', #13134, .T. ) ;
#28899=FACE_BOUND ( 'NONE', #6373, .T. ) ;
#28906=ORIENTED_EDGE ( 'NONE', *, *, #34748, .F. ) ;
#28918=CARTESIAN_POINT ( 'NONE',  ( 8.293999462566144842, 11.53598992149257008, 6.000000000000000000 ) ) ;
#28919=ORIENTED_EDGE ( 'NONE', *, *, #26517, .F. ) ;
#28924=ORIENTED_EDGE ( 'NONE', *, *, #186, .F. ) ;
#28931=AXIS2_PLACEMENT_3D ( 'NONE', #37248, #25252, #31347 ) ;
#28932=AXIS2_PLACEMENT_3D ( 'NONE', #9880, #9090, #22261 ) ;
#28935=EDGE_CURVE ( 'NONE', #15766, #11791, #19503, .T. ) ;
#28939=DIRECTION ( 'NONE',  ( 0.000000000000000000, 0.000000000000000000, 1.000000000000000000 ) ) ;
#28948=DIRECTION ( 'NONE',  ( 0.000000000000000000, 0.000000000000000000, 1.000000000000000000 ) ) ;
#28958=AXIS2_PLACEMENT_3D ( 'NONE', #4374, #16780, #23470 ) ;
#28959=EDGE_CURVE ( 'NONE', #8671, #5684, #7171, .T. ) ;
#28967=DIRECTION ( 'NONE',  ( 0.000000000000000000, 0.000000000000000000, 1.000000000000000000 ) ) ;
#28990=AXIS2_PLACEMENT_3D ( 'NONE', #16844, #32070, #10740 ) ;
#28993=DIRECTION ( 'NONE',  ( 0.000000000000000000, 0.000000000000000000, 1.000000000000000000 ) ) ;
#28994=CARTESIAN_POINT ( 'NONE',  ( 9.917734535019443243, 14.47043272369397116, 13.00000000000000178 ) ) ;
#28995=CYLINDRICAL_SURFACE ( 'NONE', #14264, 1.000000000000000000 ) ;
#28996=EDGE_LOOP ( 'NONE', ( #17057, #972, #3343, #34610 ) ) ;
#28998=DIRECTION ( 'NONE',  ( 1.000000000000000000, 0.000000000000000000, 0.000000000000000000 ) ) ;
#29000=DIRECTION ( 'NONE',  ( 0.000000000000000000, 0.000000000000000000, 1.000000000000000000 ) ) ;
#29001=CARTESIAN_POINT ( 'NONE',  ( 15.26584437371809955, 27.13525491562438319, 6.000000000000000000 ) ) ;
#29007=ORIENTED_EDGE ( 'NONE', *, *, #36853, .T. ) ;
#29028=ORIENTED_EDGE ( 'NONE', *, *, #7146, .F. ) ;
#29045=CIRCLE ( 'NONE', #27103, 1.000000000000000888 ) ;
#29047=VERTEX_POINT ( 'NONE', #33321 ) ;
#29050=DIRECTION ( 'NONE',  ( 0.000000000000000000, 0.000000000000000000, 1.000000000000000000 ) ) ;
#29063=VERTEX_POINT ( 'NONE', #2037 ) ;
#29072=FACE_BOUND ( 'NONE', #16698, .T. ) ;
#29074=AXIS2_PLACEMENT_3D ( 'NONE', #29933, #1916, #33404 ) ;
#29079=FACE_OUTER_BOUND ( 'NONE', #21253, .T. ) ;
#29081=VECTOR ( 'NONE', #8007, 1000.000000000000000 ) ;
#29097=DIRECTION ( 'NONE',  ( 1.000000000000000000, 0.000000000000000000, 0.000000000000000000 ) ) ;
#29100=AXIS2_PLACEMENT_3D ( 'NONE', #33802, #23300, #13744 ) ;
#29101=CIRCLE ( 'NONE', #5096, 1.000000000000000888 ) ;
#29110=EDGE_LOOP ( 'NONE', ( #32072, #3942, #35942, #36073 ) ) ;
#29118=CARTESIAN_POINT ( 'NONE',  ( 3.229431105722923245, 20.49260818092372460, 12.00000000000000000 ) ) ;
#29131=CARTESIAN_POINT ( 'NONE',  ( -1.000003370709253492, 22.50000000000031264, 12.00000000000000000 ) ) ;
#29140=VERTEX_POINT ( 'NONE', #37151 ) ;
#29145=CYLINDRICAL_SURFACE ( 'NONE', #38774, 1.000000000000000888 ) ;
#29148=EDGE_CURVE ( 'NONE', #18344, #11394, #577, .T. ) ;
#29149=DIRECTION ( 'NONE',  ( 0.000000000000000000, 0.000000000000000000, 1.000000000000000000 ) ) ;
#29154=DIRECTION ( 'NONE',  ( 0.000000000000000000, 0.000000000000000000, 1.000000000000000000 ) ) ;
#29165=EDGE_CURVE ( 'NONE', #11380, #25337, #13700, .T. ) ;
#29170=ORIENTED_EDGE ( 'NONE', *, *, #23510, .T. ) ;
#29174=EDGE_LOOP ( 'NONE', ( #1422, #36681 ) ) ;
#29187=ORIENTED_EDGE ( 'NONE', *, *, #23154, .T. ) ;
#29197=ORIENTED_EDGE ( 'NONE', *, *, #17845, .T. ) ;
#29201=DIRECTION ( 'NONE',  ( 0.000000000000000000, 0.000000000000000000, 1.000000000000000000 ) ) ;
#29204=DIRECTION ( 'NONE',  ( 1.000000000000000000, 0.000000000000000000, 0.000000000000000000 ) ) ;
#29214=DIRECTION ( 'NONE',  ( 0.000000000000000000, 0.000000000000000000, 1.000000000000000000 ) ) ;
#29235=DIRECTION ( 'NONE',  ( 1.000000000000000000, 0.000000000000000000, 0.000000000000000000 ) ) ;
#29245=EDGE_LOOP ( 'NONE', ( #22981, #18436 ) ) ;
#29247=CARTESIAN_POINT ( 'NONE',  ( -10.14717575287011542, 32.53695909538323860, 13.00000000000000178 ) ) ;
#29248=DIRECTION ( 'NONE',  ( 1.000000000000000000, 0.000000000000000000, 0.000000000000000000 ) ) ;
#29251=DIRECTION ( 'NONE',  ( 0.000000000000000000, 0.000000000000000000, 1.000000000000000000 ) ) ;
#29252=VERTEX_POINT ( 'NONE', #6066 ) ;
#29254=DIRECTION ( 'NONE',  ( 1.000000000000000000, 0.000000000000000000, 0.000000000000000000 ) ) ;
#29259=EDGE_LOOP ( 'NONE', ( #17905, #12232 ) ) ;
#29260=DIRECTION ( 'NONE',  ( 0.000000000000000000, 0.000000000000000000, 1.000000000000000000 ) ) ;
#29261=CARTESIAN_POINT ( 'NONE',  ( -12.41268156625113406, 18.79179606750104981, 12.00000000000000000 ) ) ;
#29272=CIRCLE ( 'NONE', #7213, 1.000000000000000888 ) ;
#29278=DIRECTION ( 'NONE',  ( 1.000000000000000000, 0.000000000000000000, -0.000000000000000000 ) ) ;
#29280=DIRECTION ( 'NONE',  ( 1.000000000000000000, 0.000000000000000000, 0.000000000000000000 ) ) ;
#29284=CYLINDRICAL_SURFACE ( 'NONE', #7022, 1.000000000000000000 ) ;
#29285=CARTESIAN_POINT ( 'NONE',  ( -3.211402178667006169, 32.38366924255629442, 12.00000000000000000 ) ) ;
#29289=EDGE_CURVE ( 'NONE', #10554, #29357, #34505, .T. ) ;
#29290=EDGE_LOOP ( 'NONE', ( #8096, #18190 ) ) ;
#29294=EDGE_CURVE ( 'NONE', #708, #19619, #9724, .T. ) ;
#29303=FACE_OUTER_BOUND ( 'NONE', #34371, .T. ) ;
#29305=DIRECTION ( 'NONE',  ( 1.000000000000000000, 0.000000000000000000, 0.000000000000000000 ) ) ;
#29314=ORIENTED_EDGE ( 'NONE', *, *, #11618, .F. ) ;
#29319=VERTEX_POINT ( 'NONE', #4419 ) ;
#29332=ORIENTED_EDGE ( 'NONE', *, *, #14261, .F. ) ;
#29340=ORIENTED_EDGE ( 'NONE', *, *, #29393, .T. ) ;
#29346=CYLINDRICAL_SURFACE ( 'NONE', #21423, 1.000000000000000888 ) ;
#29347=DIRECTION ( 'NONE',  ( 1.000000000000000000, 0.000000000000000000, 0.000000000000000000 ) ) ;
#29354=DIRECTION ( 'NONE',  ( 1.000000000000000000, 0.000000000000000000, 0.000000000000000000 ) ) ;
#29357=VERTEX_POINT ( 'NONE', #977 ) ;
#29360=EDGE_CURVE ( 'NONE', #24105, #36787, #3816, .T. ) ;
#29361=AXIS2_PLACEMENT_3D ( 'NONE', #28432, #19487, #3453 ) ;
#29367=EDGE_LOOP ( 'NONE', ( #32586, #1287, #37239, #25183 ) ) ;
#29376=EDGE_CURVE ( 'NONE', #35634, #5931, #27976, .T. ) ;
#29377=VERTEX_POINT ( 'NONE', #7254 ) ;
#29380=DIRECTION ( 'NONE',  ( 0.000000000000000000, 0.000000000000000000, 1.000000000000000000 ) ) ;
#29382=CARTESIAN_POINT ( 'NONE',  ( -1.247473515615844075, 16.63111439559750693, 6.000000000000000000 ) ) ;
#29389=CARTESIAN_POINT ( 'NONE',  ( 5.706335727061685681, 24.35410196624994583, 12.00000000000000000 ) ) ;
#29391=CIRCLE ( 'NONE', #33923, 1.000000000000000000 ) ;
#29393=EDGE_CURVE ( 'NONE', #36335, #30133, #1377, .T. ) ;
#29394=ORIENTED_EDGE ( 'NONE', *, *, #16052, .T. ) ;
#29398=AXIS2_PLACEMENT_3D ( 'NONE', #25196, #812, #28440 ) ;
#29399=DIRECTION ( 'NONE',  ( 0.000000000000000000, 0.000000000000000000, 1.000000000000000000 ) ) ;
#29400=ORIENTED_EDGE ( 'NONE', *, *, #30624, .T. ) ;
#29404=CARTESIAN_POINT ( 'NONE',  ( -1.605702774688126722, 27.44183462127829642, 13.00000000000000178 ) ) ;
#29434=EDGE_LOOP ( 'NONE', ( #31765, #18543, #40069, #24631 ) ) ;
#29443=EDGE_CURVE ( 'NONE', #4065, #7337, #5271, .T. ) ;
#29448=ORIENTED_EDGE ( 'NONE', *, *, #2442, .F. ) ;
#29449=DIRECTION ( 'NONE',  ( 1.000000000000000000, 0.000000000000000000, 0.000000000000000000 ) ) ;
#29450=DIRECTION ( 'NONE',  ( 0.000000000000000000, 0.000000000000000000, 1.000000000000000000 ) ) ;
#29451=LINE ( 'NONE', #16670, #23401 ) ;
#29459=LINE ( 'NONE', #23767, #8747 ) ;
#29464=AXIS2_PLACEMENT_3D ( 'NONE', #7562, #10821, #19963 ) ;
#29471=ORIENTED_EDGE ( 'NONE', *, *, #29289, .F. ) ;
#29474=FACE_BOUND ( 'NONE', #37620, .T. ) ;
#29492=ORIENTED_EDGE ( 'NONE', *, *, #7887, .F. ) ;
#29494=EDGE_CURVE ( 'NONE', #2390, #32551, #35758, .T. ) ;
#29508=CARTESIAN_POINT ( 'NONE',  ( -2.853172919594720192, 21.57294901687549427, 13.00000000000000178 ) ) ;
#29512=ORIENTED_EDGE ( 'NONE', *, *, #10548, .T. ) ;
#29515=ORIENTED_EDGE ( 'NONE', *, *, #31009, .T. ) ;
#29519=CARTESIAN_POINT ( 'NONE',  ( -8.541476348891238857, 27.59512447410525127, 6.000000000000000000 ) ) ;
#29549=CARTESIAN_POINT ( 'NONE',  ( -5.440836655099179353, 34.39106106163288246, 12.00000000000000000 ) ) ;
#29553=ORIENTED_EDGE ( 'NONE', *, *, #20464, .T. ) ;
#29558=CARTESIAN_POINT ( 'NONE',  ( 1.587660364795204782, 9.681887955242936883, 6.000000000000000000 ) ) ;
#29561=DIRECTION ( 'NONE',  ( 1.000000000000000000, 0.000000000000000000, 0.000000000000000000 ) ) ;
#29562=ORIENTED_EDGE ( 'NONE', *, *, #24791, .T. ) ;
#29566=DIRECTION ( 'NONE',  ( 0.000000000000000000, 0.000000000000000000, 1.000000000000000000 ) ) ;
#29569=DIRECTION ( 'NONE',  ( 0.000000000000000000, 0.000000000000000000, 1.000000000000000000 ) ) ;
#29575=CIRCLE ( 'NONE', #12057, 1.000000000000000888 ) ;
#29583=DIRECTION ( 'NONE',  ( 0.000000000000000000, 0.000000000000000000, 1.000000000000000000 ) ) ;
#29595=CARTESIAN_POINT ( 'NONE',  ( 1.605696033269625955, 17.55816537872232530, 13.00000000000000178 ) ) ;
#29596=CIRCLE ( 'NONE', #34788, 1.000000000000000000 ) ;
#29599=VERTEX_POINT ( 'NONE', #30421 ) ;
#29600=ADVANCED_FACE ( 'NONE', ( #14370 ), #24312, .F. ) ;
#29603=AXIS2_PLACEMENT_3D ( 'NONE', #34862, #13111, #25706 ) ;
#29606=DIRECTION ( 'NONE',  ( 0.000000000000000000, 0.000000000000000000, 1.000000000000000000 ) ) ;
#29610=CARTESIAN_POINT ( 'NONE',  ( -9.165211421344535481, 24.66068167190384841, 13.00000000000000178 ) ) ;
#29613=DIRECTION ( 'NONE',  ( 1.000000000000000000, 0.000000000000000000, 0.000000000000000000 ) ) ;
#29630=AXIS2_PLACEMENT_3D ( 'NONE', #30190, #5204, #24091 ) ;
#29638=ORIENTED_EDGE ( 'NONE', *, *, #25872, .F. ) ;
#29645=CARTESIAN_POINT ( 'NONE',  ( -7.935776944912362296, 22.65328985282726393, 6.000000000000000000 ) ) ;
#29648=DIRECTION ( 'NONE',  ( 1.000000000000000000, 0.000000000000000000, 0.000000000000000000 ) ) ;
#29661=CYLINDRICAL_SURFACE ( 'NONE', #14927, 1.000000000000000000 ) ;
#29682=DIRECTION ( 'NONE',  ( 0.000000000000000000, 0.000000000000000000, 1.000000000000000000 ) ) ;
#29685=ORIENTED_EDGE ( 'NONE', *, *, #32764, .T. ) ;
#29697=EDGE_CURVE ( 'NONE', #10198, #15741, #37469, .T. ) ;
#29699=AXIS2_PLACEMENT_3D ( 'NONE', #37278, #9452, #21832 ) ;
#29700=DIRECTION ( 'NONE',  ( 0.000000000000000000, 0.000000000000000000, 1.000000000000000000 ) ) ;
#29701=ORIENTED_EDGE ( 'NONE', *, *, #14619, .F. ) ;
#29712=ORIENTED_EDGE ( 'NONE', *, *, #36181, .F. ) ;
#29717=CIRCLE ( 'NONE', #12202, 1.000000000000000000 ) ;
#29729=EDGE_CURVE ( 'NONE', #27275, #17659, #14741, .T. ) ;
#29730=ORIENTED_EDGE ( 'NONE', *, *, #38781, .F. ) ;
#29735=ORIENTED_EDGE ( 'NONE', *, *, #70, .T. ) ;
#29746=EDGE_CURVE ( 'NONE', #32987, #16453, #8913, .T. ) ;
#29754=ADVANCED_FACE ( 'NONE', ( #5619 ), #36313, .F. ) ;
#29755=DIRECTION ( 'NONE',  ( 0.000000000000000000, 0.000000000000000000, 1.000000000000000000 ) ) ;
#29766=ORIENTED_EDGE ( 'NONE', *, *, #18466, .F. ) ;
#29776=DIRECTION ( 'NONE',  ( 1.000000000000000000, 0.000000000000000000, 0.000000000000000000 ) ) ;
#29781=AXIS2_PLACEMENT_3D ( 'NONE', #34266, #31018, #34462 ) ;
#29785=ORIENTED_EDGE ( 'NONE', *, *, #33279, .T. ) ;
#29788=CARTESIAN_POINT ( 'NONE',  ( -13.01838097023000707, 23.73363068877903359, 6.000000000000000000 ) ) ;
#29795=LINE ( 'NONE', #1564, #21339 ) ;
#29800=DIRECTION ( 'NONE',  ( 1.000000000000000000, 0.000000000000000000, 0.000000000000000000 ) ) ;
#29805=DIRECTION ( 'NONE',  ( 0.000000000000000000, 0.000000000000000000, 1.000000000000000000 ) ) ;
#29806=CARTESIAN_POINT ( 'NONE',  ( 12.41267482483262796, 26.20820393249957192, 13.00000000000000178 ) ) ;
#29810=CYLINDRICAL_SURFACE ( 'NONE', #30093, 1.000000000000000888 ) ;
#29826=LINE ( 'NONE', #2011, #13440 ) ;
#29827=EDGE_CURVE ( 'NONE', #5736, #24952, #2977, .T. ) ;
#29831=CIRCLE ( 'NONE', #35665, 1.000000000000000000 ) ;
#29833=VERTEX_POINT ( 'NONE', #34058 ) ;
#29834=CARTESIAN_POINT ( 'NONE',  ( 8.917734535019441466, 14.47043272369397116, 12.00000000000000000 ) ) ;
#29836=CIRCLE ( 'NONE', #2584, 1.000000000000000888 ) ;
#29837=ORIENTED_EDGE ( 'NONE', *, *, #18379, .F. ) ;
#29848=DIRECTION ( 'NONE',  ( 0.000000000000000000, 0.000000000000000000, 1.000000000000000000 ) ) ;
#29849=ORIENTED_EDGE ( 'NONE', *, *, #32363, .F. ) ;
#29852=ADVANCED_FACE ( 'NONE', ( #28152 ), #15167, .F. ) ;
#29866=EDGE_CURVE ( 'NONE', #2121, #1690, #1777, .T. ) ;
#29867=CARTESIAN_POINT ( 'NONE',  ( 5.082600654608392610, 21.41965916404854298, 13.00000000000000178 ) ) ;
#29872=DIRECTION ( 'NONE',  ( 1.000000000000000000, 0.000000000000000000, 0.000000000000000000 ) ) ;
#29875=DIRECTION ( 'NONE',  ( 0.000000000000000000, 0.000000000000000000, 1.000000000000000000 ) ) ;
#29892=AXIS2_PLACEMENT_3D ( 'NONE', #16966, #27854, #9374 ) ;
#29897=ORIENTED_EDGE ( 'NONE', *, *, #18510, .T. ) ;
#29904=VECTOR ( 'NONE', #820, 1000.000000000000000 ) ;
#29910=DIRECTION ( 'NONE',  ( 1.000000000000000000, 0.000000000000000000, 0.000000000000000000 ) ) ;
#29914=EDGE_LOOP ( 'NONE', ( #18269, #6191, #6763, #14287 ) ) ;
#29919=ORIENTED_EDGE ( 'NONE', *, *, #25561, .T. ) ;
#29921=ORIENTED_EDGE ( 'NONE', *, *, #5509, .T. ) ;
#29931=EDGE_LOOP ( 'NONE', ( #19659, #36736, #16607, #32098 ) ) ;
#29933=CARTESIAN_POINT ( 'NONE',  ( 8.917734535019441466, 14.47043272369397116, 6.000000000000000000 ) ) ;
#29934=CARTESIAN_POINT ( 'NONE',  ( -0.7344975573282397363, 36.24516302788250499, 6.000000000000000000 ) ) ;
#29945=DIRECTION ( 'NONE',  ( 1.000000000000000000, 0.000000000000000000, 0.000000000000000000 ) ) ;
#29947=EDGE_CURVE ( 'NONE', #8857, #10191, #34259, .T. ) ;
#29949=CARTESIAN_POINT ( 'NONE',  ( -4.458872323573595864, 26.51478363815348160, 13.00000000000000178 ) ) ;
#29965=DIRECTION ( 'NONE',  ( 0.000000000000000000, 0.000000000000000000, 1.000000000000000000 ) ) ;
#29969=ORIENTED_EDGE ( 'NONE', *, *, #7509, .T. ) ;
#29977=CARTESIAN_POINT ( 'NONE',  ( -9.788946493797832105, 21.72623886970244911, 12.00000000000000000 ) ) ;
#29982=DIRECTION ( 'NONE',  ( 0.000000000000000000, 0.000000000000000000, 1.000000000000000000 ) ) ;
#29986=CARTESIAN_POINT ( 'NONE',  ( 12.39463915635820612, 18.33192650902018883, 12.00000000000000000 ) ) ;
#29990=EDGE_CURVE ( 'NONE', #23748, #9924, #16164, .T. ) ;
#29991=VECTOR ( 'NONE', #35028, 1000.000000000000000 ) ;
#29992=DIRECTION ( 'NONE',  ( 0.000000000000000000, 0.000000000000000000, 1.000000000000000000 ) ) ;
#29994=CARTESIAN_POINT ( 'NONE',  ( 1.981960960816328887, 14.62372257652092422, 13.00000000000000178 ) ) ;
#30001=ADVANCED_FACE ( 'NONE', ( #22244 ), #19607, .F. ) ;
#30003=DIRECTION ( 'NONE',  ( 0.000000000000000000, 0.000000000000000000, 1.000000000000000000 ) ) ;
#30009=CARTESIAN_POINT ( 'NONE',  ( 16.99999999999999645, 22.50000000000000711, 11.00000000000000178 ) ) ;
#30011=CARTESIAN_POINT ( 'NONE',  ( 10.16520467992603294, 20.33931832809677331, 12.00000000000000000 ) ) ;
#30018=DIRECTION ( 'NONE',  ( 1.000000000000000000, 0.000000000000000000, 0.000000000000000000 ) ) ;
#30036=ORIENTED_EDGE ( 'NONE', *, *, #20302, .F. ) ;
#30039=EDGE_LOOP ( 'NONE', ( #1647, #34665 ) ) ;
#30040=CARTESIAN_POINT ( 'NONE',  ( -1.981967702234832984, 30.37627742347970283, 6.000000000000000000 ) ) ;
#30042=CARTESIAN_POINT ( 'NONE',  ( -1.229437847141422901, 24.50739181907689712, 13.00000000000000178 ) ) ;
#30049=ORIENTED_EDGE ( 'NONE', *, *, #7887, .T. ) ;
#30055=AXIS2_PLACEMENT_3D ( 'NONE', #3363, #12701, #9069 ) ;
#30063=VERTEX_POINT ( 'NONE', #23056 ) ;
#30067=( GEOMETRIC_REPRESENTATION_CONTEXT ( 3 ) GLOBAL_UNCERTAINTY_ASSIGNED_CONTEXT ( ( #24034 ) ) GLOBAL_UNIT_ASSIGNED_CONTEXT ( ( #14816, #40032, #16665 ) ) REPRESENTATION_CONTEXT ( 'NONE', 'WORKASPACE' ) );
#30070=DIRECTION ( 'NONE',  ( 1.000000000000000000, 0.000000000000000000, 0.000000000000000000 ) ) ;
#30073=VECTOR ( 'NONE', #31099, 1000.000000000000000 ) ;
#30081=VECTOR ( 'NONE', #23657, 1000.000000000000000 ) ;
#30085=CARTESIAN_POINT ( 'NONE',  ( 4.835130509701799362, 15.55077355964573904, 6.000000000000000000 ) ) ;
#30091=ORIENTED_EDGE ( 'NONE', *, *, #26900, .F. ) ;
#30093=AXIS2_PLACEMENT_3D ( 'NONE', #1582, #4220, #23715 ) ;
#30095=EDGE_LOOP ( 'NONE', ( #24439, #5581, #23643, #1708 ) ) ;
#30103=VERTEX_POINT ( 'NONE', #31799 ) ;
#30109=VECTOR ( 'NONE', #39746, 1000.000000000000000 ) ;
#30110=EDGE_CURVE ( 'NONE', #16796, #5069, #32286, .T. ) ;
#30125=EDGE_LOOP ( 'NONE', ( #14202, #26175, #20107, #2740 ) ) ;
#30132=CIRCLE ( 'NONE', #37256, 1.000000000000000000 ) ;
#30133=VERTEX_POINT ( 'NONE', #22849 ) ;
#30151=AXIS2_PLACEMENT_3D ( 'NONE', #18281, #9130, #33533 ) ;
#30159=CARTESIAN_POINT ( 'NONE',  ( 16.99999999999999645, 22.50000000000000711, 13.00000000000000178 ) ) ;
#30165=LINE ( 'NONE', #29558, #14500 ) ;
#30166=CARTESIAN_POINT ( 'NONE',  ( 6.953805871968278929, 30.22298757065274444, 13.00000000000000178 ) ) ;
#30169=ORIENTED_EDGE ( 'NONE', *, *, #9621, .F. ) ;
#30181=LINE ( 'NONE', #6184, #5615 ) ;
#30182=CIRCLE ( 'NONE', #19793, 1.000000000000000000 ) ;
#30190=CARTESIAN_POINT ( 'NONE',  ( 16.00000000000000000, 22.50000000000000355, 11.00000000000000178 ) ) ;
#30192=DIRECTION ( 'NONE',  ( 0.000000000000000000, 0.000000000000000000, 1.000000000000000000 ) ) ;
#30211=EDGE_CURVE ( 'NONE', #26292, #4871, #38904, .T. ) ;
#30212=CYLINDRICAL_SURFACE ( 'NONE', #35642, 1.000000000000000888 ) ;
#30215=CARTESIAN_POINT ( 'NONE',  ( -2.605702774688126500, 27.44183462127829642, 6.000000000000000000 ) ) ;
#30216=DIRECTION ( 'NONE',  ( 0.000000000000000000, 0.000000000000000000, 1.000000000000000000 ) ) ;
#30220=ORIENTED_EDGE ( 'NONE', *, *, #17240, .F. ) ;
#30221=EDGE_CURVE ( 'NONE', #15652, #34128, #36539, .T. ) ;
#30223=AXIS2_PLACEMENT_3D ( 'NONE', #36776, #33746, #17504 ) ;
#30250=CIRCLE ( 'NONE', #38687, 1.000000000000000888 ) ;
#30251=ORIENTED_EDGE ( 'NONE', *, *, #25596, .T. ) ;
#30253=ORIENTED_EDGE ( 'NONE', *, *, #2219, .T. ) ;
#30257=FACE_OUTER_BOUND ( 'NONE', #7896, .T. ) ;
#30259=EDGE_CURVE ( 'NONE', #34344, #8098, #9310, .T. ) ;
#30267=EDGE_LOOP ( 'NONE', ( #7657, #6101 ) ) ;
#30284=EDGE_CURVE ( 'NONE', #40053, #2398, #30165, .T. ) ;
#30287=EDGE_CURVE ( 'NONE', #13580, #36183, #19016, .T. ) ;
#30296=ORIENTED_EDGE ( 'NONE', *, *, #15922, .T. ) ;
#30304=AXIS2_PLACEMENT_3D ( 'NONE', #11504, #21241, #2366 ) ;
#30306=CARTESIAN_POINT ( 'NONE',  ( 0.000000000000000000, 22.50000000000000355, 11.00000000000000178 ) ) ;
#30313=DIRECTION ( 'NONE',  ( 1.000000000000000000, 0.000000000000000000, 0.000000000000000000 ) ) ;
#30326=VERTEX_POINT ( 'NONE', #4977 ) ;
#30334=VECTOR ( 'NONE', #13127, 1000.000000000000000 ) ;
#30335=ORIENTED_EDGE ( 'NONE', *, *, #2345, .F. ) ;
#30339=ORIENTED_EDGE ( 'NONE', *, *, #25728, .F. ) ;
#30341=EDGE_CURVE ( 'NONE', #10782, #22765, #27113, .T. ) ;
#30352=ORIENTED_EDGE ( 'NONE', *, *, #16352, .T. ) ;
#30358=DIRECTION ( 'NONE',  ( 0.000000000000000000, 0.000000000000000000, 1.000000000000000000 ) ) ;
#30359=AXIS2_PLACEMENT_3D ( 'NONE', #12224, #33177, #37008 ) ;
#30361=AXIS2_PLACEMENT_3D ( 'NONE', #30394, #14345, #5203 ) ;
#30362=FACE_BOUND ( 'NONE', #30858, .T. ) ;
#30366=DIRECTION ( 'NONE',  ( 1.000000000000000000, 0.000000000000000000, 0.000000000000000000 ) ) ;
#30370=CIRCLE ( 'NONE', #23229, 1.000000000000000888 ) ;
#30375=ORIENTED_EDGE ( 'NONE', *, *, #17620, .T. ) ;
#30380=ORIENTED_EDGE ( 'NONE', *, *, #5773, .T. ) ;
#30382=VERTEX_POINT ( 'NONE', #31295 ) ;
#30389=CYLINDRICAL_SURFACE ( 'NONE', #145, 1.000000000000000888 ) ;
#30394=CARTESIAN_POINT ( 'NONE',  ( -0.9819677022348329842, 30.37627742347970283, 13.00000000000000178 ) ) ;
#30397=VERTEX_POINT ( 'NONE', #3859 ) ;
#30412=CYLINDRICAL_SURFACE ( 'NONE', #24269, 1.000000000000000888 ) ;
#30417=ADVANCED_FACE ( 'NONE', ( #15856 ), #34945, .F. ) ;
#30419=ADVANCED_FACE ( 'NONE', ( #19293 ), #34542, .F. ) ;
#30421=CARTESIAN_POINT ( 'NONE',  ( 6.706335727061685681, 24.35410196624994583, 13.00000000000000178 ) ) ;
#30422=CARTESIAN_POINT ( 'NONE',  ( -1.247473515615844075, 16.63111439559750693, 12.00000000000000000 ) ) ;
#30427=CIRCLE ( 'NONE', #12893, 1.000000000000000888 ) ;
#30435=AXIS2_PLACEMENT_3D ( 'NONE', #12259, #22793, #29097 ) ;
#30450=CYLINDRICAL_SURFACE ( 'NONE', #34276, 1.000000000000000000 ) ;
#30455=AXIS2_PLACEMENT_3D ( 'NONE', #9482, #30820, #9082 ) ;
#30458=CARTESIAN_POINT ( 'NONE',  ( 0.000000000000000000, 22.50000000000000355, 11.00000000000000178 ) ) ;
#30464=DIRECTION ( 'NONE',  ( 0.000000000000000000, 0.000000000000000000, 1.000000000000000000 ) ) ;
#30473=DIRECTION ( 'NONE',  ( 1.000000000000000000, 0.000000000000000000, 0.000000000000000000 ) ) ;
#30476=DIRECTION ( 'NONE',  ( 1.000000000000000000, 0.000000000000000000, 0.000000000000000000 ) ) ;
#30483=ORIENTED_EDGE ( 'NONE', *, *, #1825, .F. ) ;
#30484=EDGE_LOOP ( 'NONE', ( #17628, #7033, #7007, #4745 ) ) ;
#30493=EDGE_CURVE ( 'NONE', #34024, #31085, #34590, .T. ) ;
#30494=CARTESIAN_POINT ( 'NONE',  ( -3.118678732975735279, 7.827785988993307242, 12.00000000000000000 ) ) ;
#30510=ORIENTED_EDGE ( 'NONE', *, *, #26514, .F. ) ;
#30511=CARTESIAN_POINT ( 'NONE',  ( -6.953812613386785912, 14.77701242934787906, 12.00000000000000000 ) ) ;
#30517=DIRECTION ( 'NONE',  ( 0.000000000000000000, 0.000000000000000000, 1.000000000000000000 ) ) ;
#30530=FACE_OUTER_BOUND ( 'NONE', #36218, .T. ) ;
#30537=EDGE_CURVE ( 'NONE', #6333, #11673, #21742, .T. ) ;
#30543=ORIENTED_EDGE ( 'NONE', *, *, #31738, .T. ) ;
#30547=DIRECTION ( 'NONE',  ( 0.000000000000000000, 0.000000000000000000, 1.000000000000000000 ) ) ;
#30551=VERTEX_POINT ( 'NONE', #29247 ) ;
#30556=CARTESIAN_POINT ( 'NONE',  ( -8.917741276437942233, 30.52956727630665057, 13.00000000000000178 ) ) ;
#30560=CIRCLE ( 'NONE', #33145, 1.000000000000000888 ) ;
#30561=CARTESIAN_POINT ( 'NONE',  ( 0.000000000000000000, 22.50000000000000355, 11.00000000000000178 ) ) ;
#30562=FACE_BOUND ( 'NONE', #23226, .T. ) ;
#30563=CYLINDRICAL_SURFACE ( 'NONE', #19187, 1.000000000000000000 ) ;
#30566=DIRECTION ( 'NONE',  ( 1.000000000000000000, 0.000000000000000000, 0.000000000000000000 ) ) ;
#30574=VERTEX_POINT ( 'NONE', #1827 ) ;
#30579=ORIENTED_EDGE ( 'NONE', *, *, #1944, .T. ) ;
#30581=DIRECTION ( 'NONE',  ( 1.000000000000000000, 0.000000000000000000, 0.000000000000000000 ) ) ;
#30587=VECTOR ( 'NONE', #17327, 1000.000000000000000 ) ;
#30592=ORIENTED_EDGE ( 'NONE', *, *, #27474, .T. ) ;
#30598=EDGE_LOOP ( 'NONE', ( #35861, #22723, #36896, #10886 ) ) ;
#30604=CARTESIAN_POINT ( 'NONE',  ( 0.6237317017440463518, 25.43444280220171194, 13.00000000000000178 ) ) ;
#30607=AXIS2_PLACEMENT_3D ( 'NONE', #14012, #29050, #23563 ) ;
#30611=CIRCLE ( 'NONE', #13076, 1.000000000000000888 ) ;
#30621=ORIENTED_EDGE ( 'NONE', *, *, #35046, .T. ) ;
#30624=EDGE_CURVE ( 'NONE', #5290, #31950, #22890, .T. ) ;
#30625=DIRECTION ( 'NONE',  ( 0.000000000000000000, 0.000000000000000000, 1.000000000000000000 ) ) ;
#30626=CIRCLE ( 'NONE', #37748, 16.00000000000000000 ) ;
#30645=ORIENTED_EDGE ( 'NONE', *, *, #11083, .T. ) ;
#30649=EDGE_CURVE ( 'NONE', #15047, #11157, #1535, .T. ) ;
#30655=ORIENTED_EDGE ( 'NONE', *, *, #28735, .F. ) ;
#30657=DIRECTION ( 'NONE',  ( -1.000000000000000000, 0.000000000000000000, 0.000000000000000000 ) ) ;
#30658=VECTOR ( 'NONE', #999, 1000.000000000000000 ) ;
#30659=CARTESIAN_POINT ( 'NONE',  ( -1.265509184090266137, 8.754836972118123839, 6.000000000000000000 ) ) ;
#30662=CARTESIAN_POINT ( 'NONE',  ( -10.41268156625113228, 18.79179606750104981, 13.00000000000000178 ) ) ;
#30663=DIRECTION ( 'NONE',  ( 1.000000000000000000, 0.000000000000000000, 0.000000000000000000 ) ) ;
#30665=EDGE_CURVE ( 'NONE', #33664, #9387, #17122, .T. ) ;
#30669=ORIENTED_EDGE ( 'NONE', *, *, #1313, .T. ) ;
#30679=AXIS2_PLACEMENT_3D ( 'NONE', #27239, #30694, #28036 ) ;
#30689=DIRECTION ( 'NONE',  ( 0.000000000000000000, 0.000000000000000000, 1.000000000000000000 ) ) ;
#30692=EDGE_LOOP ( 'NONE', ( #27681, #11358 ) ) ;
#30694=DIRECTION ( 'NONE',  ( 0.000000000000000000, 0.000000000000000000, 1.000000000000000000 ) ) ;
#30695=AXIS2_PLACEMENT_3D ( 'NONE', #15168, #28346, #15366 ) ;
#30705=ORIENTED_EDGE ( 'NONE', *, *, #32462, .F. ) ;
#30708=CARTESIAN_POINT ( 'NONE',  ( -3.835137251120299684, 29.44922644035488446, 6.000000000000000000 ) ) ;
#30713=EDGE_CURVE ( 'NONE', #5055, #18400, #894, .T. ) ;
#30720=CIRCLE ( 'NONE', #21637, 1.000000000000000888 ) ;
#30721=EDGE_LOOP ( 'NONE', ( #4658, #34604 ) ) ;
#30727=ORIENTED_EDGE ( 'NONE', *, *, #11540, .F. ) ;
#30728=EDGE_LOOP ( 'NONE', ( #4597, #26508, #38925, #4865 ) ) ;
#30736=ORIENTED_EDGE ( 'NONE', *, *, #2196, .T. ) ;
#30739=CARTESIAN_POINT ( 'NONE',  ( -14.26585111513660031, 17.86474508437623143, 12.00000000000000000 ) ) ;
#30741=ORIENTED_EDGE ( 'NONE', *, *, #22739, .F. ) ;
#30757=EDGE_CURVE ( 'NONE', #708, #27813, #5421, .T. ) ;
#30759=FACE_BOUND ( 'NONE', #32288, .T. ) ;
#30764=CARTESIAN_POINT ( 'NONE',  ( -7.577547685840081648, 11.84256962714647798, 12.00000000000000000 ) ) ;
#30765=DIRECTION ( 'NONE',  ( 1.000000000000000000, 0.000000000000000000, 0.000000000000000000 ) ) ;
#30769=EDGE_LOOP ( 'NONE', ( #3991, #26674 ) ) ;
#30773=DIRECTION ( 'NONE',  ( 0.000000000000000000, 0.000000000000000000, 1.000000000000000000 ) ) ;
#30777=ORIENTED_EDGE ( 'NONE', *, *, #31891, .F. ) ;
#30801=CARTESIAN_POINT ( 'NONE',  ( -6.064571727552472424, 31.45661825943146894, 12.00000000000000000 ) ) ;
#30803=ORIENTED_EDGE ( 'NONE', *, *, #9565, .F. ) ;
#30809=CARTESIAN_POINT ( 'NONE',  ( -11.41268156625113406, 18.79179606750104981, 12.00000000000000000 ) ) ;
#30810=FACE_OUTER_BOUND ( 'NONE', #9311, .T. ) ;
#30813=DIRECTION ( 'NONE',  ( 1.000000000000000000, 0.000000000000000000, 0.000000000000000000 ) ) ;
#30817=DIRECTION ( 'NONE',  ( 0.000000000000000000, 0.000000000000000000, 1.000000000000000000 ) ) ;
#30820=DIRECTION ( 'NONE',  ( 0.000000000000000000, 0.000000000000000000, 1.000000000000000000 ) ) ;
#30827=CARTESIAN_POINT ( 'NONE',  ( 4.082600654608392610, 21.41965916404854298, 13.00000000000000178 ) ) ;
#30849=CARTESIAN_POINT ( 'NONE',  ( 4.458865582155095986, 18.48521636184714012, 13.00000000000000178 ) ) ;
#30858=EDGE_LOOP ( 'NONE', ( #29562, #30980 ) ) ;
#30861=DIRECTION ( 'NONE',  ( 1.000000000000000000, 0.000000000000000000, 0.000000000000000000 ) ) ;
#30869=EDGE_CURVE ( 'NONE', #20339, #21746, #18414, .T. ) ;
#30871=CYLINDRICAL_SURFACE ( 'NONE', #17838, 1.000000000000000000 ) ;
#30873=DIRECTION ( 'NONE',  ( 0.000000000000000000, 0.000000000000000000, 1.000000000000000000 ) ) ;
#30878=ORIENTED_EDGE ( 'NONE', *, *, #32363, .T. ) ;
#30886=DIRECTION ( 'NONE',  ( 0.000000000000000000, 0.000000000000000000, 1.000000000000000000 ) ) ;
#30887=AXIS2_PLACEMENT_3D ( 'NONE', #4019, #25954, #16421 ) ;
#30888=DIRECTION ( 'NONE',  ( 0.000000000000000000, 0.000000000000000000, 1.000000000000000000 ) ) ;
#30897=EDGE_CURVE ( 'NONE', #17512, #28635, #24552, .T. ) ;
#30899=DIRECTION ( 'NONE',  ( 1.000000000000000000, 0.000000000000000000, 0.000000000000000000 ) ) ;
#30901=DIRECTION ( 'NONE',  ( 0.000000000000000000, 0.000000000000000000, 1.000000000000000000 ) ) ;
#30903=FACE_OUTER_BOUND ( 'NONE', #1902, .T. ) ;
#30907=CARTESIAN_POINT ( 'NONE',  ( -3.724378136954612284, 12.76962061027129458, 13.00000000000000178 ) ) ;
#30911=VECTOR ( 'NONE', #10032, 1000.000000000000000 ) ;
#30918=ORIENTED_EDGE ( 'NONE', *, *, #30284, .T. ) ;
#30928=FACE_BOUND ( 'NONE', #11075, .T. ) ;
#30929=ORIENTED_EDGE ( 'NONE', *, *, #34976, .T. ) ;
#30945=ORIENTED_EDGE ( 'NONE', *, *, #1074, .F. ) ;
#30951=FACE_BOUND ( 'NONE', #30769, .T. ) ;
#30954=DIRECTION ( 'NONE',  ( 1.000000000000000000, 0.000000000000000000, 0.000000000000000000 ) ) ;
#30966=ORIENTED_EDGE ( 'NONE', *, *, #36100, .F. ) ;
#30980=ORIENTED_EDGE ( 'NONE', *, *, #15452, .T. ) ;
#30982=DIRECTION ( 'NONE',  ( 0.000000000000000000, 0.000000000000000000, 1.000000000000000000 ) ) ;
#30994=DIRECTION ( 'NONE',  ( 1.000000000000000000, 0.000000000000000000, 0.000000000000000000 ) ) ;
#30995=AXIS2_PLACEMENT_3D ( 'NONE', #6927, #32338, #35177 ) ;
#30997=EDGE_CURVE ( 'NONE', #15842, #19485, #16470, .T. ) ;
#30998=ORIENTED_EDGE ( 'NONE', *, *, #11386, .T. ) ;
#31003=CARTESIAN_POINT ( 'NONE',  ( -5.064571727552472424, 31.45661825943146894, 13.00000000000000178 ) ) ;
#31009=EDGE_CURVE ( 'NONE', #13548, #12651, #22287, .T. ) ;
#31011=CARTESIAN_POINT ( 'NONE',  ( 10.78893975237932956, 23.27376113029817617, 13.00000000000000178 ) ) ;
#31013=ADVANCED_FACE ( 'NONE', ( #19244 ), #19445, .F. ) ;
#31015=CARTESIAN_POINT ( 'NONE',  ( -12.77091082532341382, 29.60251629318183575, 6.000000000000000000 ) ) ;
#31016=ORIENTED_EDGE ( 'NONE', *, *, #20636, .T. ) ;
#31018=DIRECTION ( 'NONE',  ( 0.000000000000000000, 0.000000000000000000, 1.000000000000000000 ) ) ;
#31025=DIRECTION ( 'NONE',  ( 0.000000000000000000, 0.000000000000000000, 1.000000000000000000 ) ) ;
#31029=CIRCLE ( 'NONE', #18069, 1.000000000000000000 ) ;
#31043=EDGE_LOOP ( 'NONE', ( #28473, #20525, #24891, #1217 ) ) ;
#31046=CYLINDRICAL_SURFACE ( 'NONE', #38821, 1.000000000000000000 ) ;
#31049=ORIENTED_EDGE ( 'NONE', *, *, #337, .T. ) ;
#31051=EDGE_LOOP ( 'NONE', ( #10759, #15530 ) ) ;
#31054=CIRCLE ( 'NONE', #1216, 1.000000000000000888 ) ;
#31072=CARTESIAN_POINT ( 'NONE',  ( -12.39464589777671044, 26.66807349098043289, 12.00000000000000000 ) ) ;
#31082=AXIS2_PLACEMENT_3D ( 'NONE', #11741, #17449, #2006 ) ;
#31085=VERTEX_POINT ( 'NONE', #37544 ) ;
#31094=ORIENTED_EDGE ( 'NONE', *, *, #11585, .T. ) ;
#31099=DIRECTION ( 'NONE',  ( 0.000000000000000000, 0.000000000000000000, 1.000000000000000000 ) ) ;
#31102=FACE_OUTER_BOUND ( 'NONE', #8183, .T. ) ;
#31105=DIRECTION ( 'NONE',  ( 0.000000000000000000, 0.000000000000000000, 1.000000000000000000 ) ) ;
#31106=CARTESIAN_POINT ( 'NONE',  ( -13.01838097023000707, 23.73363068877903359, 13.00000000000000178 ) ) ;
#31114=EDGE_CURVE ( 'NONE', #10357, #28074, #4779, .T. ) ;
#31121=EDGE_CURVE ( 'NONE', #35485, #11948, #22929, .T. ) ;
#31126=FACE_BOUND ( 'NONE', #23649, .T. ) ;
#31131=ORIENTED_EDGE ( 'NONE', *, *, #19715, .F. ) ;
#31133=DIRECTION ( 'NONE',  ( 0.000000000000000000, 0.000000000000000000, 1.000000000000000000 ) ) ;
#31134=CARTESIAN_POINT ( 'NONE',  ( -6.706342468480190000, 20.64589803375067945, 6.000000000000000000 ) ) ;
#31156=LINE ( 'NONE', #9221, #33097 ) ;
#31161=ORIENTED_EDGE ( 'NONE', *, *, #22087, .F. ) ;
#31166=ORIENTED_EDGE ( 'NONE', *, *, #9771, .T. ) ;
#31168=ORIENTED_EDGE ( 'NONE', *, *, #1523, .F. ) ;
#31170=DIRECTION ( 'NONE',  ( 1.000000000000000000, 0.000000000000000000, 0.000000000000000000 ) ) ;
#31172=LINE ( 'NONE', #16536, #30911 ) ;
#31186=CIRCLE ( 'NONE', #5862, 1.000000000000000888 ) ;
#31194=AXIS2_PLACEMENT_3D ( 'NONE', #38596, #19913, #10770 ) ;
#31200=CARTESIAN_POINT ( 'NONE',  ( 10.41267482483262619, 26.20820393249957192, 12.00000000000000000 ) ) ;
#31238=EDGE_CURVE ( 'NONE', #15391, #5046, #35899, .T. ) ;
#31242=CIRCLE ( 'NONE', #31874, 1.000000000000000000 ) ;
#31243=AXIS2_PLACEMENT_3D ( 'NONE', #18709, #12606, #12403 ) ;
#31245=CARTESIAN_POINT ( 'NONE',  ( -16.99999999999999645, 22.50000000000000355, 6.000000000000000000 ) ) ;
#31252=DIRECTION ( 'NONE',  ( 0.000000000000000000, 0.000000000000000000, 1.000000000000000000 ) ) ;
#31257=EDGE_CURVE ( 'NONE', #25284, #29357, #25562, .T. ) ;
#31260=EDGE_LOOP ( 'NONE', ( #28233, #23945, #25610, #25985 ) ) ;
#31262=DIRECTION ( 'NONE',  ( 1.000000000000000000, 0.000000000000000000, 0.000000000000000000 ) ) ;
#31285=CARTESIAN_POINT ( 'NONE',  ( 6.330070799514983193, 27.28854476845134513, 13.00000000000000178 ) ) ;
#31288=FACE_OUTER_BOUND ( 'NONE', #14197, .T. ) ;
#31295=CARTESIAN_POINT ( 'NONE',  ( 12.77090408390491305, 15.39748370681878775, 13.00000000000000178 ) ) ;
#31315=ORIENTED_EDGE ( 'NONE', *, *, #4531, .F. ) ;
#31319=FACE_BOUND ( 'NONE', #35124, .T. ) ;
#31324=VERTEX_POINT ( 'NONE', #35703 ) ;
#31328=ORIENTED_EDGE ( 'NONE', *, *, #18510, .F. ) ;
#31332=AXIS2_PLACEMENT_3D ( 'NONE', #10062, #22441, #35048 ) ;
#31335=EDGE_CURVE ( 'NONE', #16497, #23691, #3503, .T. ) ;
#31341=DIRECTION ( 'NONE',  ( 1.000000000000000000, 0.000000000000000000, 0.000000000000000000 ) ) ;
#31342=EDGE_CURVE ( 'NONE', #24101, #4798, #4155, .T. ) ;
#31344=ADVANCED_FACE ( 'NONE', ( #19645 ), #38944, .F. ) ;
#31345=VECTOR ( 'NONE', #36906, 1000.000000000000000 ) ;
#31347=DIRECTION ( 'NONE',  ( 1.000000000000000000, 0.000000000000000000, 0.000000000000000000 ) ) ;
#31351=DIRECTION ( 'NONE',  ( 0.000000000000000000, 0.000000000000000000, 1.000000000000000000 ) ) ;
#31353=CIRCLE ( 'NONE', #34603, 1.000000000000000000 ) ;
#31359=ADVANCED_FACE ( 'NONE', ( #7450 ), #7854, .F. ) ;
#31370=VERTEX_POINT ( 'NONE', #1366 ) ;
#31385=EDGE_LOOP ( 'NONE', ( #19797, #30929, #39278, #13158, #7201, #32536, #18187 ) ) ;
#31390=ADVANCED_FACE ( 'NONE', ( #30903 ), #426, .F. ) ;
#31393=AXIS2_PLACEMENT_3D ( 'NONE', #6402, #34445, #3167 ) ;
#31394=CARTESIAN_POINT ( 'NONE',  ( -13.64211604268330724, 20.79918788657763429, 6.000000000000000000 ) ) ;
#31395=CARTESIAN_POINT ( 'NONE',  ( -8.917741276437942233, 30.52956727630665057, 6.000000000000000000 ) ) ;
#31400=DIRECTION ( 'NONE',  ( 0.000000000000000000, 0.000000000000000000, 1.000000000000000000 ) ) ;
#31405=ORIENTED_EDGE ( 'NONE', *, *, #26893, .F. ) ;
#31412=EDGE_CURVE ( 'NONE', #12134, #24274, #34641, .T. ) ;
#31417=EDGE_LOOP ( 'NONE', ( #22821, #16483, #27438, #3056 ) ) ;
#31418=CARTESIAN_POINT ( 'NONE',  ( 9.806975420853749625, 31.15003855377755571, 13.00000000000000178 ) ) ;
#31421=CIRCLE ( 'NONE', #26224, 1.000000000000000000 ) ;
#31431=CIRCLE ( 'NONE', #1597, 1.000000000000000000 ) ;
#31441=ADVANCED_FACE ( 'NONE', ( #33066 ), #30412, .F. ) ;
#31450=CARTESIAN_POINT ( 'NONE',  ( 3.118671991557230516, 37.17221401100731981, 13.00000000000000178 ) ) ;
#31476=AXIS2_PLACEMENT_3D ( 'NONE', #4230, #22311, #28409 ) ;
#31478=EDGE_LOOP ( 'NONE', ( #31906, #33891 ) ) ;
#31486=EDGE_CURVE ( 'NONE', #12932, #22404, #2766, .T. ) ;
#31490=CIRCLE ( 'NONE', #5528, 1.000000000000000888 ) ;
#31492=EDGE_LOOP ( 'NONE', ( #11261, #19114 ) ) ;
#31498=CYLINDRICAL_SURFACE ( 'NONE', #1927, 1.000000000000000888 ) ;
#31499=VERTEX_POINT ( 'NONE', #39340 ) ;
#31509=ADVANCED_FACE ( 'NONE', ( #11518 ), #5417, .F. ) ;
#31515=AXIS2_PLACEMENT_3D ( 'NONE', #31905, #38207, #35365 ) ;
#31523=FACE_BOUND ( 'NONE', #10185, .T. ) ;
#31545=FACE_BOUND ( 'NONE', #14230, .T. ) ;
#31563=DIRECTION ( 'NONE',  ( 0.000000000000000000, 0.000000000000000000, 1.000000000000000000 ) ) ;
#31581=CARTESIAN_POINT ( 'NONE',  ( 1.247466774197339978, 28.36888560440311480, 12.00000000000000000 ) ) ;
#31583=EDGE_CURVE ( 'NONE', #32934, #4065, #24497, .T. ) ;
#31585=CIRCLE ( 'NONE', #33590, 1.000000000000000000 ) ;
#31587=CARTESIAN_POINT ( 'NONE',  ( 8.935770203493859754, 22.34671014717335780, 12.00000000000000000 ) ) ;
#31590=EDGE_LOOP ( 'NONE', ( #37074, #14479, #24182, #23304, #11015, #4483, #38859, #35472, #32922, #4953, #24486, #10481, #9102, #2055, #22140, #36065, #29712, #14331, #28721, #5779, #35154, #18806, #24160, #7649, #7774, #900 ) ) ;
#31592=CARTESIAN_POINT ( 'NONE',  ( -1.853172919594719970, 21.57294901687549427, 13.00000000000000178 ) ) ;
#31593=AXIS2_PLACEMENT_3D ( 'NONE', #36938, #34289, #33895 ) ;
#31601=LINE ( 'NONE', #17135, #23948 ) ;
#31603=EDGE_CURVE ( 'NONE', #33412, #26968, #30132, .T. ) ;
#31605=DIRECTION ( 'NONE',  ( 1.000000000000000000, 0.000000000000000000, 0.000000000000000000 ) ) ;
#31607=VERTEX_POINT ( 'NONE', #11321 ) ;
#31624=ORIENTED_EDGE ( 'NONE', *, *, #19332, .F. ) ;
#31626=CIRCLE ( 'NONE', #7604, 1.000000000000000000 ) ;
#31641=DIRECTION ( 'NONE',  ( 0.000000000000000000, 0.000000000000000000, 1.000000000000000000 ) ) ;
#31644=ORIENTED_EDGE ( 'NONE', *, *, #23863, .T. ) ;
#31649=AXIS2_PLACEMENT_3D ( 'NONE', #25404, #21962, #9974 ) ;
#31653=CIRCLE ( 'NONE', #30995, 1.000000000000000888 ) ;
#31687=ORIENTED_EDGE ( 'NONE', *, *, #30110, .F. ) ;
#31690=AXIS2_PLACEMENT_3D ( 'NONE', #1931, #22839, #14307 ) ;
#31699=FACE_OUTER_BOUND ( 'NONE', #30598, .T. ) ;
#31703=ORIENTED_EDGE ( 'NONE', *, *, #17845, .F. ) ;
#31716=ORIENTED_EDGE ( 'NONE', *, *, #5810, .T. ) ;
#31721=FACE_BOUND ( 'NONE', #4351, .T. ) ;
#31738=EDGE_CURVE ( 'NONE', #25686, #23343, #12504, .T. ) ;
#31740=DIRECTION ( 'NONE',  ( 0.000000000000000000, 0.000000000000000000, 1.000000000000000000 ) ) ;
#31741=ADVANCED_FACE ( 'NONE', ( #13091 ), #25480, .F. ) ;
#31743=AXIS2_PLACEMENT_3D ( 'NONE', #26459, #35613, #11033 ) ;
#31745=FACE_OUTER_BOUND ( 'NONE', #7853, .T. ) ;
#31749=FACE_BOUND ( 'NONE', #31492, .T. ) ;
#31760=DIRECTION ( 'NONE',  ( 0.000000000000000000, 0.000000000000000000, 1.000000000000000000 ) ) ;
#31765=ORIENTED_EDGE ( 'NONE', *, *, #31738, .F. ) ;
#31770=VECTOR ( 'NONE', #3567, 1000.000000000000000 ) ;
#31771=ORIENTED_EDGE ( 'NONE', *, *, #14135, .F. ) ;
#31781=ORIENTED_EDGE ( 'NONE', *, *, #23412, .T. ) ;
#31793=CARTESIAN_POINT ( 'NONE',  ( 12.77090408390491305, 15.39748370681878775, 12.00000000000000000 ) ) ;
#31794=ORIENTED_EDGE ( 'NONE', *, *, #28630, .F. ) ;
#31796=DIRECTION ( 'NONE',  ( 0.000000000000000000, 0.000000000000000000, 1.000000000000000000 ) ) ;
#31799=CARTESIAN_POINT ( 'NONE',  ( -3.229437847141423124, 24.50739181907689712, 12.00000000000000000 ) ) ;
#31803=ORIENTED_EDGE ( 'NONE', *, *, #11386, .F. ) ;
#31823=DIRECTION ( 'NONE',  ( 1.000000000000000000, 0.000000000000000000, 0.000000000000000000 ) ) ;
#31835=EDGE_CURVE ( 'NONE', #11673, #17087, #6106, .T. ) ;
#31836=ORIENTED_EDGE ( 'NONE', *, *, #15348, .T. ) ;
#31841=DIRECTION ( 'NONE',  ( 0.000000000000000000, 0.000000000000000000, 1.000000000000000000 ) ) ;
#31842=ORIENTED_EDGE ( 'NONE', *, *, #7631, .F. ) ;
#31843=EDGE_CURVE ( 'NONE', #25686, #15880, #34680, .T. ) ;
#31845=AXIS2_PLACEMENT_3D ( 'NONE', #28343, #3366, #15362 ) ;
#31847=CARTESIAN_POINT ( 'NONE',  ( 6.330070799514983193, 27.28854476845134513, 12.00000000000000000 ) ) ;
#31851=CARTESIAN_POINT ( 'NONE',  ( -4.211402178667006169, 32.38366924255629442, 12.00000000000000000 ) ) ;
#31868=DIRECTION ( 'NONE',  ( 0.000000000000000000, 0.000000000000000000, 1.000000000000000000 ) ) ;
#31869=LINE ( 'NONE', #28823, #30658 ) ;
#31870=ADVANCED_FACE ( 'NONE', ( #39242 ), #16355, .F. ) ;
#31874=AXIS2_PLACEMENT_3D ( 'NONE', #38996, #7302, #7508 ) ;
#31875=DIRECTION ( 'NONE',  ( 0.000000000000000000, 0.000000000000000000, 1.000000000000000000 ) ) ;
#31876=ORIENTED_EDGE ( 'NONE', *, *, #37381, .T. ) ;
#31881=EDGE_LOOP ( 'NONE', ( #7844, #24696 ) ) ;
#31883=CYLINDRICAL_SURFACE ( 'NONE', #9247, 1.000000000000000888 ) ;
#31887=AXIS2_PLACEMENT_3D ( 'NONE', #9551, #13178, #407 ) ;
#31891=EDGE_CURVE ( 'NONE', #33301, #7705, #11973, .T. ) ;
#31894=ORIENTED_EDGE ( 'NONE', *, *, #1592, .T. ) ;
#31900=AXIS2_PLACEMENT_3D ( 'NONE', #28001, #37149, #175 ) ;
#31902=CARTESIAN_POINT ( 'NONE',  ( -0.7344975573282397363, 36.24516302788250499, 13.00000000000000178 ) ) ;
#31905=CARTESIAN_POINT ( 'NONE',  ( 14.26584437371809777, 27.13525491562438319, 13.00000000000000178 ) ) ;
#31906=ORIENTED_EDGE ( 'NONE', *, *, #14466, .F. ) ;
#31910=CIRCLE ( 'NONE', #33874, 1.000000000000000000 ) ;
#31911=DIRECTION ( 'NONE',  ( 0.000000000000000000, 0.000000000000000000, 1.000000000000000000 ) ) ;
#31913=ORIENTED_EDGE ( 'NONE', *, *, #7352, .T. ) ;
#31914=ORIENTED_EDGE ( 'NONE', *, *, #164, .F. ) ;
#31917=FACE_BOUND ( 'NONE', #31051, .T. ) ;
#31938=EDGE_CURVE ( 'NONE', #34128, #30574, #22637, .T. ) ;
#31939=AXIS2_PLACEMENT_3D ( 'NONE', #22526, #22331, #28634 ) ;
#31941=ADVANCED_FACE ( 'NONE', ( #28737 ), #1117, .F. ) ;
#31943=DIRECTION ( 'NONE',  ( 0.000000000000000000, 0.000000000000000000, 1.000000000000000000 ) ) ;
#31950=VERTEX_POINT ( 'NONE', #1317 ) ;
#31957=CARTESIAN_POINT ( 'NONE',  ( -0.6237384431625470071, 19.56555719779890978, 12.00000000000000000 ) ) ;
#31966=VECTOR ( 'NONE', #18961, 1000.000000000000000 ) ;
#31967=ORIENTED_EDGE ( 'NONE', *, *, #575, .F. ) ;
#31970=DIRECTION ( 'NONE',  ( 0.000000000000000000, 0.000000000000000000, 1.000000000000000000 ) ) ;
#31975=AXIS2_PLACEMENT_3D ( 'NONE', #10225, #35018, #6764 ) ;
#31981=ORIENTED_EDGE ( 'NONE', *, *, #23042, .F. ) ;
#31993=DIRECTION ( 'NONE',  ( 1.000000000000000000, 0.000000000000000000, 0.000000000000000000 ) ) ;
#31994=DIRECTION ( 'NONE',  ( 0.000000000000000000, 0.000000000000000000, 1.000000000000000000 ) ) ;
#31998=CARTESIAN_POINT ( 'NONE',  ( 5.440829913680675034, 10.60893893836775348, 6.000000000000000000 ) ) ;
#32000=DIRECTION ( 'NONE',  ( 0.000000000000000000, 0.000000000000000000, 1.000000000000000000 ) ) ;
#32001=LINE ( 'NONE', #19206, #35909 ) ;
#32004=VERTEX_POINT ( 'NONE', #24606 ) ;
#32005=AXIS2_PLACEMENT_3D ( 'NONE', #5374, #36061, #4775 ) ;
#32017=CIRCLE ( 'NONE', #2818, 1.000000000000000888 ) ;
#32027=DIRECTION ( 'NONE',  ( 1.000000000000000000, 0.000000000000000000, 0.000000000000000000 ) ) ;
#32032=ORIENTED_EDGE ( 'NONE', *, *, #30493, .T. ) ;
#32038=ADVANCED_FACE ( 'NONE', ( #36796 ), #36599, .F. ) ;
#32047=CARTESIAN_POINT ( 'NONE',  ( 0.9999966292907466192, 22.50000000000031264, 13.00000000000000178 ) ) ;
#32048=DIRECTION ( 'NONE',  ( 1.000000000000000000, 0.000000000000000000, 0.000000000000000000 ) ) ;
#32056=DIRECTION ( 'NONE',  ( 0.000000000000000000, 0.000000000000000000, 1.000000000000000000 ) ) ;
#32060=DIRECTION ( 'NONE',  ( 1.000000000000000000, 0.000000000000000000, 0.000000000000000000 ) ) ;
#32063=DIRECTION ( 'NONE',  ( 0.000000000000000000, 0.000000000000000000, 1.000000000000000000 ) ) ;
#32069=EDGE_CURVE ( 'NONE', #4829, #33109, #26903, .T. ) ;
#32070=DIRECTION ( 'NONE',  ( 0.000000000000000000, 0.000000000000000000, 1.000000000000000000 ) ) ;
#32072=ORIENTED_EDGE ( 'NONE', *, *, #2203, .F. ) ;
#32076=CARTESIAN_POINT ( 'NONE',  ( -9.183247089818959097, 16.78440424842446532, 13.00000000000000178 ) ) ;
#32088=CIRCLE ( 'NONE', #21072, 1.000000000000000000 ) ;
#32093=VECTOR ( 'NONE', #18822, 1000.000000000000000 ) ;
#32098=ORIENTED_EDGE ( 'NONE', *, *, #9085, .T. ) ;
#32106=DIRECTION ( 'NONE',  ( 0.000000000000000000, 0.000000000000000000, 1.000000000000000000 ) ) ;
#32113=EDGE_LOOP ( 'NONE', ( #11246, #12825 ) ) ;
#32118=CARTESIAN_POINT ( 'NONE',  ( -1.494943660522439099, 10.76222879119470832, 12.00000000000000000 ) ) ;
#32119=ORIENTED_EDGE ( 'NONE', *, *, #21941, .T. ) ;
#32120=ORIENTED_EDGE ( 'NONE', *, *, #20795, .T. ) ;
#32127=VECTOR ( 'NONE', #11695, 1000.000000000000000 ) ;
#32128=CARTESIAN_POINT ( 'NONE',  ( 13.64210930126480115, 24.20081211342298744, 12.00000000000000000 ) ) ;
#32133=CYLINDRICAL_SURFACE ( 'NONE', #40085, 1.000000000000000000 ) ;
#32142=ORIENTED_EDGE ( 'NONE', *, *, #21458, .F. ) ;
#32151=EDGE_CURVE ( 'NONE', #38676, #39628, #317, .T. ) ;
#32152=CIRCLE ( 'NONE', #9453, 1.000000000000000000 ) ;
#32155=FACE_BOUND ( 'NONE', #26984, .T. ) ;
#32165=DIRECTION ( 'NONE',  ( 0.000000000000000000, 0.000000000000000000, 1.000000000000000000 ) ) ;
#32167=ORIENTED_EDGE ( 'NONE', *, *, #19192, .F. ) ;
#32169=CYLINDRICAL_SURFACE ( 'NONE', #31975, 1.000000000000000888 ) ;
#32176=VERTEX_POINT ( 'NONE', #15059 ) ;
#32185=VECTOR ( 'NONE', #32165, 1000.000000000000000 ) ;
#32201=DIRECTION ( 'NONE',  ( 1.000000000000000000, 0.000000000000000000, 0.000000000000000000 ) ) ;
#32203=CYLINDRICAL_SURFACE ( 'NONE', #31332, 1.000000000000000000 ) ;
#32215=DIRECTION ( 'NONE',  ( 0.000000000000000000, 0.000000000000000000, 1.000000000000000000 ) ) ;
#32228=EDGE_LOOP ( 'NONE', ( #4401, #8384, #25852, #9728 ) ) ;
#32245=AXIS2_PLACEMENT_3D ( 'NONE', #5888, #34131, #4 ) ;
#32250=EDGE_CURVE ( 'NONE', #36138, #5201, #10974, .T. ) ;
#32251=EDGE_CURVE ( 'NONE', #30326, #12836, #33422, .T. ) ;
#32253=ORIENTED_EDGE ( 'NONE', *, *, #33979, .T. ) ;
#32259=CARTESIAN_POINT ( 'NONE',  ( 4.724371395536106633, 32.23037938972932892, 12.00000000000000000 ) ) ;
#32261=DIRECTION ( 'NONE',  ( -1.000000000000000000, 0.000000000000000000, 0.000000000000000000 ) ) ;
#32270=DIRECTION ( 'NONE',  ( 1.000000000000000000, 0.000000000000000000, 0.000000000000000000 ) ) ;
#32272=AXIS2_PLACEMENT_3D ( 'NONE', #24833, #9198, #9798 ) ;
#32280=CARTESIAN_POINT ( 'NONE',  ( 11.77090408390491305, 15.39748370681878775, 6.000000000000000000 ) ) ;
#32281=VERTEX_POINT ( 'NONE', #39196 ) ;
#32283=AXIS2_PLACEMENT_3D ( 'NONE', #30801, #2762, #6399 ) ;
#32286=CIRCLE ( 'NONE', #25108, 1.000000000000000888 ) ;
#32288=EDGE_LOOP ( 'NONE', ( #35035, #3285 ) ) ;
#32294=ORIENTED_EDGE ( 'NONE', *, *, #12942, .F. ) ;
#32299=DIRECTION ( 'NONE',  ( 0.000000000000000000, 0.000000000000000000, 1.000000000000000000 ) ) ;
#32303=AXIS2_PLACEMENT_3D ( 'NONE', #25082, #304, #15940 ) ;
#32308=CARTESIAN_POINT ( 'NONE',  ( 3.835130509701798918, 15.55077355964573904, 13.00000000000000178 ) ) ;
#32309=EDGE_CURVE ( 'NONE', #36348, #12651, #32914, .T. ) ;
#32317=DIRECTION ( 'NONE',  ( 0.000000000000000000, 0.000000000000000000, 1.000000000000000000 ) ) ;
#32320=DIRECTION ( 'NONE',  ( 0.000000000000000000, 0.000000000000000000, 1.000000000000000000 ) ) ;
#32330=CARTESIAN_POINT ( 'NONE',  ( 4.082600654608392610, 21.41965916404854298, 6.000000000000000000 ) ) ;
#32334=DIRECTION ( 'NONE',  ( 1.000000000000000000, 0.000000000000000000, 0.000000000000000000 ) ) ;
#32338=DIRECTION ( 'NONE',  ( 0.000000000000000000, 0.000000000000000000, 1.000000000000000000 ) ) ;
#32355=CARTESIAN_POINT ( 'NONE',  ( -2.494943660522439099, 10.76222879119470832, 6.000000000000000000 ) ) ;
#32360=VECTOR ( 'NONE', #29214, 1000.000000000000000 ) ;
#32362=CIRCLE ( 'NONE', #10964, 16.99999999999999645 ) ;
#32363=EDGE_CURVE ( 'NONE', #17409, #6680, #2034, .T. ) ;
#32366=EDGE_CURVE ( 'NONE', #2590, #15085, #1423, .T. ) ;
#32368=CIRCLE ( 'NONE', #14850, 1.000000000000000888 ) ;
#32369=CARTESIAN_POINT ( 'NONE',  ( -12.39464589777671044, 26.66807349098043289, 13.00000000000000178 ) ) ;
#32379=EDGE_LOOP ( 'NONE', ( #33502, #13942 ) ) ;
#32392=CARTESIAN_POINT ( 'NONE',  ( -9.806982162272253944, 13.84996144622306247, 13.00000000000000178 ) ) ;
#32396=VERTEX_POINT ( 'NONE', #35353 ) ;
#32398=AXIS2_PLACEMENT_3D ( 'NONE', #8979, #17537, #5924 ) ;
#32402=ORIENTED_EDGE ( 'NONE', *, *, #28126, .F. ) ;
#32404=CIRCLE ( 'NONE', #14876, 1.000000000000000000 ) ;
#32408=EDGE_CURVE ( 'NONE', #4328, #37515, #31431, .T. ) ;
#32413=CARTESIAN_POINT ( 'NONE',  ( -12.41268156625113406, 18.79179606750104981, 13.00000000000000178 ) ) ;
#32432=DIRECTION ( 'NONE',  ( 1.000000000000000000, 0.000000000000000000, 0.000000000000000000 ) ) ;
#32438=ORIENTED_EDGE ( 'NONE', *, *, #19953, .T. ) ;
#32447=EDGE_LOOP ( 'NONE', ( #23763, #27243, #28437, #9631 ) ) ;
#32455=AXIS2_PLACEMENT_3D ( 'NONE', #11521, #20869, #5422 ) ;
#32456=CARTESIAN_POINT ( 'NONE',  ( -2.871208588069141143, 13.69667159339610762, 6.000000000000000000 ) ) ;
#32460=DIRECTION ( 'NONE',  ( 0.000000000000000000, 0.000000000000000000, 1.000000000000000000 ) ) ;
#32462=EDGE_CURVE ( 'NONE', #39039, #888, #24301, .T. ) ;
#32468=CARTESIAN_POINT ( 'NONE',  ( 0.6237317017440463518, 25.43444280220171194, 13.00000000000000178 ) ) ;
#32469=DIRECTION ( 'NONE',  ( 0.000000000000000000, 0.000000000000000000, 1.000000000000000000 ) ) ;
#32473=CIRCLE ( 'NONE', #15667, 1.000000000000000888 ) ;
#32477=DIRECTION ( 'NONE',  ( 0.000000000000000000, 0.000000000000000000, 1.000000000000000000 ) ) ;
#32482=CARTESIAN_POINT ( 'NONE',  ( 0.2655024426717602637, 36.24516302788250499, 6.000000000000000000 ) ) ;
#32489=ORIENTED_EDGE ( 'NONE', *, *, #18379, .T. ) ;
#32493=VERTEX_POINT ( 'NONE', #30662 ) ;
#32494=EDGE_CURVE ( 'NONE', #6257, #30063, #4863, .T. ) ;
#32505=VERTEX_POINT ( 'NONE', #11572 ) ;
#32524=DIRECTION ( 'NONE',  ( 1.000000000000000000, 0.000000000000000000, 0.000000000000000000 ) ) ;
#32525=DIRECTION ( 'NONE',  ( 1.000000000000000000, 0.000000000000000000, 0.000000000000000000 ) ) ;
#32527=DIRECTION ( 'NONE',  ( 0.000000000000000000, 0.000000000000000000, 1.000000000000000000 ) ) ;
#32535=DIRECTION ( 'NONE',  ( 0.000000000000000000, 0.000000000000000000, 1.000000000000000000 ) ) ;
#32536=ORIENTED_EDGE ( 'NONE', *, *, #2965, .T. ) ;
#32537=ORIENTED_EDGE ( 'NONE', *, *, #9642, .T. ) ;
#32540=FACE_BOUND ( 'NONE', #9975, .T. ) ;
#32551=VERTEX_POINT ( 'NONE', #11768 ) ;
#32554=VERTEX_POINT ( 'NONE', #24154 ) ;
#32586=ORIENTED_EDGE ( 'NONE', *, *, #35900, .F. ) ;
#32595=CARTESIAN_POINT ( 'NONE',  ( 7.935770203493858865, 22.34671014717335780, 13.00000000000000178 ) ) ;
#32602=AXIS2_PLACEMENT_3D ( 'NONE', #18209, #14954, #11510 ) ;
#32606=DIRECTION ( 'NONE',  ( 0.000000000000000000, 0.000000000000000000, 1.000000000000000000 ) ) ;
#32611=AXIS2_PLACEMENT_3D ( 'NONE', #12665, #81, #9027 ) ;
#32613=ORIENTED_EDGE ( 'NONE', *, *, #164, .T. ) ;
#32650=ADVANCED_FACE ( 'NONE', ( #36550 ), #21113, .F. ) ;
#32653=FACE_OUTER_BOUND ( 'NONE', #39855, .T. ) ;
#32660=FACE_OUTER_BOUND ( 'NONE', #27460, .T. ) ;
#32663=CARTESIAN_POINT ( 'NONE',  ( -13.01838097023000707, 23.73363068877903359, 13.00000000000000178 ) ) ;
#32666=ADVANCED_FACE ( 'NONE', ( #25745 ), #28395, .F. ) ;
#32672=FACE_OUTER_BOUND ( 'NONE', #4396, .T. ) ;
#32678=CARTESIAN_POINT ( 'NONE',  ( 8.312035131040566682, 19.41226734497195849, 6.000000000000000000 ) ) ;
#32692=ORIENTED_EDGE ( 'NONE', *, *, #19550, .T. ) ;
#32696=ORIENTED_EDGE ( 'NONE', *, *, #14570, .T. ) ;
#32699=ORIENTED_EDGE ( 'NONE', *, *, #37592, .T. ) ;
#32701=ORIENTED_EDGE ( 'NONE', *, *, #8091, .F. ) ;
#32704=VERTEX_POINT ( 'NONE', #9722 ) ;
#32708=DIRECTION ( 'NONE',  ( 1.000000000000000000, 0.000000000000000000, 0.000000000000000000 ) ) ;
#32709=DIRECTION ( 'NONE',  ( 0.000000000000000000, 0.000000000000000000, 1.000000000000000000 ) ) ;
#32711=AXIS2_PLACEMENT_3D ( 'NONE', #33960, #3276, #12222 ) ;
#32723=DIRECTION ( 'NONE',  ( 1.000000000000000000, 0.000000000000000000, 0.000000000000000000 ) ) ;
#32731=CARTESIAN_POINT ( 'NONE',  ( 8.312035131040566682, 19.41226734497195849, 13.00000000000000178 ) ) ;
#32735=DIRECTION ( 'NONE',  ( 0.000000000000000000, 0.000000000000000000, 1.000000000000000000 ) ) ;
#32737=FACE_BOUND ( 'NONE', #12480, .T. ) ;
#32740=DIRECTION ( 'NONE',  ( 0.000000000000000000, 0.000000000000000000, 1.000000000000000000 ) ) ;
#32747=ORIENTED_EDGE ( 'NONE', *, *, #15720, .F. ) ;
#32755=ORIENTED_EDGE ( 'NONE', *, *, #37592, .F. ) ;
#32758=DIRECTION ( 'NONE',  ( 1.000000000000000000, 0.000000000000000000, 0.000000000000000000 ) ) ;
#32764=EDGE_CURVE ( 'NONE', #9924, #22293, #18505, .T. ) ;
#32767=FACE_OUTER_BOUND ( 'NONE', #3302, .T. ) ;
#32777=AXIS2_PLACEMENT_3D ( 'NONE', #22492, #31252, #3813 ) ;
#32780=DIRECTION ( 'NONE',  ( 0.000000000000000000, 0.000000000000000000, 1.000000000000000000 ) ) ;
#32786=DIRECTION ( 'NONE',  ( 1.000000000000000000, 0.000000000000000000, 0.000000000000000000 ) ) ;
#32802=CIRCLE ( 'NONE', #31476, 1.000000000000000000 ) ;
#32807=CIRCLE ( 'NONE', #20474, 1.000000000000000888 ) ;
#32809=DIRECTION ( 'NONE',  ( 1.000000000000000000, 0.000000000000000000, 0.000000000000000000 ) ) ;
#32811=CIRCLE ( 'NONE', #8785, 1.000000000000000000 ) ;
#32812=DIRECTION ( 'NONE',  ( 0.000000000000000000, 0.000000000000000000, 1.000000000000000000 ) ) ;
#32822=DIRECTION ( 'NONE',  ( 0.000000000000000000, 0.000000000000000000, 1.000000000000000000 ) ) ;
#32825=PRESENTATION_STYLE_ASSIGNMENT (( #22852 ) ) ;
#32830=CARTESIAN_POINT ( 'NONE',  ( 6.330070799514983193, 27.28854476845134513, 12.00000000000000000 ) ) ;
#32832=VERTEX_POINT ( 'NONE', #974 ) ;
#32833=CARTESIAN_POINT ( 'NONE',  ( -7.953812613386786801, 14.77701242934787906, 12.00000000000000000 ) ) ;
#32834=ORIENTED_EDGE ( 'NONE', *, *, #25728, .T. ) ;
#32835=VECTOR ( 'NONE', #22402, 1000.000000000000000 ) ;
#32840=AXIS2_PLACEMENT_3D ( 'NONE', #14169, #1180, #13563 ) ;
#32860=CARTESIAN_POINT ( 'NONE',  ( -7.577547685840081648, 11.84256962714647798, 13.00000000000000178 ) ) ;
#32862=CARTESIAN_POINT ( 'NONE',  ( 2.871201846650637268, 31.30332840660451765, 12.00000000000000000 ) ) ;
#32865=DIRECTION ( 'NONE',  ( 0.000000000000000000, 0.000000000000000000, 1.000000000000000000 ) ) ;
#32866=AXIS2_PLACEMENT_3D ( 'NONE', #21231, #12086, #34028 ) ;
#32871=CARTESIAN_POINT ( 'NONE',  ( 6.082600654608392610, 21.41965916404854298, 13.00000000000000178 ) ) ;
#32878=EDGE_CURVE ( 'NONE', #2749, #3856, #37320, .T. ) ;
#32881=EDGE_CURVE ( 'NONE', #28480, #3881, #38591, .T. ) ;
#32890=DIRECTION ( 'NONE',  ( 0.000000000000000000, 0.000000000000000000, 1.000000000000000000 ) ) ;
#32891=EDGE_LOOP ( 'NONE', ( #30705, #9906, #29921, #25323 ) ) ;
#32899=DIRECTION ( 'NONE',  ( 0.000000000000000000, 0.000000000000000000, -1.000000000000000000 ) ) ;
#32905=ORIENTED_EDGE ( 'NONE', *, *, #20961, .T. ) ;
#32907=EDGE_LOOP ( 'NONE', ( #21733, #23060 ) ) ;
#32909=VERTEX_POINT ( 'NONE', #32047 ) ;
#32913=VERTEX_POINT ( 'NONE', #38545 ) ;
#32914=LINE ( 'NONE', #26603, #7440 ) ;
#32921=AXIS2_PLACEMENT_3D ( 'NONE', #28176, #3789, #40168 ) ;
#32922=ORIENTED_EDGE ( 'NONE', *, *, #3758, .F. ) ;
#32929=AXIS2_PLACEMENT_3D ( 'NONE', #27358, #11527, #8677 ) ;
#32933=LINE ( 'NONE', #16891, #4957 ) ;
#32934=VERTEX_POINT ( 'NONE', #10928 ) ;
#32941=ORIENTED_EDGE ( 'NONE', *, *, #11789, .F. ) ;
#32944=DIRECTION ( 'NONE',  ( 1.000000000000000000, 0.000000000000000000, 0.000000000000000000 ) ) ;
#32949=CARTESIAN_POINT ( 'NONE',  ( 3.211395437248501850, 12.61633075744433796, 13.00000000000000178 ) ) ;
#32951=ADVANCED_FACE ( 'NONE', ( #4822 ), #17431, .F. ) ;
#32964=EDGE_LOOP ( 'NONE', ( #9800, #20976, #26392, #17273, #8794, #34366 ) ) ;
#32965=DIRECTION ( 'NONE',  ( 1.000000000000000000, 0.000000000000000000, 0.000000000000000000 ) ) ;
#32966=CARTESIAN_POINT ( 'NONE',  ( -11.39464589777670867, 26.66807349098043289, 6.000000000000000000 ) ) ;
#32970=ADVANCED_FACE ( 'NONE', ( #13961 ), #16619, .F. ) ;
#32987=VERTEX_POINT ( 'NONE', #14368 ) ;
#32995=AXIS2_PLACEMENT_3D ( 'NONE', #17053, #25576, #29235 ) ;
#33000=EDGE_LOOP ( 'NONE', ( #4126, #30621 ) ) ;
#33003=CYLINDRICAL_SURFACE ( 'NONE', #19296, 1.000000000000000000 ) ;
#33004=EDGE_CURVE ( 'NONE', #18451, #32281, #6790, .T. ) ;
#33014=DIRECTION ( 'NONE',  ( 1.000000000000000000, 0.000000000000000000, 0.000000000000000000 ) ) ;
#33015=CIRCLE ( 'NONE', #9661, 16.99999999999999645 ) ;
#33019=AXIS2_PLACEMENT_3D ( 'NONE', #15792, #27983, #9103 ) ;
#33023=LINE ( 'NONE', #27106, #11424 ) ;
#33024=ORIENTED_EDGE ( 'NONE', *, *, #7352, .F. ) ;
#33026=CARTESIAN_POINT ( 'NONE',  ( 8.917734535019441466, 14.47043272369397116, 13.00000000000000178 ) ) ;
#33033=EDGE_LOOP ( 'NONE', ( #36375, #13002, #40181, #30049 ) ) ;
#33036=LINE ( 'NONE', #5185, #39285 ) ;
#33038=VERTEX_POINT ( 'NONE', #39741 ) ;
#33057=ORIENTED_EDGE ( 'NONE', *, *, #25674, .F. ) ;
#33063=CARTESIAN_POINT ( 'NONE',  ( 0.3762615568374529929, 19.56555719779890978, 13.00000000000000178 ) ) ;
#33066=FACE_OUTER_BOUND ( 'NONE', #17485, .T. ) ;
#33067=AXIS2_PLACEMENT_3D ( 'NONE', #21019, #17787, #11278 ) ;
#33073=CARTESIAN_POINT ( 'NONE',  ( 5.082600654608392610, 21.41965916404854298, 12.00000000000000000 ) ) ;
#33088=DIRECTION ( 'NONE',  ( 0.000000000000000000, 0.000000000000000000, 1.000000000000000000 ) ) ;
#33097=VECTOR ( 'NONE', #78, 1000.000000000000000 ) ;
#33099=ORIENTED_EDGE ( 'NONE', *, *, #27945, .F. ) ;
#33109=VERTEX_POINT ( 'NONE', #17831 ) ;
#33113=DIRECTION ( 'NONE',  ( 1.000000000000000000, 0.000000000000000000, 0.000000000000000000 ) ) ;
#33116=ORIENTED_EDGE ( 'NONE', *, *, #1577, .T. ) ;
#33118=CARTESIAN_POINT ( 'NONE',  ( -7.064571727552472424, 31.45661825943146894, 13.00000000000000178 ) ) ;
#33129=CARTESIAN_POINT ( 'NONE',  ( -7.917741276437941345, 30.52956727630665057, 12.00000000000000000 ) ) ;
#33140=DIRECTION ( 'NONE',  ( 1.000000000000000000, 0.000000000000000000, 0.000000000000000000 ) ) ;
#33141=AXIS2_PLACEMENT_3D ( 'NONE', #4413, #28591, #35704 ) ;
#33143=ORIENTED_EDGE ( 'NONE', *, *, #40040, .T. ) ;
#33145=AXIS2_PLACEMENT_3D ( 'NONE', #17636, #23909, #8473 ) ;
#33149=ORIENTED_EDGE ( 'NONE', *, *, #21707, .F. ) ;
#33162=CARTESIAN_POINT ( 'NONE',  ( 3.118671991557230516, 37.17221401100731981, 6.000000000000000000 ) ) ;
#33164=DIRECTION ( 'NONE',  ( 1.000000000000000000, 0.000000000000000000, 0.000000000000000000 ) ) ;
#33165=ORIENTED_EDGE ( 'NONE', *, *, #12109, .T. ) ;
#33166=DIRECTION ( 'NONE',  ( 1.000000000000000000, 0.000000000000000000, 0.000000000000000000 ) ) ;
#33167=DIRECTION ( 'NONE',  ( 1.000000000000000000, 0.000000000000000000, 0.000000000000000000 ) ) ;
#33177=DIRECTION ( 'NONE',  ( 0.000000000000000000, 0.000000000000000000, 1.000000000000000000 ) ) ;
#33185=VERTEX_POINT ( 'NONE', #36109 ) ;
#33190=CYLINDRICAL_SURFACE ( 'NONE', #40003, 1.000000000000000000 ) ;
#33193=ORIENTED_EDGE ( 'NONE', *, *, #13339, .F. ) ;
#33197=ORIENTED_EDGE ( 'NONE', *, *, #23609, .T. ) ;
#33199=DIRECTION ( 'NONE',  ( 0.000000000000000000, 0.000000000000000000, 1.000000000000000000 ) ) ;
#33200=CARTESIAN_POINT ( 'NONE',  ( 1.605696033269625955, 17.55816537872232530, 6.000000000000000000 ) ) ;
#33210=EDGE_LOOP ( 'NONE', ( #7943, #22159, #39020, #31166 ) ) ;
#33218=DIRECTION ( 'NONE',  ( 1.000000000000000000, 0.000000000000000000, 0.000000000000000000 ) ) ;
#33220=DIRECTION ( 'NONE',  ( -0.000000000000000000, -0.000000000000000000, -1.000000000000000000 ) ) ;
#33223=DIRECTION ( 'NONE',  ( 1.000000000000000000, 0.000000000000000000, 0.000000000000000000 ) ) ;
#33226=EDGE_CURVE ( 'NONE', #17512, #25213, #1014, .T. ) ;
#33228=CARTESIAN_POINT ( 'NONE',  ( -9.806982162272253944, 13.84996144622306247, 12.00000000000000000 ) ) ;
#33238=ORIENTED_EDGE ( 'NONE', *, *, #2203, .T. ) ;
#33259=CIRCLE ( 'NONE', #20910, 1.000000000000000000 ) ;
#33261=EDGE_CURVE ( 'NONE', #39628, #38676, #2325, .T. ) ;
#33269=DIRECTION ( 'NONE',  ( 1.000000000000000000, 0.000000000000000000, 0.000000000000000000 ) ) ;
#33274=AXIS2_PLACEMENT_3D ( 'NONE', #32949, #23791, #5107 ) ;
#33279=EDGE_CURVE ( 'NONE', #20514, #32554, #5559, .T. ) ;
#33283=CIRCLE ( 'NONE', #833, 1.000000000000000000 ) ;
#33296=CARTESIAN_POINT ( 'NONE',  ( 9.165204679926031162, 20.33931832809677331, 13.00000000000000178 ) ) ;
#33298=VERTEX_POINT ( 'NONE', #34845 ) ;
#33301=VERTEX_POINT ( 'NONE', #31793 ) ;
#33311=CARTESIAN_POINT ( 'NONE',  ( 8.541469607472738090, 17.40487552589537401, 13.00000000000000178 ) ) ;
#33315=AXIS2_PLACEMENT_3D ( 'NONE', #14969, #21070, #8678 ) ;
#33318=CIRCLE ( 'NONE', #15782, 1.000000000000000888 ) ;
#33321=CARTESIAN_POINT ( 'NONE',  ( 2.247466774197339756, 28.36888560440311480, 12.00000000000000000 ) ) ;
#33323=CIRCLE ( 'NONE', #24859, 1.000000000000000888 ) ;
#33325=EDGE_LOOP ( 'NONE', ( #6305, #37540, #24003, #12443 ) ) ;
#33328=CARTESIAN_POINT ( 'NONE',  ( 5.100636323082810009, 29.29593658752792962, 13.00000000000000178 ) ) ;
#33348=VERTEX_POINT ( 'NONE', #18814 ) ;
#33367=ORIENTED_EDGE ( 'NONE', *, *, #22787, .F. ) ;
#33369=FACE_OUTER_BOUND ( 'NONE', #22490, .T. ) ;
#33371=DIRECTION ( 'NONE',  ( 0.000000000000000000, 0.000000000000000000, 1.000000000000000000 ) ) ;
#33374=EDGE_CURVE ( 'NONE', #23691, #17784, #719, .T. ) ;
#33397=ORIENTED_EDGE ( 'NONE', *, *, #15348, .F. ) ;
#33404=DIRECTION ( 'NONE',  ( 1.000000000000000000, 0.000000000000000000, 0.000000000000000000 ) ) ;
#33405=DIRECTION ( 'NONE',  ( 1.000000000000000000, 0.000000000000000000, 0.000000000000000000 ) ) ;
#33408=VERTEX_POINT ( 'NONE', #3365 ) ;
#33412=VERTEX_POINT ( 'NONE', #3563 ) ;
#33417=AXIS2_PLACEMENT_3D ( 'NONE', #35967, #32527, #30070 ) ;
#33418=CARTESIAN_POINT ( 'NONE',  ( -6.577547685840081648, 11.84256962714647798, 12.00000000000000000 ) ) ;
#33422=CIRCLE ( 'NONE', #6133, 1.000000000000000000 ) ;
#33423=FACE_BOUND ( 'NONE', #35502, .T. ) ;
#33424=DIRECTION ( 'NONE',  ( 1.000000000000000000, 0.000000000000000000, 0.000000000000000000 ) ) ;
#33425=VERTEX_POINT ( 'NONE', #15961 ) ;
#33427=CARTESIAN_POINT ( 'NONE',  ( -4.100643064501314328, 15.70406341247269211, 6.000000000000000000 ) ) ;
#33434=EDGE_LOOP ( 'NONE', ( #37339, #21736 ) ) ;
#33443=CARTESIAN_POINT ( 'NONE',  ( 14.64210930126480115, 24.20081211342298744, 13.00000000000000178 ) ) ;
#33453=CARTESIAN_POINT ( 'NONE',  ( -1.605702774688126722, 27.44183462127829642, 12.00000000000000000 ) ) ;
#33456=CIRCLE ( 'NONE', #13964, 1.000000000000000888 ) ;
#33457=EDGE_LOOP ( 'NONE', ( #14292, #16803, #19285, #26942 ) ) ;
#33465=EDGE_CURVE ( 'NONE', #31607, #19767, #3958, .T. ) ;
#33467=ORIENTED_EDGE ( 'NONE', *, *, #26045, .F. ) ;
#33470=CARTESIAN_POINT ( 'NONE',  ( -3.118678732975735279, 7.827785988993307242, 6.000000000000000000 ) ) ;
#33494=ADVANCED_FACE ( 'NONE', ( #19809 ), #23051, .F. ) ;
#33502=ORIENTED_EDGE ( 'NONE', *, *, #21667, .F. ) ;
#33505=CARTESIAN_POINT ( 'NONE',  ( 0.9819609608163288872, 14.62372257652092422, 13.00000000000000178 ) ) ;
#33508=ADVANCED_FACE ( 'NONE', ( #35654 ), #20419, .F. ) ;
#33513=ORIENTED_EDGE ( 'NONE', *, *, #21557, .F. ) ;
#33520=CARTESIAN_POINT ( 'NONE',  ( 9.541469607472739867, 17.40487552589537401, 6.000000000000000000 ) ) ;
#33531=ADVANCED_FACE ( 'NONE', ( #38290 ), #20014, .F. ) ;
#33533=DIRECTION ( 'NONE',  ( 1.000000000000000000, 0.000000000000000000, 0.000000000000000000 ) ) ;
#33539=CARTESIAN_POINT ( 'NONE',  ( -7.953812613386786801, 14.77701242934787906, 6.000000000000000000 ) ) ;
#33541=ORIENTED_EDGE ( 'NONE', *, *, #466, .F. ) ;
#33543=DIRECTION ( 'NONE',  ( 0.000000000000000000, 0.000000000000000000, 1.000000000000000000 ) ) ;
#33544=DIRECTION ( 'NONE',  ( 0.000000000000000000, 0.000000000000000000, 1.000000000000000000 ) ) ;
#33546=VERTEX_POINT ( 'NONE', #10668 ) ;
#33548=CARTESIAN_POINT ( 'NONE',  ( -1.265509184090266137, 8.754836972118123839, 13.00000000000000178 ) ) ;
#33556=ORIENTED_EDGE ( 'NONE', *, *, #28126, .T. ) ;
#33564=EDGE_LOOP ( 'NONE', ( #18673, #30352, #564, #14405 ) ) ;
#33566=CYLINDRICAL_SURFACE ( 'NONE', #2676, 1.000000000000000000 ) ;
#33588=DIRECTION ( 'NONE',  ( 1.000000000000000000, 0.000000000000000000, 0.000000000000000000 ) ) ;
#33589=VECTOR ( 'NONE', #23442, 1000.000000000000000 ) ;
#33590=AXIS2_PLACEMENT_3D ( 'NONE', #26983, #14795, #23935 ) ;
#33597=DIRECTION ( 'NONE',  ( 1.000000000000000000, 0.000000000000000000, 0.000000000000000000 ) ) ;
#33598=CYLINDRICAL_SURFACE ( 'NONE', #13439, 1.000000000000000000 ) ;
#33600=EDGE_LOOP ( 'NONE', ( #1741, #36520 ) ) ;
#33602=VERTEX_POINT ( 'NONE', #8011 ) ;
#33617=CIRCLE ( 'NONE', #25795, 1.000000000000000000 ) ;
#33618=FACE_BOUND ( 'NONE', #40173, .T. ) ;
#33622=DIRECTION ( 'NONE',  ( 1.000000000000000000, 0.000000000000000000, 0.000000000000000000 ) ) ;
#33623=DIRECTION ( 'NONE',  ( 1.000000000000000000, 0.000000000000000000, 0.000000000000000000 ) ) ;
#33625=CIRCLE ( 'NONE', #39434, 1.000000000000000000 ) ;
#33630=EDGE_LOOP ( 'NONE', ( #15897, #28762, #23676, #35122 ) ) ;
#33639=EDGE_LOOP ( 'NONE', ( #10766, #17568, #11435, #24867 ) ) ;
#33643=CYLINDRICAL_SURFACE ( 'NONE', #32866, 1.000000000000000000 ) ;
#33648=VERTEX_POINT ( 'NONE', #35451 ) ;
#33650=CARTESIAN_POINT ( 'NONE',  ( 1.871201846650637046, 31.30332840660451765, 13.00000000000000178 ) ) ;
#33664=VERTEX_POINT ( 'NONE', #16563 ) ;
#33672=DIRECTION ( 'NONE',  ( 0.000000000000000000, 0.000000000000000000, 1.000000000000000000 ) ) ;
#33678=AXIS2_PLACEMENT_3D ( 'NONE', #9991, #9797, #22177 ) ;
#33689=ORIENTED_EDGE ( 'NONE', *, *, #8064, .T. ) ;
#33696=DIRECTION ( 'NONE',  ( 0.000000000000000000, 0.000000000000000000, 1.000000000000000000 ) ) ;
#33698=ORIENTED_EDGE ( 'NONE', *, *, #8552, .T. ) ;
#33707=CIRCLE ( 'NONE', #2552, 1.000000000000000000 ) ;
#33708=AXIS2_PLACEMENT_3D ( 'NONE', #35719, #26971, #29613 ) ;
#33713=ORIENTED_EDGE ( 'NONE', *, *, #8091, .T. ) ;
#33714=AXIS2_PLACEMENT_3D ( 'NONE', #11620, #11813, #8562 ) ;
#33715=DIRECTION ( 'NONE',  ( 0.000000000000000000, 0.000000000000000000, 1.000000000000000000 ) ) ;
#33719=ORIENTED_EDGE ( 'NONE', *, *, #24021, .T. ) ;
#33727=ORIENTED_EDGE ( 'NONE', *, *, #22054, .F. ) ;
#33732=ADVANCED_FACE ( 'NONE', ( #14312 ), #36654, .F. ) ;
#33735=EDGE_CURVE ( 'NONE', #19392, #20347, #17382, .T. ) ;
#33743=CIRCLE ( 'NONE', #36974, 1.000000000000000888 ) ;
#33745=CARTESIAN_POINT ( 'NONE',  ( -13.64211604268330724, 20.79918788657763429, 13.00000000000000178 ) ) ;
#33746=DIRECTION ( 'NONE',  ( 0.000000000000000000, 0.000000000000000000, 1.000000000000000000 ) ) ;
#33748=ORIENTED_EDGE ( 'NONE', *, *, #12866, .T. ) ;
#33756=ORIENTED_EDGE ( 'NONE', *, *, #31121, .T. ) ;
#33765=DIRECTION ( 'NONE',  ( 1.000000000000000000, 0.000000000000000000, 0.000000000000000000 ) ) ;
#33776=ORIENTED_EDGE ( 'NONE', *, *, #38040, .F. ) ;
#33787=SHAPE_REPRESENTATION ( 'Protective Beveled Outer Blade Guard', ( #24238 ), #27483 ) ;
#33800=VERTEX_POINT ( 'NONE', #11868 ) ;
#33802=CARTESIAN_POINT ( 'NONE',  ( -1.247473515615844075, 16.63111439559750693, 6.000000000000000000 ) ) ;
#33804=EDGE_LOOP ( 'NONE', ( #37327, #34391 ) ) ;
#33807=CARTESIAN_POINT ( 'NONE',  ( 1.247466774197339978, 28.36888560440311480, 6.000000000000000000 ) ) ;
#33812=FACE_BOUND ( 'NONE', #13307, .T. ) ;
#33816=DIRECTION ( 'NONE',  ( 0.000000000000000000, 0.000000000000000000, 1.000000000000000000 ) ) ;
#33817=CARTESIAN_POINT ( 'NONE',  ( 4.476901250629513385, 26.36149378532653031, 6.000000000000000000 ) ) ;
#33834=DIRECTION ( 'NONE',  ( 0.000000000000000000, 0.000000000000000000, 1.000000000000000000 ) ) ;
#33840=ORIENTED_EDGE ( 'NONE', *, *, #31342, .T. ) ;
#33843=DIRECTION ( 'NONE',  ( 1.000000000000000000, 0.000000000000000000, 0.000000000000000000 ) ) ;
#33847=ORIENTED_EDGE ( 'NONE', *, *, #27248, .T. ) ;
#33869=CARTESIAN_POINT ( 'NONE',  ( -3.458872323573595864, 26.51478363815348160, 12.00000000000000000 ) ) ;
#33874=AXIS2_PLACEMENT_3D ( 'NONE', #22983, #38024, #16700 ) ;
#33879=ORIENTED_EDGE ( 'NONE', *, *, #37381, .F. ) ;
#33881=EDGE_CURVE ( 'NONE', #40077, #9569, #33023, .T. ) ;
#33891=ORIENTED_EDGE ( 'NONE', *, *, #25894, .F. ) ;
#33895=DIRECTION ( 'NONE',  ( 1.000000000000000000, 0.000000000000000000, 0.000000000000000000 ) ) ;
#33896=DIRECTION ( 'NONE',  ( 0.000000000000000000, 0.000000000000000000, 1.000000000000000000 ) ) ;
#33900=ADVANCED_FACE ( 'NONE', ( #8620 ), #30563, .F. ) ;
#33920=CARTESIAN_POINT ( 'NONE',  ( -6.953812613386785912, 14.77701242934787906, 13.00000000000000178 ) ) ;
#33923=AXIS2_PLACEMENT_3D ( 'NONE', #27699, #18174, #40091 ) ;
#33933=ORIENTED_EDGE ( 'NONE', *, *, #40180, .T. ) ;
#33935=CARTESIAN_POINT ( 'NONE',  ( 6.688300058587269170, 16.47782454277055564, 12.00000000000000000 ) ) ;
#33937=ORIENTED_EDGE ( 'NONE', *, *, #30624, .F. ) ;
#33947=ADVANCED_FACE ( 'NONE', ( #9421 ), #22393, .F. ) ;
#33960=CARTESIAN_POINT ( 'NONE',  ( -4.724378136954611840, 12.76962061027129458, 6.000000000000000000 ) ) ;
#33962=FACE_OUTER_BOUND ( 'NONE', #5275, .T. ) ;
#33967=AXIS2_PLACEMENT_3D ( 'NONE', #5423, #8060, #13958 ) ;
#33977=AXIS2_PLACEMENT_3D ( 'NONE', #1785, #30216, #26964 ) ;
#33978=VERTEX_POINT ( 'NONE', #18520 ) ;
#33979=EDGE_CURVE ( 'NONE', #6485, #30397, #15305, .T. ) ;
#33982=CARTESIAN_POINT ( 'NONE',  ( -5.348113209407908464, 9.835177808069893501, 12.00000000000000000 ) ) ;
#34001=CYLINDRICAL_SURFACE ( 'NONE', #23954, 1.000000000000000888 ) ;
#34002=CARTESIAN_POINT ( 'NONE',  ( 8.806975420853749625, 31.15003855377755571, 13.00000000000000178 ) ) ;
#34004=VECTOR ( 'NONE', #18820, 1000.000000000000000 ) ;
#34005=FACE_OUTER_BOUND ( 'NONE', #7077, .T. ) ;
#34013=CARTESIAN_POINT ( 'NONE',  ( -9.917741276437942233, 30.52956727630665057, 12.00000000000000000 ) ) ;
#34016=ORIENTED_EDGE ( 'NONE', *, *, #30713, .F. ) ;
#34020=CARTESIAN_POINT ( 'NONE',  ( -0.6057027746881266106, 27.44183462127829642, 13.00000000000000178 ) ) ;
#34022=EDGE_LOOP ( 'NONE', ( #15592, #21984, #26839, #2191 ) ) ;
#34023=CARTESIAN_POINT ( 'NONE',  ( 12.39463915635820612, 18.33192650902018883, 13.00000000000000178 ) ) ;
#34024=VERTEX_POINT ( 'NONE', #19457 ) ;
#34028=DIRECTION ( 'NONE',  ( 1.000000000000000000, 0.000000000000000000, 0.000000000000000000 ) ) ;
#34031=AXIS2_PLACEMENT_3D ( 'NONE', #9725, #8567, #20967 ) ;
#34035=EDGE_LOOP ( 'NONE', ( #4881, #23467 ) ) ;
#34058=CARTESIAN_POINT ( 'NONE',  ( -4.476907992048016816, 18.63850621467409496, 12.00000000000000000 ) ) ;
#34060=CARTESIAN_POINT ( 'NONE',  ( -0.6057027746881266106, 27.44183462127829642, 6.000000000000000000 ) ) ;
#34061=VECTOR ( 'NONE', #26367, 1000.000000000000000 ) ;
#34067=CARTESIAN_POINT ( 'NONE',  ( -3.853172919594720192, 21.57294901687549427, 6.000000000000000000 ) ) ;
#34077=AXIS2_PLACEMENT_3D ( 'NONE', #14011, #6064, #2625 ) ;
#34088=ORIENTED_EDGE ( 'NONE', *, *, #35457, .F. ) ;
#34097=ORIENTED_EDGE ( 'NONE', *, *, #38799, .F. ) ;
#34101=VECTOR ( 'NONE', #37100, 1000.000000000000000 ) ;
#34108=CARTESIAN_POINT ( 'NONE',  ( 8.935770203493859754, 22.34671014717335780, 6.000000000000000000 ) ) ;
#34110=DIRECTION ( 'NONE',  ( 0.000000000000000000, 0.000000000000000000, 1.000000000000000000 ) ) ;
#34128=VERTEX_POINT ( 'NONE', #8975 ) ;
#34130=AXIS2_PLACEMENT_3D ( 'NONE', #39659, #8986, #2690 ) ;
#34131=DIRECTION ( 'NONE',  ( 0.000000000000000000, 0.000000000000000000, 1.000000000000000000 ) ) ;
#34132=DIRECTION ( 'NONE',  ( 1.000000000000000000, 0.000000000000000000, 0.000000000000000000 ) ) ;
#34140=CARTESIAN_POINT ( 'NONE',  ( -12.64211604268330724, 20.79918788657763429, 6.000000000000000000 ) ) ;
#34144=ORIENTED_EDGE ( 'NONE', *, *, #14106, .T. ) ;
#34148=CARTESIAN_POINT ( 'NONE',  ( -1.871208588069141143, 13.69667159339610762, 6.000000000000000000 ) ) ;
#34155=CARTESIAN_POINT ( 'NONE',  ( 9.183240348400453001, 28.21559575157615996, 12.00000000000000000 ) ) ;
#34165=CYLINDRICAL_SURFACE ( 'NONE', #38141, 1.000000000000000000 ) ;
#34170=CYLINDRICAL_SURFACE ( 'NONE', #10106, 1.000000000000000000 ) ;
#34176=FACE_BOUND ( 'NONE', #2422, .T. ) ;
#34177=VERTEX_POINT ( 'NONE', #15266 ) ;
#34181=EDGE_LOOP ( 'NONE', ( #10926, #5874, #14595, #19888 ) ) ;
#34189=AXIS2_PLACEMENT_3D ( 'NONE', #15341, #13078, #34626 ) ;
#34193=ORIENTED_EDGE ( 'NONE', *, *, #40127, .T. ) ;
#34196=ADVANCED_FACE ( 'NONE', ( #27656 ), #24611, .T. ) ;
#34200=FACE_OUTER_BOUND ( 'NONE', #32228, .T. ) ;
#34205=CARTESIAN_POINT ( 'NONE',  ( 0.000000000000000000, 22.50000000000000355, 13.00000000000000178 ) ) ;
#34217=EDGE_LOOP ( 'NONE', ( #8039, #36177 ) ) ;
#34218=DIRECTION ( 'NONE',  ( 0.000000000000000000, 0.000000000000000000, 1.000000000000000000 ) ) ;
#34222=FACE_OUTER_BOUND ( 'NONE', #4919, .T. ) ;
#34223=EDGE_CURVE ( 'NONE', #12836, #30326, #15969, .T. ) ;
#34242=EDGE_LOOP ( 'NONE', ( #6924, #3558, #5532, #516 ) ) ;
#34248=ADVANCED_FACE ( 'NONE', ( #25950 ), #35510, .F. ) ;
#34252=CIRCLE ( 'NONE', #16742, 1.000000000000000000 ) ;
#34259=LINE ( 'NONE', #9474, #35500 ) ;
#34260=DIRECTION ( 'NONE',  ( 0.000000000000000000, 0.000000000000000000, 1.000000000000000000 ) ) ;
#34261=LINE ( 'NONE', #9679, #34004 ) ;
#34266=CARTESIAN_POINT ( 'NONE',  ( -1.871208588069141143, 13.69667159339610762, 12.00000000000000000 ) ) ;
#34272=ORIENTED_EDGE ( 'NONE', *, *, #19953, .F. ) ;
#34273=CARTESIAN_POINT ( 'NONE',  ( -2.871208588069141143, 13.69667159339610762, 12.00000000000000000 ) ) ;
#34276=AXIS2_PLACEMENT_3D ( 'NONE', #39579, #33896, #15597 ) ;
#34286=CIRCLE ( 'NONE', #24539, 1.000000000000000000 ) ;
#34289=DIRECTION ( 'NONE',  ( 0.000000000000000000, 0.000000000000000000, 1.000000000000000000 ) ) ;
#34296=ORIENTED_EDGE ( 'NONE', *, *, #1577, .F. ) ;
#34299=VECTOR ( 'NONE', #37762, 1000.000000000000000 ) ;
#34302=VERTEX_POINT ( 'NONE', #29610 ) ;
#34309=CARTESIAN_POINT ( 'NONE',  ( -6.935776944912362296, 22.65328985282726393, 13.00000000000000178 ) ) ;
#34313=DIRECTION ( 'NONE',  ( 1.000000000000000000, 0.000000000000000000, 0.000000000000000000 ) ) ;
#34318=FACE_OUTER_BOUND ( 'NONE', #4932, .T. ) ;
#34330=AXIS2_PLACEMENT_3D ( 'NONE', #21370, #15070, #39847 ) ;
#34331=CIRCLE ( 'NONE', #26557, 1.000000000000000888 ) ;
#34339=CIRCLE ( 'NONE', #21346, 1.000000000000000000 ) ;
#34344=VERTEX_POINT ( 'NONE', #13763 ) ;
#34366=ORIENTED_EDGE ( 'NONE', *, *, #23412, .F. ) ;
#34370=CARTESIAN_POINT ( 'NONE',  ( -13.03641663870442891, 15.85735326529964873, 12.00000000000000000 ) ) ;
#34371=EDGE_LOOP ( 'NONE', ( #11501, #1354, #14787, #34688 ) ) ;
#34376=FACE_BOUND ( 'NONE', #20983, .T. ) ;
#34377=ORIENTED_EDGE ( 'NONE', *, *, #39692, .T. ) ;
#34391=ORIENTED_EDGE ( 'NONE', *, *, #29746, .F. ) ;
#34393=AXIS2_PLACEMENT_3D ( 'NONE', #38745, #29399, #24104 ) ;
#34399=EDGE_CURVE ( 'NONE', #6396, #10818, #9389, .T. ) ;
#34401=FACE_BOUND ( 'NONE', #32907, .T. ) ;
#34404=CARTESIAN_POINT ( 'NONE',  ( 10.18324034840045478, 28.21559575157615996, 6.000000000000000000 ) ) ;
#34422=CARTESIAN_POINT ( 'NONE',  ( 11.89031559783844827, 11.79390851039467236, 12.00000000000000000 ) ) ;
#34430=DIRECTION ( 'NONE',  ( 1.000000000000000000, 0.000000000000000000, 0.000000000000000000 ) ) ;
#34433=DIRECTION ( 'NONE',  ( 0.000000000000000000, 0.000000000000000000, 1.000000000000000000 ) ) ;
#34434=VERTEX_POINT ( 'NONE', #33869 ) ;
#34437=VECTOR ( 'NONE', #12060, 1000.000000000000000 ) ;
#34444=AXIS2_PLACEMENT_3D ( 'NONE', #10368, #20319, #4472 ) ;
#34445=DIRECTION ( 'NONE',  ( 0.000000000000000000, 0.000000000000000000, 1.000000000000000000 ) ) ;
#34448=DIRECTION ( 'NONE',  ( 0.000000000000000000, 0.000000000000000000, 1.000000000000000000 ) ) ;
#34462=DIRECTION ( 'NONE',  ( 1.000000000000000000, 0.000000000000000000, 0.000000000000000000 ) ) ;
#34470=DIRECTION ( 'NONE',  ( 1.000000000000000000, 0.000000000000000000, 0.000000000000000000 ) ) ;
#34472=EDGE_CURVE ( 'NONE', #1614, #34434, #1678, .T. ) ;
#34478=EDGE_CURVE ( 'NONE', #24820, #12832, #29575, .T. ) ;
#34492=CIRCLE ( 'NONE', #11783, 1.000000000000000000 ) ;
#34494=ORIENTED_EDGE ( 'NONE', *, *, #13823, .T. ) ;
#34495=LINE ( 'NONE', #35844, #18075 ) ;
#34499=EDGE_CURVE ( 'NONE', #6918, #31607, #37944, .T. ) ;
#34505=LINE ( 'NONE', #28201, #20184 ) ;
#34506=DIRECTION ( 'NONE',  ( 0.000000000000000000, 0.000000000000000000, 1.000000000000000000 ) ) ;
#34513=DIRECTION ( 'NONE',  ( 0.000000000000000000, 0.000000000000000000, 1.000000000000000000 ) ) ;
#34521=EDGE_CURVE ( 'NONE', #27468, #6833, #28200, .T. ) ;
#34527=DIRECTION ( 'NONE',  ( 0.000000000000000000, 0.000000000000000000, 1.000000000000000000 ) ) ;
#34531=DIRECTION ( 'NONE',  ( 1.000000000000000000, 0.000000000000000000, 0.000000000000000000 ) ) ;
#34532=CIRCLE ( 'NONE', #26736, 1.000000000000000888 ) ;
#34539=AXIS2_PLACEMENT_3D ( 'NONE', #12583, #38167, #12780 ) ;
#34542=CYLINDRICAL_SURFACE ( 'NONE', #2178, 1.000000000000000000 ) ;
#34550=CARTESIAN_POINT ( 'NONE',  ( -2.605702774688126500, 27.44183462127829642, 13.00000000000000178 ) ) ;
#34560=ORIENTED_EDGE ( 'NONE', *, *, #17836, .T. ) ;
#34562=AXIS2_PLACEMENT_3D ( 'NONE', #32128, #4292, #453 ) ;
#34565=LINE ( 'NONE', #16075, #17291 ) ;
#34566=EDGE_LOOP ( 'NONE', ( #3768, #28680 ) ) ;
#34570=FACE_BOUND ( 'NONE', #1226, .T. ) ;
#34575=ORIENTED_EDGE ( 'NONE', *, *, #38359, .T. ) ;
#34585=DIRECTION ( 'NONE',  ( 1.000000000000000000, 0.000000000000000000, 0.000000000000000000 ) ) ;
#34590=CIRCLE ( 'NONE', #3445, 1.000000000000000000 ) ;
#34595=VECTOR ( 'NONE', #34843, 1000.000000000000000 ) ;
#34603=AXIS2_PLACEMENT_3D ( 'NONE', #4476, #4677, #16881 ) ;
#34604=ORIENTED_EDGE ( 'NONE', *, *, #24651, .T. ) ;
#34608=DIRECTION ( 'NONE',  ( 1.000000000000000000, 0.000000000000000000, 0.000000000000000000 ) ) ;
#34610=ORIENTED_EDGE ( 'NONE', *, *, #35998, .T. ) ;
#34611=DIRECTION ( 'NONE',  ( 0.000000000000000000, 0.000000000000000000, 1.000000000000000000 ) ) ;
#34612=EDGE_LOOP ( 'NONE', ( #24225, #8316, #34377, #460 ) ) ;
#34620=LINE ( 'NONE', #26070, #29991 ) ;
#34622=ORIENTED_EDGE ( 'NONE', *, *, #19795, .T. ) ;
#34626=DIRECTION ( 'NONE',  ( 1.000000000000000000, 0.000000000000000000, 0.000000000000000000 ) ) ;
#34634=ORIENTED_EDGE ( 'NONE', *, *, #2395, .T. ) ;
#34641=CIRCLE ( 'NONE', #17151, 1.000000000000000000 ) ;
#34648=CARTESIAN_POINT ( 'NONE',  ( 0.6417673702184640838, 33.31072022568110924, 12.00000000000000000 ) ) ;
#34665=ORIENTED_EDGE ( 'NONE', *, *, #39973, .T. ) ;
#34669=CIRCLE ( 'NONE', #5464, 1.000000000000000000 ) ;
#34675=LINE ( 'NONE', #3001, #30334 ) ;
#34680=CIRCLE ( 'NONE', #8082, 1.000000000000000000 ) ;
#34683=DIRECTION ( 'NONE',  ( 0.000000000000000000, 0.000000000000000000, 1.000000000000000000 ) ) ;
#34688=ORIENTED_EDGE ( 'NONE', *, *, #20961, .F. ) ;
#34692=FACE_OUTER_BOUND ( 'NONE', #22016, .T. ) ;
#34701=DIRECTION ( 'NONE',  ( 0.000000000000000000, 0.000000000000000000, 1.000000000000000000 ) ) ;
#34721=EDGE_CURVE ( 'NONE', #10357, #32704, #3180, .T. ) ;
#34724=ADVANCED_FACE ( 'NONE', ( #15968 ), #16169, .F. ) ;
#34725=EDGE_CURVE ( 'NONE', #15697, #28039, #15570, .T. ) ;
#34731=CARTESIAN_POINT ( 'NONE',  ( -7.577547685840081648, 11.84256962714647798, 13.00000000000000178 ) ) ;
#34747=ORIENTED_EDGE ( 'NONE', *, *, #21043, .T. ) ;
#34748=EDGE_CURVE ( 'NONE', #28039, #6207, #24956, .T. ) ;
#34752=DIRECTION ( 'NONE',  ( 0.000000000000000000, 0.000000000000000000, 1.000000000000000000 ) ) ;
#34767=DIRECTION ( 'NONE',  ( 0.000000000000000000, 0.000000000000000000, 1.000000000000000000 ) ) ;
#34768=ORIENTED_EDGE ( 'NONE', *, *, #39580, .F. ) ;
#34772=FACE_BOUND ( 'NONE', #21005, .T. ) ;
#34774=DIRECTION ( 'NONE',  ( 1.000000000000000000, 0.000000000000000000, 0.000000000000000000 ) ) ;
#34775=ORIENTED_EDGE ( 'NONE', *, *, #26727, .F. ) ;
#34777=DIRECTION ( 'NONE',  ( 0.000000000000000000, 0.000000000000000000, 1.000000000000000000 ) ) ;
#34780=ORIENTED_EDGE ( 'NONE', *, *, #18060, .T. ) ;
#34784=CARTESIAN_POINT ( 'NONE',  ( -2.118678732975735279, 7.827785988993307242, 6.000000000000000000 ) ) ;
#34788=AXIS2_PLACEMENT_3D ( 'NONE', #9980, #638, #22561 ) ;
#34795=FACE_BOUND ( 'NONE', #17817, .T. ) ;
#34799=DIRECTION ( 'NONE',  ( 1.000000000000000000, 0.000000000000000000, 0.000000000000000000 ) ) ;
#34801=ORIENTED_EDGE ( 'NONE', *, *, #14799, .T. ) ;
#34809=ORIENTED_EDGE ( 'NONE', *, *, #34478, .F. ) ;
#34814=AXIS2_PLACEMENT_3D ( 'NONE', #9654, #28325, #21633 ) ;
#34833=EDGE_CURVE ( 'NONE', #33301, #30382, #35462, .T. ) ;
#34843=DIRECTION ( 'NONE',  ( 0.000000000000000000, 0.000000000000000000, 1.000000000000000000 ) ) ;
#34845=CARTESIAN_POINT ( 'NONE',  ( 5.330070799514983193, 27.28854476845134513, 13.00000000000000178 ) ) ;
#34847=EDGE_CURVE ( 'NONE', #34128, #15652, #10051, .T. ) ;
#34858=CARTESIAN_POINT ( 'NONE',  ( 4.458865582155095986, 18.48521636184714012, 6.000000000000000000 ) ) ;
#34861=DIRECTION ( 'NONE',  ( 1.000000000000000000, 0.000000000000000000, 0.000000000000000000 ) ) ;
#34862=CARTESIAN_POINT ( 'NONE',  ( -13.64211604268330724, 20.79918788657763429, 6.000000000000000000 ) ) ;
#34866=EDGE_LOOP ( 'NONE', ( #37739, #6717 ) ) ;
#34875=ORIENTED_EDGE ( 'NONE', *, *, #27246, .F. ) ;
#34882=CIRCLE ( 'NONE', #32272, 1.000000000000000000 ) ;
#34892=EDGE_LOOP ( 'NONE', ( #22082, #13712 ) ) ;
#34893=DIRECTION ( 'NONE',  ( 0.000000000000000000, 0.000000000000000000, 1.000000000000000000 ) ) ;
#34900=EDGE_CURVE ( 'NONE', #12932, #3455, #314, .T. ) ;
#34902=DIRECTION ( 'NONE',  ( 0.000000000000000000, 0.000000000000000000, 1.000000000000000000 ) ) ;
#34908=VECTOR ( 'NONE', #23840, 1000.000000000000000 ) ;
#34911=DIRECTION ( 'NONE',  ( 0.000000000000000000, 0.000000000000000000, 1.000000000000000000 ) ) ;
#34930=EDGE_LOOP ( 'NONE', ( #20206, #8782 ) ) ;
#34945=CYLINDRICAL_SURFACE ( 'NONE', #29398, 1.000000000000000000 ) ;
#34952=MANIFOLD_SOLID_BREP ( 'Fill Pattern1', #7328 ) ;
#34965=ORIENTED_EDGE ( 'NONE', *, *, #11864, .T. ) ;
#34971=ORIENTED_EDGE ( 'NONE', *, *, #22945, .T. ) ;
#34972=ORIENTED_EDGE ( 'NONE', *, *, #22246, .T. ) ;
#34976=EDGE_CURVE ( 'NONE', #35589, #12341, #5495, .T. ) ;
#34977=LINE ( 'NONE', #32330, #19152 ) ;
#34993=ORIENTED_EDGE ( 'NONE', *, *, #18589, .F. ) ;
#34999=LINE ( 'NONE', #38242, #9018 ) ;
#35004=FACE_BOUND ( 'NONE', #8943, .T. ) ;
#35011=ORIENTED_EDGE ( 'NONE', *, *, #33465, .F. ) ;
#35018=DIRECTION ( 'NONE',  ( 0.000000000000000000, 0.000000000000000000, 1.000000000000000000 ) ) ;
#35021=DIRECTION ( 'NONE',  ( 0.000000000000000000, 0.000000000000000000, 1.000000000000000000 ) ) ;
#35023=DIRECTION ( 'NONE',  ( 0.000000000000000000, 0.000000000000000000, 1.000000000000000000 ) ) ;
#35028=DIRECTION ( 'NONE',  ( 0.000000000000000000, 0.000000000000000000, 1.000000000000000000 ) ) ;
#35033=CYLINDRICAL_SURFACE ( 'NONE', #14170, 1.000000000000000000 ) ;
#35035=ORIENTED_EDGE ( 'NONE', *, *, #5916, .T. ) ;
#35039=EDGE_LOOP ( 'NONE', ( #26520, #21827, #6649, #22289 ) ) ;
#35041=DIRECTION ( 'NONE',  ( 1.000000000000000000, 0.000000000000000000, 0.000000000000000000 ) ) ;
#35042=DIRECTION ( 'NONE',  ( 1.000000000000000000, 0.000000000000000000, 0.000000000000000000 ) ) ;
#35044=CARTESIAN_POINT ( 'NONE',  ( 3.211395437248501850, 12.61633075744433796, 6.000000000000000000 ) ) ;
#35046=EDGE_CURVE ( 'NONE', #6333, #3736, #19799, .T. ) ;
#35048=DIRECTION ( 'NONE',  ( 1.000000000000000000, 0.000000000000000000, 0.000000000000000000 ) ) ;
#35062=ORIENTED_EDGE ( 'NONE', *, *, #2965, .F. ) ;
#35075=AXIS2_PLACEMENT_3D ( 'NONE', #31847, #4009, #32048 ) ;
#35079=ORIENTED_EDGE ( 'NONE', *, *, #6496, .F. ) ;
#35084=DIRECTION ( 'NONE',  ( 0.000000000000000000, 0.000000000000000000, 1.000000000000000000 ) ) ;
#35090=DIRECTION ( 'NONE',  ( 1.000000000000000000, 0.000000000000000000, 0.000000000000000000 ) ) ;
#35097=CARTESIAN_POINT ( 'NONE',  ( -0.3582326297815359162, 33.31072022568110924, 13.00000000000000178 ) ) ;
#35122=ORIENTED_EDGE ( 'NONE', *, *, #6094, .T. ) ;
#35124=EDGE_LOOP ( 'NONE', ( #22069, #21296 ) ) ;
#35127=ORIENTED_EDGE ( 'NONE', *, *, #1324, .F. ) ;
#35129=AXIS2_PLACEMENT_3D ( 'NONE', #5657, #20517, #30657 ) ;
#35134=ORIENTED_EDGE ( 'NONE', *, *, #20126, .T. ) ;
#35145=CARTESIAN_POINT ( 'NONE',  ( -1.605702774688126722, 27.44183462127829642, 6.000000000000000000 ) ) ;
#35150=ADVANCED_FACE ( 'NONE', ( #37904 ), #536, .F. ) ;
#35154=ORIENTED_EDGE ( 'NONE', *, *, #26694, .F. ) ;
#35159=DIRECTION ( 'NONE',  ( 1.000000000000000000, 0.000000000000000000, 0.000000000000000000 ) ) ;
#35169=FACE_OUTER_BOUND ( 'NONE', #34612, .T. ) ;
#35170=DIRECTION ( 'NONE',  ( 0.000000000000000000, 0.000000000000000000, 1.000000000000000000 ) ) ;
#35176=CARTESIAN_POINT ( 'NONE',  ( 2.871201846650637268, 31.30332840660451765, 6.000000000000000000 ) ) ;
#35177=DIRECTION ( 'NONE',  ( 1.000000000000000000, 0.000000000000000000, 0.000000000000000000 ) ) ;
#35195=FACE_BOUND ( 'NONE', #13380, .T. ) ;
#35206=CARTESIAN_POINT ( 'NONE',  ( -10.77091082532341204, 29.60251629318183575, 13.00000000000000178 ) ) ;
#35213=DIRECTION ( 'NONE',  ( 0.000000000000000000, 0.000000000000000000, 1.000000000000000000 ) ) ;
#35225=AXIS2_PLACEMENT_3D ( 'NONE', #12474, #24868, #21618 ) ;
#35230=EDGE_CURVE ( 'NONE', #26705, #32832, #36047, .T. ) ;
#35241=AXIS2_PLACEMENT_3D ( 'NONE', #30556, #6154, #2716 ) ;
#35243=AXIS2_PLACEMENT_3D ( 'NONE', #29389, #10707, #26950 ) ;
#35250=CARTESIAN_POINT ( 'NONE',  ( 10.41267482483262619, 26.20820393249957192, 6.000000000000000000 ) ) ;
#35252=CARTESIAN_POINT ( 'NONE',  ( 4.118671991557230072, 37.17221401100731981, 6.000000000000000000 ) ) ;
#35268=CARTESIAN_POINT ( 'NONE',  ( 4.100636323082810009, 29.29593658752792962, 6.000000000000000000 ) ) ;
#35275=ORIENTED_EDGE ( 'NONE', *, *, #16116, .F. ) ;
#35280=ORIENTED_EDGE ( 'NONE', *, *, #22114, .F. ) ;
#35306=ORIENTED_EDGE ( 'NONE', *, *, #11083, .F. ) ;
#35312=DIRECTION ( 'NONE',  ( 1.000000000000000000, 0.000000000000000000, 0.000000000000000000 ) ) ;
#35316=AXIS2_PLACEMENT_3D ( 'NONE', #13346, #10923, #38134 ) ;
#35323=VERTEX_POINT ( 'NONE', #14732 ) ;
#35337=ORIENTED_EDGE ( 'NONE', *, *, #23296, .T. ) ;
#35342=SHAPE_REPRESENTATION_RELATIONSHIP ( 'NONE' , 'NONE' ,  #33787, #3225 ) ;
#35344=EDGE_CURVE ( 'NONE', #25235, #21075, #20233, .T. ) ;
#35347=CARTESIAN_POINT ( 'NONE',  ( 6.953805871968278929, 30.22298757065274444, 12.00000000000000000 ) ) ;
#35349=VECTOR ( 'NONE', #28939, 1000.000000000000000 ) ;
#35353=CARTESIAN_POINT ( 'NONE',  ( 11.39463915635820612, 18.33192650902018883, 12.00000000000000000 ) ) ;
#35359=CARTESIAN_POINT ( 'NONE',  ( 6.953805871968278929, 30.22298757065274444, 6.000000000000000000 ) ) ;
#35365=DIRECTION ( 'NONE',  ( 1.000000000000000000, 0.000000000000000000, 0.000000000000000000 ) ) ;
#35374=CIRCLE ( 'NONE', #24352, 1.000000000000000000 ) ;
#35377=AXIS2_PLACEMENT_3D ( 'NONE', #1781, #32865, #14162 ) ;
#35379=CIRCLE ( 'NONE', #22455, 1.000000000000000888 ) ;
#35383=DIRECTION ( 'NONE',  ( 0.000000000000000000, 0.000000000000000000, 1.000000000000000000 ) ) ;
#35385=ORIENTED_EDGE ( 'NONE', *, *, #35436, .F. ) ;
#35387=EDGE_CURVE ( 'NONE', #20746, #6207, #35868, .T. ) ;
#35389=ORIENTED_EDGE ( 'NONE', *, *, #8508, .T. ) ;
#35400=AXIS2_PLACEMENT_3D ( 'NONE', #3680, #31911, #4284 ) ;
#35402=CIRCLE ( 'NONE', #13972, 1.000000000000000000 ) ;
#35403=CYLINDRICAL_SURFACE ( 'NONE', #29464, 1.000000000000000000 ) ;
#35406=EDGE_CURVE ( 'NONE', #7, #14009, #32152, .T. ) ;
#35408=CARTESIAN_POINT ( 'NONE',  ( -5.082607396026893376, 23.58034083595207875, 6.000000000000000000 ) ) ;
#35416=EDGE_LOOP ( 'NONE', ( #28666, #34622 ) ) ;
#35418=DIRECTION ( 'NONE',  ( 0.000000000000000000, 0.000000000000000000, 1.000000000000000000 ) ) ;
#35421=FACE_OUTER_BOUND ( 'NONE', #11834, .T. ) ;
#35424=VERTEX_POINT ( 'NONE', #16985 ) ;
#35432=DIRECTION ( 'NONE',  ( 1.000000000000000000, 0.000000000000000000, 0.000000000000000000 ) ) ;
#35436=EDGE_CURVE ( 'NONE', #24757, #18996, #33036, .T. ) ;
#35439=EDGE_CURVE ( 'NONE', #17409, #40053, #35374, .T. ) ;
#35451=CARTESIAN_POINT ( 'NONE',  ( -0.8712085880691411433, 13.69667159339610762, 13.00000000000000178 ) ) ;
#35452=EDGE_LOOP ( 'NONE', ( #22727, #11154, #2566, #1008 ) ) ;
#35457=EDGE_CURVE ( 'NONE', #38453, #7138, #33456, .T. ) ;
#35462=LINE ( 'NONE', #16978, #8754 ) ;
#35470=EDGE_LOOP ( 'NONE', ( #11107, #24389, #20174, #13175 ) ) ;
#35472=ORIENTED_EDGE ( 'NONE', *, *, #3052, .F. ) ;
#35485=VERTEX_POINT ( 'NONE', #9035 ) ;
#35487=ADVANCED_FACE ( 'NONE', ( #37060 ), #39707, .F. ) ;
#35496=CIRCLE ( 'NONE', #5644, 1.000000000000000000 ) ;
#35499=CARTESIAN_POINT ( 'NONE',  ( 10.18324034840045478, 28.21559575157615996, 12.00000000000000000 ) ) ;
#35500=VECTOR ( 'NONE', #27952, 1000.000000000000000 ) ;
#35502=EDGE_LOOP ( 'NONE', ( #3528, #35794 ) ) ;
#35510=CYLINDRICAL_SURFACE ( 'NONE', #12713, 1.000000000000000888 ) ;
#35513=DIRECTION ( 'NONE',  ( 1.000000000000000000, 0.000000000000000000, 0.000000000000000000 ) ) ;
#35529=AXIS2_PLACEMENT_3D ( 'NONE', #711, #38486, #35041 ) ;
#35532=AXIS2_PLACEMENT_3D ( 'NONE', #29986, #30192, #8043 ) ;
#35534=ORIENTED_EDGE ( 'NONE', *, *, #20636, .F. ) ;
#35549=CIRCLE ( 'NONE', #36195, 1.000000000000000000 ) ;
#35551=ORIENTED_EDGE ( 'NONE', *, *, #2717, .F. ) ;
#35553=FACE_OUTER_BOUND ( 'NONE', #20199, .T. ) ;
#35569=EDGE_CURVE ( 'NONE', #10001, #8098, #6176, .T. ) ;
#35575=CYLINDRICAL_SURFACE ( 'NONE', #17868, 1.000000000000000888 ) ;
#35586=CARTESIAN_POINT ( 'NONE',  ( -7.312041872459064784, 25.58773265502866678, 12.00000000000000000 ) ) ;
#35587=UNCERTAINTY_MEASURE_WITH_UNIT (LENGTH_MEASURE( 1.000000000000000082E-05 ), #35664, 'distance_accuracy_value', 'NONE');
#35588=CIRCLE ( 'NONE', #6361, 1.000000000000000888 ) ;
#35589=VERTEX_POINT ( 'NONE', #24666 ) ;
#35591=ORIENTED_EDGE ( 'NONE', *, *, #22054, .T. ) ;
#35596=EDGE_LOOP ( 'NONE', ( #33689, #16248 ) ) ;
#35605=AXIS2_PLACEMENT_3D ( 'NONE', #13979, #23330, #35726 ) ;
#35611=AXIS2_PLACEMENT_3D ( 'NONE', #38443, #1069, #16918 ) ;
#35613=DIRECTION ( 'NONE',  ( 0.000000000000000000, 0.000000000000000000, 1.000000000000000000 ) ) ;
#35614=EDGE_CURVE ( 'NONE', #11394, #34302, #32807, .T. ) ;
#35617=EDGE_LOOP ( 'NONE', ( #35551, #20185, #2531, #37875 ) ) ;
#35634=VERTEX_POINT ( 'NONE', #34020 ) ;
#35636=DIRECTION ( 'NONE',  ( 0.000000000000000000, 0.000000000000000000, 1.000000000000000000 ) ) ;
#35637=DIRECTION ( 'NONE',  ( 0.000000000000000000, 0.000000000000000000, 1.000000000000000000 ) ) ;
#35638=EDGE_LOOP ( 'NONE', ( #24025, #23936, #10373, #5813 ) ) ;
#35642=AXIS2_PLACEMENT_3D ( 'NONE', #2583, #2975, #2384 ) ;
#35648=CIRCLE ( 'NONE', #36947, 18.00000000000000000 ) ;
#35651=CARTESIAN_POINT ( 'NONE',  ( -6.348113209407908464, 9.835177808069893501, 12.00000000000000000 ) ) ;
#35652=CARTESIAN_POINT ( 'NONE',  ( 11.14716901145161643, 12.46304090461738667, 6.000000000000000000 ) ) ;
#35654=FACE_OUTER_BOUND ( 'NONE', #24551, .T. ) ;
#35664=( LENGTH_UNIT ( ) NAMED_UNIT ( * ) SI_UNIT ( .MILLI., .METRE. ) );
#35665=AXIS2_PLACEMENT_3D ( 'NONE', #39890, #21411, #30765 ) ;
#35686=DIRECTION ( 'NONE',  ( 0.000000000000000000, 0.000000000000000000, 1.000000000000000000 ) ) ;
#35693=DIRECTION ( 'NONE',  ( 1.000000000000000000, 0.000000000000000000, 0.000000000000000000 ) ) ;
#35695=EDGE_CURVE ( 'NONE', #7177, #22373, #15302, .T. ) ;
#35702=AXIS2_PLACEMENT_3D ( 'NONE', #6596, #12901, #25297 ) ;
#35703=CARTESIAN_POINT ( 'NONE',  ( 5.724371395536106633, 32.23037938972932892, 12.00000000000000000 ) ) ;
#35704=DIRECTION ( 'NONE',  ( 1.000000000000000000, 0.000000000000000000, 0.000000000000000000 ) ) ;
#35705=CYLINDRICAL_SURFACE ( 'NONE', #11059, 1.000000000000000888 ) ;
#35710=CARTESIAN_POINT ( 'NONE',  ( -13.03641663870442891, 15.85735326529964873, 6.000000000000000000 ) ) ;
#35711=DIRECTION ( 'NONE',  ( 0.000000000000000000, 0.000000000000000000, 1.000000000000000000 ) ) ;
#35712=ADVANCED_FACE ( 'NONE', ( #10425 ), #38256, .F. ) ;
#35719=CARTESIAN_POINT ( 'NONE',  ( 5.348106467989403257, 35.16482219193073178, 12.00000000000000000 ) ) ;
#35720=CARTESIAN_POINT ( 'NONE',  ( 6.706335727061685681, 24.35410196624994583, 6.000000000000000000 ) ) ;
#35726=DIRECTION ( 'NONE',  ( 1.000000000000000000, 0.000000000000000000, 0.000000000000000000 ) ) ;
#35732=DIRECTION ( 'NONE',  ( 1.000000000000000000, 0.000000000000000000, 0.000000000000000000 ) ) ;
#35752=DIRECTION ( 'NONE',  ( 0.000000000000000000, 0.000000000000000000, 1.000000000000000000 ) ) ;
#35756=DIRECTION ( 'NONE',  ( 0.000000000000000000, 0.000000000000000000, 1.000000000000000000 ) ) ;
#35758=CIRCLE ( 'NONE', #18249, 1.000000000000000000 ) ;
#35762=ORIENTED_EDGE ( 'NONE', *, *, #20895, .T. ) ;
#35777=ORIENTED_EDGE ( 'NONE', *, *, #39048, .T. ) ;
#35780=FACE_BOUND ( 'NONE', #9099, .T. ) ;
#35785=CARTESIAN_POINT ( 'NONE',  ( -8.294006203984645609, 33.46401007850805343, 12.00000000000000000 ) ) ;
#35794=ORIENTED_EDGE ( 'NONE', *, *, #33261, .T. ) ;
#35796=EDGE_CURVE ( 'NONE', #31499, #37740, #22809, .T. ) ;
#35798=CARTESIAN_POINT ( 'NONE',  ( 11.78893975237933134, 23.27376113029817617, 13.00000000000000178 ) ) ;
#35800=CYLINDRICAL_SURFACE ( 'NONE', #38856, 1.000000000000000888 ) ;
#35801=ORIENTED_EDGE ( 'NONE', *, *, #14799, .F. ) ;
#35803=DIRECTION ( 'NONE',  ( 1.000000000000000000, 0.000000000000000000, 0.000000000000000000 ) ) ;
#35813=VERTEX_POINT ( 'NONE', #35206 ) ;
#35816=EDGE_CURVE ( 'NONE', #9639, #23635, #19771, .T. ) ;
#35821=ORIENTED_EDGE ( 'NONE', *, *, #27780, .F. ) ;
#35823=DIRECTION ( 'NONE',  ( 1.000000000000000000, 0.000000000000000000, 0.000000000000000000 ) ) ;
#35825=CARTESIAN_POINT ( 'NONE',  ( -7.294006203984644721, 33.46401007850805343, 12.00000000000000000 ) ) ;
#35835=ORIENTED_EDGE ( 'NONE', *, *, #19306, .F. ) ;
#35840=EDGE_LOOP ( 'NONE', ( #21603, #12428 ) ) ;
#35844=CARTESIAN_POINT ( 'NONE',  ( 7.559505275947156377, 25.28115294937476065, 6.000000000000000000 ) ) ;
#35845=EDGE_CURVE ( 'NONE', #30103, #488, #372, .T. ) ;
#35848=CARTESIAN_POINT ( 'NONE',  ( -7.559512017365658920, 19.71884705062586107, 12.00000000000000000 ) ) ;
#35849=CIRCLE ( 'NONE', #23528, 1.000000000000000888 ) ;
#35854=LINE ( 'NONE', #35250, #24639 ) ;
#35861=ORIENTED_EDGE ( 'NONE', *, *, #22246, .F. ) ;
#35865=AXIS2_PLACEMENT_3D ( 'NONE', #8956, #36987, #24594 ) ;
#35868=LINE ( 'NONE', #11292, #16583 ) ;
#35874=FACE_OUTER_BOUND ( 'NONE', #24860, .T. ) ;
#35885=DIRECTION ( 'NONE',  ( 1.000000000000000000, 0.000000000000000000, 0.000000000000000000 ) ) ;
#35890=AXIS2_PLACEMENT_3D ( 'NONE', #12419, #12223, #12022 ) ;
#35899=LINE ( 'NONE', #32456, #13887 ) ;
#35900=EDGE_CURVE ( 'NONE', #12849, #10495, #19183, .T. ) ;
#35903=ORIENTED_EDGE ( 'NONE', *, *, #12815, .T. ) ;
#35908=DIRECTION ( 'NONE',  ( 0.000000000000000000, 0.000000000000000000, 1.000000000000000000 ) ) ;
#35909=VECTOR ( 'NONE', #3764, 1000.000000000000000 ) ;
#35910=DIRECTION ( 'NONE',  ( 0.000000000000000000, 0.000000000000000000, 1.000000000000000000 ) ) ;
#35916=AXIS2_PLACEMENT_3D ( 'NONE', #32663, #4619, #20470 ) ;
#35917=DIRECTION ( 'NONE',  ( 0.000000000000000000, 0.000000000000000000, 1.000000000000000000 ) ) ;
#35919=CARTESIAN_POINT ( 'NONE',  ( 8.806975420853749625, 31.15003855377755571, 6.000000000000000000 ) ) ;
#35924=AXIS2_PLACEMENT_3D ( 'NONE', #3765, #329, #6604 ) ;
#35931=EDGE_LOOP ( 'NONE', ( #34272, #244, #37382, #6418 ) ) ;
#35933=ORIENTED_EDGE ( 'NONE', *, *, #18952, .T. ) ;
#35942=ORIENTED_EDGE ( 'NONE', *, *, #36181, .T. ) ;
#35944=AXIS2_PLACEMENT_3D ( 'NONE', #31395, #7199, #13702 ) ;
#35945=EDGE_CURVE ( 'NONE', #34434, #37407, #11236, .T. ) ;
#35948=CARTESIAN_POINT ( 'NONE',  ( -0.6237384431625470071, 19.56555719779890978, 6.000000000000000000 ) ) ;
#35954=DIRECTION ( 'NONE',  ( 0.000000000000000000, 0.000000000000000000, 1.000000000000000000 ) ) ;
#35956=( NAMED_UNIT ( * ) PLANE_ANGLE_UNIT ( ) SI_UNIT ( $, .RADIAN. ) );
#35958=DIRECTION ( 'NONE',  ( 0.000000000000000000, 0.000000000000000000, 1.000000000000000000 ) ) ;
#35962=VECTOR ( 'NONE', #6595, 1000.000000000000000 ) ;
#35964=DIRECTION ( 'NONE',  ( 0.000000000000000000, 0.000000000000000000, 1.000000000000000000 ) ) ;
#35967=CARTESIAN_POINT ( 'NONE',  ( -2.494943660522439099, 10.76222879119470832, 13.00000000000000178 ) ) ;
#35968=ADVANCED_FACE ( 'NONE', ( #14477 ), #7572, .F. ) ;
#35971=EDGE_CURVE ( 'NONE', #16598, #7337, #38660, .T. ) ;
#35973=AXIS2_PLACEMENT_3D ( 'NONE', #32468, #25947, #10931 ) ;
#35978=VERTEX_POINT ( 'NONE', #27666 ) ;
#35981=CARTESIAN_POINT ( 'NONE',  ( -14.26585111513660031, 17.86474508437623143, 6.000000000000000000 ) ) ;
#35998=EDGE_CURVE ( 'NONE', #20584, #25338, #21133, .T. ) ;
#36002=CARTESIAN_POINT ( 'NONE',  ( 7.688300058587269170, 16.47782454277055564, 12.00000000000000000 ) ) ;
#36008=CIRCLE ( 'NONE', #28225, 1.000000000000000000 ) ;
#36020=AXIS2_PLACEMENT_3D ( 'NONE', #1988, #38950, #29204 ) ;
#36027=ORIENTED_EDGE ( 'NONE', *, *, #4886, .F. ) ;
#36036=ORIENTED_EDGE ( 'NONE', *, *, #20915, .T. ) ;
#36040=ORIENTED_EDGE ( 'NONE', *, *, #38359, .F. ) ;
#36047=CIRCLE ( 'NONE', #25639, 1.000000000000000888 ) ;
#36049=DIRECTION ( 'NONE',  ( 1.000000000000000000, 0.000000000000000000, 0.000000000000000000 ) ) ;
#36051=VECTOR ( 'NONE', #8136, 1000.000000000000000 ) ;
#36058=DIRECTION ( 'NONE',  ( 0.000000000000000000, 0.000000000000000000, 1.000000000000000000 ) ) ;
#36061=DIRECTION ( 'NONE',  ( 0.000000000000000000, 0.000000000000000000, 1.000000000000000000 ) ) ;
#36065=ORIENTED_EDGE ( 'NONE', *, *, #32764, .F. ) ;
#36073=ORIENTED_EDGE ( 'NONE', *, *, #29990, .F. ) ;
#36087=CIRCLE ( 'NONE', #18563, 1.000000000000000888 ) ;
#36091=FACE_OUTER_BOUND ( 'NONE', #19580, .T. ) ;
#36100=EDGE_CURVE ( 'NONE', #20514, #7288, #40051, .T. ) ;
#36101=EDGE_LOOP ( 'NONE', ( #19944, #39817, #1063, #24595 ) ) ;
#36102=EDGE_CURVE ( 'NONE', #35323, #4132, #36618, .T. ) ;
#36106=CARTESIAN_POINT ( 'NONE',  ( -5.330077540933487512, 17.71145523154927659, 6.000000000000000000 ) ) ;
#36109=CARTESIAN_POINT ( 'NONE',  ( -8.183247089818959097, 16.78440424842446532, 12.00000000000000000 ) ) ;
#36110=VECTOR ( 'NONE', #35023, 1000.000000000000000 ) ;
#36119=CARTESIAN_POINT ( 'NONE',  ( 0.8712018466506370462, 31.30332840660451765, 13.00000000000000178 ) ) ;
#36126=DIRECTION ( 'NONE',  ( 1.000000000000000000, 0.000000000000000000, 0.000000000000000000 ) ) ;
#36131=CARTESIAN_POINT ( 'NONE',  ( -6.064571727552472424, 31.45661825943146894, 6.000000000000000000 ) ) ;
#36134=VERTEX_POINT ( 'NONE', #24621 ) ;
#36138=VERTEX_POINT ( 'NONE', #18140 ) ;
#36141=VERTEX_POINT ( 'NONE', #3284 ) ;
#36148=ADVANCED_FACE ( 'NONE', ( #30530 ), #34170, .F. ) ;
#36150=CARTESIAN_POINT ( 'NONE',  ( -5.348113209407908464, 9.835177808069893501, 13.00000000000000178 ) ) ;
#36152=ORIENTED_EDGE ( 'NONE', *, *, #6591, .F. ) ;
#36154=DIRECTION ( 'NONE',  ( 0.000000000000000000, 0.000000000000000000, 1.000000000000000000 ) ) ;
#36158=AXIS2_PLACEMENT_3D ( 'NONE', #8406, #20803, #33405 ) ;
#36160=VECTOR ( 'NONE', #27782, 1000.000000000000000 ) ;
#36163=DIRECTION ( 'NONE',  ( 1.000000000000000000, 0.000000000000000000, 0.000000000000000000 ) ) ;
#36177=ORIENTED_EDGE ( 'NONE', *, *, #8661, .F. ) ;
#36181=EDGE_CURVE ( 'NONE', #19810, #9924, #38002, .T. ) ;
#36183=VERTEX_POINT ( 'NONE', #242 ) ;
#36188=ORIENTED_EDGE ( 'NONE', *, *, #15267, .T. ) ;
#36195=AXIS2_PLACEMENT_3D ( 'NONE', #15544, #28324, #33843 ) ;
#36197=ORIENTED_EDGE ( 'NONE', *, *, #9993, .T. ) ;
#36200=AXIS2_PLACEMENT_3D ( 'NONE', #30604, #12898, #30994 ) ;
#36202=ADVANCED_FACE ( 'NONE', ( #12627 ), #4078, .F. ) ;
#36207=DIRECTION ( 'NONE',  ( -0.000000000000000000, -0.000000000000000000, -1.000000000000000000 ) ) ;
#36218=EDGE_LOOP ( 'NONE', ( #7506, #32489, #720, #11869 ) ) ;
#36221=VECTOR ( 'NONE', #35084, 1000.000000000000000 ) ;
#36236=LINE ( 'NONE', #27281, #14644 ) ;
#36239=ADVANCED_FACE ( 'NONE', ( #13217 ), #9585, .F. ) ;
#36246=FACE_OUTER_BOUND ( 'NONE', #38340, .T. ) ;
#36247=ORIENTED_EDGE ( 'NONE', *, *, #37458, .F. ) ;
#36261=DIRECTION ( 'NONE',  ( 0.000000000000000000, 0.000000000000000000, 1.000000000000000000 ) ) ;
#36274=EDGE_CURVE ( 'NONE', #4798, #24101, #29596, .T. ) ;
#36275=DIRECTION ( 'NONE',  ( 1.000000000000000000, 0.000000000000000000, 0.000000000000000000 ) ) ;
#36281=CARTESIAN_POINT ( 'NONE',  ( -2.853172919594720192, 21.57294901687549427, 6.000000000000000000 ) ) ;
#36289=EDGE_LOOP ( 'NONE', ( #16905, #7674 ) ) ;
#36291=DIRECTION ( 'NONE',  ( 1.000000000000000000, 0.000000000000000000, 0.000000000000000000 ) ) ;
#36293=DIRECTION ( 'NONE',  ( 1.000000000000000000, 0.000000000000000000, 0.000000000000000000 ) ) ;
#36300=DIRECTION ( 'NONE',  ( 0.000000000000000000, 0.000000000000000000, 1.000000000000000000 ) ) ;
#36303=ADVANCED_FACE ( 'NONE', ( #443 ), #28664, .F. ) ;
#36305=CARTESIAN_POINT ( 'NONE',  ( -8.294006203984645609, 33.46401007850805343, 13.00000000000000178 ) ) ;
#36309=CARTESIAN_POINT ( 'NONE',  ( -6.953812613386785912, 14.77701242934787906, 12.00000000000000000 ) ) ;
#36313=CYLINDRICAL_SURFACE ( 'NONE', #11520, 1.000000000000000888 ) ;
#36318=ORIENTED_EDGE ( 'NONE', *, *, #22787, .T. ) ;
#36326=CARTESIAN_POINT ( 'NONE',  ( 5.330070799514983193, 27.28854476845134513, 12.00000000000000000 ) ) ;
#36332=EDGE_CURVE ( 'NONE', #29063, #38519, #34565, .T. ) ;
#36335=VERTEX_POINT ( 'NONE', #34370 ) ;
#36348=VERTEX_POINT ( 'NONE', #32118 ) ;
#36351=DIRECTION ( 'NONE',  ( 1.000000000000000000, 0.000000000000000000, 0.000000000000000000 ) ) ;
#36354=PRESENTATION_STYLE_ASSIGNMENT (( #23959 ) ) ;
#36363=DIRECTION ( 'NONE',  ( 1.000000000000000000, 0.000000000000000000, 0.000000000000000000 ) ) ;
#36364=DIRECTION ( 'NONE',  ( 0.000000000000000000, 0.000000000000000000, 1.000000000000000000 ) ) ;
#36374=EDGE_CURVE ( 'NONE', #1646, #15234, #10142, .T. ) ;
#36375=ORIENTED_EDGE ( 'NONE', *, *, #21085, .F. ) ;
#36376=VERTEX_POINT ( 'NONE', #14028 ) ;
#36380=AXIS2_PLACEMENT_3D ( 'NONE', #6351, #22191, #19349 ) ;
#36384=CIRCLE ( 'NONE', #3283, 16.00000000000000000 ) ;
#36389=DIRECTION ( 'NONE',  ( 0.000000000000000000, 0.000000000000000000, 1.000000000000000000 ) ) ;
#36396=CARTESIAN_POINT ( 'NONE',  ( -16.00000000000000000, 22.50000000000000711, 11.00000000000000178 ) ) ;
#36400=DIRECTION ( 'NONE',  ( 0.000000000000000000, 0.000000000000000000, 1.000000000000000000 ) ) ;
#36409=DIRECTION ( 'NONE',  ( 0.000000000000000000, 0.000000000000000000, 1.000000000000000000 ) ) ;
#36411=DIRECTION ( 'NONE',  ( 1.000000000000000000, 0.000000000000000000, 0.000000000000000000 ) ) ;
#36412=VERTEX_POINT ( 'NONE', #32731 ) ;
#36421=VECTOR ( 'NONE', #34110, 1000.000000000000000 ) ;
#36422=ORIENTED_EDGE ( 'NONE', *, *, #23609, .F. ) ;
#36434=CARTESIAN_POINT ( 'NONE',  ( -7.935776944912362296, 22.65328985282726393, 13.00000000000000178 ) ) ;
#36438=VERTEX_POINT ( 'NONE', #10585 ) ;
#36448=DIRECTION ( 'NONE',  ( 0.000000000000000000, 0.000000000000000000, 1.000000000000000000 ) ) ;
#36463=ORIENTED_EDGE ( 'NONE', *, *, #16332, .T. ) ;
#36473=EDGE_CURVE ( 'NONE', #10495, #11157, #32933, .T. ) ;
#36496=DIRECTION ( 'NONE',  ( 1.000000000000000000, 0.000000000000000000, 0.000000000000000000 ) ) ;
#36499=EDGE_LOOP ( 'NONE', ( #17519, #20101, #25912, #28783 ) ) ;
#36500=CARTESIAN_POINT ( 'NONE',  ( 9.559505275947156377, 25.28115294937476065, 6.000000000000000000 ) ) ;
#36504=DIRECTION ( 'NONE',  ( 0.000000000000000000, 0.000000000000000000, 1.000000000000000000 ) ) ;
#36505=CARTESIAN_POINT ( 'NONE',  ( -3.853172919594720192, 21.57294901687549427, 12.00000000000000000 ) ) ;
#36515=CARTESIAN_POINT ( 'NONE',  ( 11.77090408390491305, 15.39748370681878775, 12.00000000000000000 ) ) ;
#36520=ORIENTED_EDGE ( 'NONE', *, *, #30997, .T. ) ;
#36531=VECTOR ( 'NONE', #2925, 1000.000000000000000 ) ;
#36533=ORIENTED_EDGE ( 'NONE', *, *, #24916, .F. ) ;
#36535=AXIS2_PLACEMENT_3D ( 'NONE', #5785, #29569, #38915 ) ;
#36536=DIRECTION ( 'NONE',  ( 0.000000000000000000, 0.000000000000000000, 1.000000000000000000 ) ) ;
#36539=CIRCLE ( 'NONE', #26143, 1.000000000000000000 ) ;
#36540=VERTEX_POINT ( 'NONE', #17092 ) ;
#36544=DIRECTION ( 'NONE',  ( 1.000000000000000000, 0.000000000000000000, 0.000000000000000000 ) ) ;
#36546=CIRCLE ( 'NONE', #6034, 1.000000000000000888 ) ;
#36550=FACE_OUTER_BOUND ( 'NONE', #18705, .T. ) ;
#36559=CARTESIAN_POINT ( 'NONE',  ( 1.605696033269625955, 17.55816537872232530, 12.00000000000000000 ) ) ;
#36585=FACE_OUTER_BOUND ( 'NONE', #36773, .T. ) ;
#36588=CIRCLE ( 'NONE', #4766, 1.000000000000000888 ) ;
#36597=DIRECTION ( 'NONE',  ( 1.000000000000000000, 0.000000000000000000, 0.000000000000000000 ) ) ;
#36599=CYLINDRICAL_SURFACE ( 'NONE', #39861, 1.000000000000000000 ) ;
#36604=CARTESIAN_POINT ( 'NONE',  ( 2.587660364795204782, 9.681887955242936883, 13.00000000000000178 ) ) ;
#36618=LINE ( 'NONE', #11832, #28259 ) ;
#36631=PRODUCT_DEFINITION_CONTEXT ( 'detailed design', #6209, 'design' ) ;
#36634=ORIENTED_EDGE ( 'NONE', *, *, #30287, .T. ) ;
#36640=ORIENTED_EDGE ( 'NONE', *, *, #23139, .F. ) ;
#36646=CIRCLE ( 'NONE', #4185, 1.000000000000000888 ) ;
#36651=AXIS2_PLACEMENT_3D ( 'NONE', #8021, #13711, #29561 ) ;
#36654=CYLINDRICAL_SURFACE ( 'NONE', #15274, 1.000000000000000888 ) ;
#36657=LINE ( 'NONE', #8014, #24198 ) ;
#36658=DIRECTION ( 'NONE',  ( 0.000000000000000000, 0.000000000000000000, 1.000000000000000000 ) ) ;
#36663=VERTEX_POINT ( 'NONE', #21129 ) ;
#36666=DIRECTION ( 'NONE',  ( 0.000000000000000000, 0.000000000000000000, 1.000000000000000000 ) ) ;
#36672=CYLINDRICAL_SURFACE ( 'NONE', #21821, 1.000000000000000000 ) ;
#36681=ORIENTED_EDGE ( 'NONE', *, *, #22739, .T. ) ;
#36682=EDGE_CURVE ( 'NONE', #39628, #37016, #14635, .T. ) ;
#36689=ORIENTED_EDGE ( 'NONE', *, *, #30665, .F. ) ;
#36692=VECTOR ( 'NONE', #33220, 1000.000000000000000 ) ;
#36699=ORIENTED_EDGE ( 'NONE', *, *, #20676, .T. ) ;
#36705=DIRECTION ( 'NONE',  ( 0.000000000000000000, 0.000000000000000000, 1.000000000000000000 ) ) ;
#36712=LINE ( 'NONE', #24507, #31345 ) ;
#36716=ORIENTED_EDGE ( 'NONE', *, *, #39192, .F. ) ;
#36728=EDGE_CURVE ( 'NONE', #19765, #6144, #10780, .T. ) ;
#36734=FACE_OUTER_BOUND ( 'NONE', #35039, .T. ) ;
#36736=ORIENTED_EDGE ( 'NONE', *, *, #39922, .F. ) ;
#36745=VECTOR ( 'NONE', #15534, 1000.000000000000000 ) ;
#36748=DIRECTION ( 'NONE',  ( -1.000000000000000000, 0.000000000000000000, 0.000000000000000000 ) ) ;
#36752=DIRECTION ( 'NONE',  ( 1.000000000000000000, 0.000000000000000000, 0.000000000000000000 ) ) ;
#36765=DIRECTION ( 'NONE',  ( 0.000000000000000000, 0.000000000000000000, 1.000000000000000000 ) ) ;
#36773=EDGE_LOOP ( 'NONE', ( #5303, #22474, #16298, #7727 ) ) ;
#36776=CARTESIAN_POINT ( 'NONE',  ( -5.348113209407908464, 9.835177808069893501, 13.00000000000000178 ) ) ;
#36780=FACE_OUTER_BOUND ( 'NONE', #13418, .T. ) ;
#36782=ORIENTED_EDGE ( 'NONE', *, *, #26900, .T. ) ;
#36787=VERTEX_POINT ( 'NONE', #19474 ) ;
#36792=VECTOR ( 'NONE', #31868, 1000.000000000000000 ) ;
#36796=FACE_OUTER_BOUND ( 'NONE', #11365, .T. ) ;
#36799=AXIS2_PLACEMENT_3D ( 'NONE', #14572, #26962, #11923 ) ;
#36830=EDGE_CURVE ( 'NONE', #35424, #880, #18956, .T. ) ;
#36831=AXIS2_PLACEMENT_3D ( 'NONE', #4764, #17968, #36049 ) ;
#36841=DIRECTION ( 'NONE',  ( 1.000000000000000000, 0.000000000000000000, 0.000000000000000000 ) ) ;
#36843=DIRECTION ( 'NONE',  ( 1.000000000000000000, 0.000000000000000000, 0.000000000000000000 ) ) ;
#36844=AXIS2_PLACEMENT_3D ( 'NONE', #6512, #235, #27863 ) ;
#36853=EDGE_CURVE ( 'NONE', #16522, #3856, #31869, .T. ) ;
#36857=CARTESIAN_POINT ( 'NONE',  ( -5.953812613386785912, 14.77701242934787906, 13.00000000000000178 ) ) ;
#36861=VERTEX_POINT ( 'NONE', #13379 ) ;
#36864=DIRECTION ( 'NONE',  ( 0.000000000000000000, 0.000000000000000000, 1.000000000000000000 ) ) ;
#36877=EDGE_LOOP ( 'NONE', ( #6378, #6166 ) ) ;
#36888=AXIS2_PLACEMENT_3D ( 'NONE', #32392, #13077, #1105 ) ;
#36892=CIRCLE ( 'NONE', #10943, 1.000000000000000000 ) ;
#36894=DIRECTION ( 'NONE',  ( 0.000000000000000000, 0.000000000000000000, 1.000000000000000000 ) ) ;
#36895=CIRCLE ( 'NONE', #16118, 0.9999999999999991118 ) ;
#36896=ORIENTED_EDGE ( 'NONE', *, *, #20284, .T. ) ;
#36897=DIRECTION ( 'NONE',  ( 1.000000000000000000, 0.000000000000000000, 0.000000000000000000 ) ) ;
#36899=CARTESIAN_POINT ( 'NONE',  ( -0.6417741116369681809, 11.68927977431952137, 13.00000000000000178 ) ) ;
#36902=DIRECTION ( 'NONE',  ( 1.000000000000000000, 0.000000000000000000, 0.000000000000000000 ) ) ;
#36906=DIRECTION ( 'NONE',  ( 0.000000000000000000, 0.000000000000000000, 1.000000000000000000 ) ) ;
#36910=DIRECTION ( 'NONE',  ( 0.000000000000000000, 0.000000000000000000, 1.000000000000000000 ) ) ;
#36914=CYLINDRICAL_SURFACE ( 'NONE', #30455, 1.000000000000000888 ) ;
#36919=DIRECTION ( 'NONE',  ( 0.000000000000000000, 0.000000000000000000, 1.000000000000000000 ) ) ;
#36921=CIRCLE ( 'NONE', #1892, 1.000000000000000888 ) ;
#36924=FACE_OUTER_BOUND ( 'NONE', #29931, .T. ) ;
#36933=ORIENTED_EDGE ( 'NONE', *, *, #1223, .T. ) ;
#36935=ADVANCED_FACE ( 'NONE', ( #5199 ), #1396, .F. ) ;
#36938=CARTESIAN_POINT ( 'NONE',  ( 8.559505275947156377, 25.28115294937476065, 13.00000000000000178 ) ) ;
#36939=FACE_OUTER_BOUND ( 'NONE', #10407, .T. ) ;
#36942=AXIS2_PLACEMENT_3D ( 'NONE', #17247, #23526, #19468 ) ;
#36946=VERTEX_POINT ( 'NONE', #29977 ) ;
#36947=AXIS2_PLACEMENT_3D ( 'NONE', #30306, #36207, #2478 ) ;
#36952=ORIENTED_EDGE ( 'NONE', *, *, #27799, .F. ) ;
#36966=CARTESIAN_POINT ( 'NONE',  ( -0.9819677022348329842, 30.37627742347970283, 12.00000000000000000 ) ) ;
#36974=AXIS2_PLACEMENT_3D ( 'NONE', #20065, #4005, #22292 ) ;
#36976=ADVANCED_FACE ( 'NONE', ( #22923 ), #30389, .F. ) ;
#36977=CARTESIAN_POINT ( 'NONE',  ( 14.26584437371809777, 27.13525491562438319, 12.00000000000000000 ) ) ;
#36978=CARTESIAN_POINT ( 'NONE',  ( -3.118678732975735279, 7.827785988993307242, 12.00000000000000000 ) ) ;
#36985=ORIENTED_EDGE ( 'NONE', *, *, #10260, .F. ) ;
#36987=DIRECTION ( 'NONE',  ( 0.000000000000000000, 0.000000000000000000, 1.000000000000000000 ) ) ;
#36990=ORIENTED_EDGE ( 'NONE', *, *, #6145, .F. ) ;
#37007=LINE ( 'NONE', #18132, #39763 ) ;
#37008=DIRECTION ( 'NONE',  ( 1.000000000000000000, 0.000000000000000000, 0.000000000000000000 ) ) ;
#37016=VERTEX_POINT ( 'NONE', #25965 ) ;
#37021=ORIENTED_EDGE ( 'NONE', *, *, #29729, .F. ) ;
#37025=VERTEX_POINT ( 'NONE', #7481 ) ;
#37028=DIRECTION ( 'NONE',  ( 0.000000000000000000, 0.000000000000000000, 1.000000000000000000 ) ) ;
#37046=FACE_BOUND ( 'NONE', #4889, .T. ) ;
#37060=FACE_OUTER_BOUND ( 'NONE', #39663, .T. ) ;
#37063=DIRECTION ( 'NONE',  ( 1.000000000000000000, 0.000000000000000000, 0.000000000000000000 ) ) ;
#37069=CIRCLE ( 'NONE', #30607, 1.000000000000000000 ) ;
#37074=ORIENTED_EDGE ( 'NONE', *, *, #26758, .F. ) ;
#37089=CIRCLE ( 'NONE', #4662, 1.000000000000000888 ) ;
#37093=EDGE_LOOP ( 'NONE', ( #11965, #31016, #7110, #9908 ) ) ;
#37100=DIRECTION ( 'NONE',  ( 0.000000000000000000, 0.000000000000000000, 1.000000000000000000 ) ) ;
#37117=DIRECTION ( 'NONE',  ( 1.000000000000000000, 0.000000000000000000, 0.000000000000000000 ) ) ;
#37120=DIRECTION ( 'NONE',  ( 0.000000000000000000, 0.000000000000000000, 1.000000000000000000 ) ) ;
#37129=ORIENTED_EDGE ( 'NONE', *, *, #18958, .T. ) ;
#37138=ORIENTED_EDGE ( 'NONE', *, *, #27423, .T. ) ;
#37141=EDGE_LOOP ( 'NONE', ( #14395, #7781 ) ) ;
#37146=ORIENTED_EDGE ( 'NONE', *, *, #8143, .F. ) ;
#37149=DIRECTION ( 'NONE',  ( 0.000000000000000000, 0.000000000000000000, 1.000000000000000000 ) ) ;
#37151=CARTESIAN_POINT ( 'NONE',  ( 12.64210930126479937, 24.20081211342298744, 12.00000000000000000 ) ) ;
#37163=AXIS2_PLACEMENT_3D ( 'NONE', #34205, #33816, #30566 ) ;
#37195=CYLINDRICAL_SURFACE ( 'NONE', #10349, 1.000000000000000888 ) ;
#37199=DIRECTION ( 'NONE',  ( 1.000000000000000000, 0.000000000000000000, 0.000000000000000000 ) ) ;
#37203=EDGE_CURVE ( 'NONE', #2033, #23095, #34620, .T. ) ;
#37212=CIRCLE ( 'NONE', #22939, 1.000000000000000000 ) ;
#37221=FACE_BOUND ( 'NONE', #27035, .T. ) ;
#37222=CIRCLE ( 'NONE', #24255, 16.00000000000000000 ) ;
#37232=EDGE_LOOP ( 'NONE', ( #826, #356 ) ) ;
#37234=EDGE_LOOP ( 'NONE', ( #9587, #39904, #12186, #38734 ) ) ;
#37239=ORIENTED_EDGE ( 'NONE', *, *, #30649, .T. ) ;
#37243=VECTOR ( 'NONE', #7668, 1000.000000000000000 ) ;
#37247=CARTESIAN_POINT ( 'NONE',  ( -6.330077540933487512, 17.71145523154927659, 12.00000000000000000 ) ) ;
#37248=CARTESIAN_POINT ( 'NONE',  ( 3.835130509701798918, 15.55077355964573904, 6.000000000000000000 ) ) ;
#37250=LINE ( 'NONE', #34404, #31966 ) ;
#37251=CYLINDRICAL_SURFACE ( 'NONE', #8434, 1.000000000000000000 ) ;
#37255=VERTEX_POINT ( 'NONE', #7180 ) ;
#37256=AXIS2_PLACEMENT_3D ( 'NONE', #32860, #5014, #29800 ) ;
#37261=VERTEX_POINT ( 'NONE', #23027 ) ;
#37265=DIRECTION ( 'NONE',  ( 0.000000000000000000, 0.000000000000000000, 1.000000000000000000 ) ) ;
#37278=CARTESIAN_POINT ( 'NONE',  ( 4.100636323082810009, 29.29593658752792962, 13.00000000000000178 ) ) ;
#37279=ORIENTED_EDGE ( 'NONE', *, *, #8863, .F. ) ;
#37285=ORIENTED_EDGE ( 'NONE', *, *, #24651, .F. ) ;
#37295=CARTESIAN_POINT ( 'NONE',  ( 9.788939752379329562, 23.27376113029817617, 6.000000000000000000 ) ) ;
#37305=VERTEX_POINT ( 'NONE', #9838 ) ;
#37317=DIRECTION ( 'NONE',  ( 1.000000000000000000, 0.000000000000000000, 0.000000000000000000 ) ) ;
#37320=CIRCLE ( 'NONE', #21738, 1.000000000000000000 ) ;
#37327=ORIENTED_EDGE ( 'NONE', *, *, #3320, .F. ) ;
#37334=EDGE_CURVE ( 'NONE', #18400, #5055, #33259, .T. ) ;
#37339=ORIENTED_EDGE ( 'NONE', *, *, #31335, .T. ) ;
#37342=CARTESIAN_POINT ( 'NONE',  ( -2.229437847141422679, 24.50739181907689712, 6.000000000000000000 ) ) ;
#37343=CARTESIAN_POINT ( 'NONE',  ( -14.26585111513660031, 17.86474508437623143, 12.00000000000000000 ) ) ;
#37345=VECTOR ( 'NONE', #8993, 1000.000000000000000 ) ;
#37347=ORIENTED_EDGE ( 'NONE', *, *, #13870, .F. ) ;
#37350=DIRECTION ( 'NONE',  ( 0.000000000000000000, 0.000000000000000000, 1.000000000000000000 ) ) ;
#37376=EDGE_LOOP ( 'NONE', ( #10803, #7081, #25390, #31049 ) ) ;
#37379=CIRCLE ( 'NONE', #6228, 1.000000000000000000 ) ;
#37381=EDGE_CURVE ( 'NONE', #11157, #15047, #33283, .T. ) ;
#37382=ORIENTED_EDGE ( 'NONE', *, *, #13287, .T. ) ;
#37396=DIRECTION ( 'NONE',  ( 0.000000000000000000, 0.000000000000000000, 1.000000000000000000 ) ) ;
#37398=EDGE_CURVE ( 'NONE', #12832, #24820, #13147, .T. ) ;
#37401=ADVANCED_FACE ( 'NONE', ( #13275 ), #25667, .F. ) ;
#37406=CARTESIAN_POINT ( 'NONE',  ( -0.3582326297815359162, 33.31072022568110924, 12.00000000000000000 ) ) ;
#37407=VERTEX_POINT ( 'NONE', #695 ) ;
#37412=CARTESIAN_POINT ( 'NONE',  ( -2.587667106213709101, 35.31811204475769728, 6.000000000000000000 ) ) ;
#37417=FACE_BOUND ( 'NONE', #11130, .T. ) ;
#37424=LINE ( 'NONE', #255, #2494 ) ;
#37433=VECTOR ( 'NONE', #13884, 1000.000000000000000 ) ;
#37445=FACE_BOUND ( 'NONE', #8176, .T. ) ;
#37450=CARTESIAN_POINT ( 'NONE',  ( 16.99999999999999645, 22.50000000000000711, 6.000000000000000000 ) ) ;
#37454=AXIS2_PLACEMENT_3D ( 'NONE', #1107, #35637, #35432 ) ;
#37458=EDGE_CURVE ( 'NONE', #4655, #17743, #39071, .T. ) ;
#37466=CARTESIAN_POINT ( 'NONE',  ( -6.082607396026893376, 23.58034083595207875, 12.00000000000000000 ) ) ;
#37469=CIRCLE ( 'NONE', #7596, 1.000000000000000888 ) ;
#37470=ORIENTED_EDGE ( 'NONE', *, *, #2137, .F. ) ;
#37475=ORIENTED_EDGE ( 'NONE', *, *, #13303, .F. ) ;
#37478=CARTESIAN_POINT ( 'NONE',  ( -6.330077540933487512, 17.71145523154927659, 13.00000000000000178 ) ) ;
#37491=EDGE_LOOP ( 'NONE', ( #3278, #17766 ) ) ;
#37507=ORIENTED_EDGE ( 'NONE', *, *, #21575, .T. ) ;
#37515=VERTEX_POINT ( 'NONE', #13891 ) ;
#37516=DIRECTION ( 'NONE',  ( 0.000000000000000000, 0.000000000000000000, 1.000000000000000000 ) ) ;
#37519=AXIS2_PLACEMENT_3D ( 'NONE', #25732, #961, #4203 ) ;
#37520=AXIS2_PLACEMENT_3D ( 'NONE', #3296, #15688, #9400 ) ;
#37527=CIRCLE ( 'NONE', #17447, 1.000000000000000000 ) ;
#37530=VECTOR ( 'NONE', #30886, 1000.000000000000000 ) ;
#37540=ORIENTED_EDGE ( 'NONE', *, *, #3139, .T. ) ;
#37544=CARTESIAN_POINT ( 'NONE',  ( 2.476901250629512941, 26.36149378532653031, 12.00000000000000000 ) ) ;
#37546=CIRCLE ( 'NONE', #2524, 1.000000000000000000 ) ;
#37552=CARTESIAN_POINT ( 'NONE',  ( 13.39463915635820790, 18.33192650902018883, 13.00000000000000178 ) ) ;
#37553=DIRECTION ( 'NONE',  ( 0.000000000000000000, 0.000000000000000000, 1.000000000000000000 ) ) ;
#37572=EDGE_LOOP ( 'NONE', ( #20760, #33143 ) ) ;
#37576=AXIS2_PLACEMENT_3D ( 'NONE', #10271, #39052, #732 ) ;
#37579=ORIENTED_EDGE ( 'NONE', *, *, #21941, .F. ) ;
#37584=VECTOR ( 'NONE', #8321, 1000.000000000000000 ) ;
#37588=EDGE_CURVE ( 'NONE', #15880, #25686, #9913, .T. ) ;
#37590=EDGE_LOOP ( 'NONE', ( #39461, #1442 ) ) ;
#37592=EDGE_CURVE ( 'NONE', #31950, #5290, #17706, .T. ) ;
#37597=DIRECTION ( 'NONE',  ( 0.000000000000000000, 0.000000000000000000, 1.000000000000000000 ) ) ;
#37612=VECTOR ( 'NONE', #22489, 1000.000000000000000 ) ;
#37618=DIRECTION ( 'NONE',  ( 0.000000000000000000, 0.000000000000000000, 1.000000000000000000 ) ) ;
#37620=EDGE_LOOP ( 'NONE', ( #8637, #37627 ) ) ;
#37623=FACE_BOUND ( 'NONE', #34217, .T. ) ;
#37627=ORIENTED_EDGE ( 'NONE', *, *, #618, .F. ) ;
#37629=CARTESIAN_POINT ( 'NONE',  ( -1.358232629781535916, 33.31072022568110924, 13.00000000000000178 ) ) ;
#37636=AXIS2_PLACEMENT_3D ( 'NONE', #24261, #14921, #11872 ) ;
#37646=FACE_BOUND ( 'NONE', #16491, .T. ) ;
#37680=AXIS2_PLACEMENT_3D ( 'NONE', #11670, #12260, #2329 ) ;
#37687=EDGE_CURVE ( 'NONE', #5736, #17675, #1476, .T. ) ;
#37696=CARTESIAN_POINT ( 'NONE',  ( 14.26584437371809777, 27.13525491562438319, 6.000000000000000000 ) ) ;
#37707=CARTESIAN_POINT ( 'NONE',  ( -4.118678732975735279, 7.827785988993307242, 12.00000000000000000 ) ) ;
#37711=DIRECTION ( 'NONE',  ( 1.000000000000000000, 0.000000000000000000, 0.000000000000000000 ) ) ;
#37716=DIRECTION ( 'NONE',  ( 0.000000000000000000, 0.000000000000000000, 1.000000000000000000 ) ) ;
#37739=ORIENTED_EDGE ( 'NONE', *, *, #34847, .T. ) ;
#37740=VERTEX_POINT ( 'NONE', #16087 ) ;
#37744=ORIENTED_EDGE ( 'NONE', *, *, #35816, .F. ) ;
#37748=AXIS2_PLACEMENT_3D ( 'NONE', #39019, #23782, #11197 ) ;
#37756=CARTESIAN_POINT ( 'NONE',  ( -12.39464589777671044, 26.66807349098043289, 12.00000000000000000 ) ) ;
#37762=DIRECTION ( 'NONE',  ( 0.000000000000000000, 0.000000000000000000, 1.000000000000000000 ) ) ;
#37788=DIRECTION ( 'NONE',  ( 0.000000000000000000, 0.000000000000000000, 1.000000000000000000 ) ) ;
#37802=ORIENTED_EDGE ( 'NONE', *, *, #26513, .F. ) ;
#37808=DIRECTION ( 'NONE',  ( 1.000000000000000000, 0.000000000000000000, 0.000000000000000000 ) ) ;
#37809=ADVANCED_FACE ( 'NONE', ( #19528 ), #9988, .F. ) ;
#37813=LINE ( 'NONE', #38416, #16549 ) ;
#37814=FACE_BOUND ( 'NONE', #20999, .T. ) ;
#37821=ORIENTED_EDGE ( 'NONE', *, *, #6746, .T. ) ;
#37828=ORIENTED_EDGE ( 'NONE', *, *, #38418, .F. ) ;
#37829=CIRCLE ( 'NONE', #4753, 1.000000000000000000 ) ;
#37834=FACE_OUTER_BOUND ( 'NONE', #26072, .T. ) ;
#37836=CIRCLE ( 'NONE', #23584, 1.000000000000000888 ) ;
#37837=FACE_BOUND ( 'NONE', #39234, .T. ) ;
#37842=EDGE_CURVE ( 'NONE', #634, #29140, #18994, .T. ) ;
#37853=DIRECTION ( 'NONE',  ( 0.000000000000000000, 0.000000000000000000, 1.000000000000000000 ) ) ;
#37854=ORIENTED_EDGE ( 'NONE', *, *, #28729, .F. ) ;
#37856=DIRECTION ( 'NONE',  ( 0.000000000000000000, 0.000000000000000000, 1.000000000000000000 ) ) ;
#37858=CARTESIAN_POINT ( 'NONE',  ( -9.541476348891238857, 27.59512447410525127, 6.000000000000000000 ) ) ;
#37867=DIRECTION ( 'NONE',  ( 1.000000000000000000, 0.000000000000000000, 0.000000000000000000 ) ) ;
#37875=ORIENTED_EDGE ( 'NONE', *, *, #15094, .F. ) ;
#37878=CIRCLE ( 'NONE', #27500, 1.000000000000000888 ) ;
#37887=ORIENTED_EDGE ( 'NONE', *, *, #29990, .T. ) ;
#37888=FACE_OUTER_BOUND ( 'NONE', #11621, .T. ) ;
#37893=EDGE_CURVE ( 'NONE', #15410, #761, #15108, .T. ) ;
#37904=FACE_OUTER_BOUND ( 'NONE', #30095, .T. ) ;
#37913=AXIS2_PLACEMENT_3D ( 'NONE', #5477, #8734, #24762 ) ;
#37914=ADVANCED_FACE ( 'NONE', ( #17506 ), #16899, .F. ) ;
#37924=AXIS2_PLACEMENT_3D ( 'NONE', #8370, #23805, #33166 ) ;
#37935=ORIENTED_EDGE ( 'NONE', *, *, #18466, .T. ) ;
#37943=CARTESIAN_POINT ( 'NONE',  ( -4.724378136954611840, 12.76962061027129458, 12.00000000000000000 ) ) ;
#37944=CIRCLE ( 'NONE', #2918, 1.000000000000000000 ) ;
#37945=CARTESIAN_POINT ( 'NONE',  ( -3.835137251120299684, 29.44922644035488446, 13.00000000000000178 ) ) ;
#37946=DIRECTION ( 'NONE',  ( 1.000000000000000000, 0.000000000000000000, 0.000000000000000000 ) ) ;
#37947=ADVANCED_FACE ( 'NONE', ( #13834 ), #23387, .F. ) ;
#37951=AXIS2_PLACEMENT_3D ( 'NONE', #8063, #29805, #7862 ) ;
#37968=ORIENTED_EDGE ( 'NONE', *, *, #1665, .F. ) ;
#37976=VERTEX_POINT ( 'NONE', #14238 ) ;
#37979=DIRECTION ( 'NONE',  ( 0.000000000000000000, 0.000000000000000000, 1.000000000000000000 ) ) ;
#37980=ORIENTED_EDGE ( 'NONE', *, *, #25561, .F. ) ;
#37988=DIRECTION ( 'NONE',  ( 1.000000000000000000, 0.000000000000000000, 0.000000000000000000 ) ) ;
#37989=DIRECTION ( 'NONE',  ( 0.000000000000000000, 0.000000000000000000, 1.000000000000000000 ) ) ;
#37992=VERTEX_POINT ( 'NONE', #4898 ) ;
#38002=CIRCLE ( 'NONE', #17263, 1.000000000000000000 ) ;
#38015=FACE_BOUND ( 'NONE', #23288, .T. ) ;
#38024=DIRECTION ( 'NONE',  ( 0.000000000000000000, 0.000000000000000000, 1.000000000000000000 ) ) ;
#38037=EDGE_CURVE ( 'NONE', #1841, #8501, #14379, .T. ) ;
#38038=AXIS2_PLACEMENT_3D ( 'NONE', #24873, #495, #25072 ) ;
#38040=EDGE_CURVE ( 'NONE', #4736, #22293, #30626, .T. ) ;
#38041=FACE_BOUND ( 'NONE', #8235, .T. ) ;
#38047=ORIENTED_EDGE ( 'NONE', *, *, #9565, .T. ) ;
#38053=ORIENTED_EDGE ( 'NONE', *, *, #18908, .T. ) ;
#38058=CARTESIAN_POINT ( 'NONE',  ( -7.312041872459064784, 25.58773265502866678, 6.000000000000000000 ) ) ;
#38081=AXIS2_PLACEMENT_3D ( 'NONE', #30739, #54, #9401 ) ;
#38084=CARTESIAN_POINT ( 'NONE',  ( 12.01837422881150275, 21.26636931122159169, 6.000000000000000000 ) ) ;
#38085=CARTESIAN_POINT ( 'NONE',  ( -9.541476348891238857, 27.59512447410525127, 6.000000000000000000 ) ) ;
#38092=DIRECTION ( 'NONE',  ( 1.000000000000000000, 0.000000000000000000, 0.000000000000000000 ) ) ;
#38121=AXIS2_PLACEMENT_3D ( 'NONE', #29285, #25827, #10397 ) ;
#38128=EDGE_CURVE ( 'NONE', #30397, #4798, #2651, .T. ) ;
#38134=DIRECTION ( 'NONE',  ( 1.000000000000000000, 0.000000000000000000, 0.000000000000000000 ) ) ;
#38135=DIRECTION ( 'NONE',  ( 0.000000000000000000, 0.000000000000000000, 1.000000000000000000 ) ) ;
#38136=DIRECTION ( 'NONE',  ( 1.000000000000000000, 0.000000000000000000, 0.000000000000000000 ) ) ;
#38141=AXIS2_PLACEMENT_3D ( 'NONE', #33, #16271, #436 ) ;
#38145=VECTOR ( 'NONE', #1610, 1000.000000000000000 ) ;
#38158=DIRECTION ( 'NONE',  ( 0.000000000000000000, 0.000000000000000000, 1.000000000000000000 ) ) ;
#38160=VECTOR ( 'NONE', #30689, 1000.000000000000000 ) ;
#38167=DIRECTION ( 'NONE',  ( 0.000000000000000000, 0.000000000000000000, 1.000000000000000000 ) ) ;
#38171=DIRECTION ( 'NONE',  ( 1.000000000000000000, 0.000000000000000000, 0.000000000000000000 ) ) ;
#38198=DIRECTION ( 'NONE',  ( 1.000000000000000000, 0.000000000000000000, 0.000000000000000000 ) ) ;
#38202=CARTESIAN_POINT ( 'NONE',  ( 12.01837422881150275, 21.26636931122159169, 12.00000000000000000 ) ) ;
#38203=CARTESIAN_POINT ( 'NONE',  ( 2.835130509701798918, 15.55077355964573904, 6.000000000000000000 ) ) ;
#38207=DIRECTION ( 'NONE',  ( 0.000000000000000000, 0.000000000000000000, 1.000000000000000000 ) ) ;
#38209=CIRCLE ( 'NONE', #14869, 1.000000000000000000 ) ;
#38212=AXIS2_PLACEMENT_3D ( 'NONE', #39154, #2193, #2392 ) ;
#38221=FACE_BOUND ( 'NONE', #15439, .T. ) ;
#38239=DIRECTION ( 'NONE',  ( 1.000000000000000000, 0.000000000000000000, 0.000000000000000000 ) ) ;
#38242=CARTESIAN_POINT ( 'NONE',  ( 5.724371395536106633, 32.23037938972932892, 6.000000000000000000 ) ) ;
#38246=FACE_BOUND ( 'NONE', #34866, .T. ) ;
#38250=CARTESIAN_POINT ( 'NONE',  ( 6.953805871968278929, 30.22298757065274444, 12.00000000000000000 ) ) ;
#38256=CYLINDRICAL_SURFACE ( 'NONE', #13347, 1.000000000000000888 ) ;
#38261=CARTESIAN_POINT ( 'NONE',  ( 13.64210930126480115, 24.20081211342298744, 12.00000000000000000 ) ) ;
#38271=CARTESIAN_POINT ( 'NONE',  ( -4.100643064501314328, 15.70406341247269211, 13.00000000000000178 ) ) ;
#38290=FACE_OUTER_BOUND ( 'NONE', #27480, .T. ) ;
#38293=FACE_OUTER_BOUND ( 'NONE', #8799, .T. ) ;
#38302=CYLINDRICAL_SURFACE ( 'NONE', #28958, 1.000000000000000000 ) ;
#38311=FACE_OUTER_BOUND ( 'NONE', #12603, .T. ) ;
#38318=ORIENTED_EDGE ( 'NONE', *, *, #20464, .F. ) ;
#38328=ORIENTED_EDGE ( 'NONE', *, *, #34976, .F. ) ;
#38329=CARTESIAN_POINT ( 'NONE',  ( 4.348106467989403257, 35.16482219193073178, 12.00000000000000000 ) ) ;
#38334=EDGE_CURVE ( 'NONE', #30382, #26791, #17648, .T. ) ;
#38337=DIRECTION ( 'NONE',  ( 0.000000000000000000, 0.000000000000000000, 1.000000000000000000 ) ) ;
#38338=FACE_OUTER_BOUND ( 'NONE', #11682, .T. ) ;
#38340=EDGE_LOOP ( 'NONE', ( #3582, #27177, #30998, #36952 ) ) ;
#38342=AXIS2_PLACEMENT_3D ( 'NONE', #22589, #31740, #18949 ) ;
#38349=DIRECTION ( 'NONE',  ( 1.000000000000000000, 0.000000000000000000, 0.000000000000000000 ) ) ;
#38350=ORIENTED_EDGE ( 'NONE', *, *, #38920, .T. ) ;
#38352=DIRECTION ( 'NONE',  ( 1.000000000000000000, 0.000000000000000000, 0.000000000000000000 ) ) ;
#38359=EDGE_CURVE ( 'NONE', #10298, #333, #15675, .T. ) ;
#38367=ORIENTED_EDGE ( 'NONE', *, *, #34725, .F. ) ;
#38371=AXIS2_PLACEMENT_3D ( 'NONE', #18717, #37396, #28448 ) ;
#38380=ORIENTED_EDGE ( 'NONE', *, *, #35406, .F. ) ;
#38382=EDGE_LOOP ( 'NONE', ( #19227, #5155, #4569, #36422 ) ) ;
#38387=CARTESIAN_POINT ( 'NONE',  ( 5.440829913680675034, 10.60893893836775348, 12.00000000000000000 ) ) ;
#38393=CARTESIAN_POINT ( 'NONE',  ( 2.853166178176219425, 23.42705098312512746, 13.00000000000000178 ) ) ;
#38394=DIRECTION ( 'NONE',  ( 1.000000000000000000, 0.000000000000000000, 0.000000000000000000 ) ) ;
#38398=ORIENTED_EDGE ( 'NONE', *, *, #15466, .F. ) ;
#38416=CARTESIAN_POINT ( 'NONE',  ( -5.724378136954611840, 12.76962061027129458, 6.000000000000000000 ) ) ;
#38417=DIRECTION ( 'NONE',  ( 0.000000000000000000, 0.000000000000000000, 1.000000000000000000 ) ) ;
#38418=EDGE_CURVE ( 'NONE', #22962, #12988, #37089, .T. ) ;
#38437=EDGE_CURVE ( 'NONE', #27813, #708, #25409, .T. ) ;
#38440=CARTESIAN_POINT ( 'NONE',  ( 9.293999462566146619, 11.53598992149257008, 12.00000000000000000 ) ) ;
#38443=CARTESIAN_POINT ( 'NONE',  ( 6.688300058587269170, 16.47782454277055564, 6.000000000000000000 ) ) ;
#38453=VERTEX_POINT ( 'NONE', #7891 ) ;
#38456=EDGE_CURVE ( 'NONE', #32704, #35813, #28002, .T. ) ;
#38459=EDGE_LOOP ( 'NONE', ( #3383, #15197 ) ) ;
#38461=DIRECTION ( 'NONE',  ( 1.000000000000000000, 0.000000000000000000, 0.000000000000000000 ) ) ;
#38471=DIRECTION ( 'NONE',  ( 0.000000000000000000, 0.000000000000000000, 1.000000000000000000 ) ) ;
#38486=DIRECTION ( 'NONE',  ( 0.000000000000000000, 0.000000000000000000, 1.000000000000000000 ) ) ;
#38492=ORIENTED_EDGE ( 'NONE', *, *, #2669, .T. ) ;
#38495=CARTESIAN_POINT ( 'NONE',  ( -0.3762682982559537037, 25.43444280220171194, 12.00000000000000000 ) ) ;
#38498=CARTESIAN_POINT ( 'NONE',  ( -10.14717575287011542, 32.53695909538323860, 12.00000000000000000 ) ) ;
#38519=VERTEX_POINT ( 'NONE', #20096 ) ;
#38521=DIRECTION ( 'NONE',  ( 0.000000000000000000, 0.000000000000000000, 1.000000000000000000 ) ) ;
#38524=ORIENTED_EDGE ( 'NONE', *, *, #26265, .T. ) ;
#38530=DIRECTION ( 'NONE',  ( 0.000000000000000000, 0.000000000000000000, 1.000000000000000000 ) ) ;
#38534=AXIS2_PLACEMENT_3D ( 'NONE', #25938, #38337, #1775 ) ;
#38545=CARTESIAN_POINT ( 'NONE',  ( -3.229437847141423124, 24.50739181907689712, 13.00000000000000178 ) ) ;
#38550=DIRECTION ( 'NONE',  ( 0.000000000000000000, 0.000000000000000000, 1.000000000000000000 ) ) ;
#38553=ORIENTED_EDGE ( 'NONE', *, *, #40144, .F. ) ;
#38567=EDGE_CURVE ( 'NONE', #1690, #17473, #12455, .T. ) ;
#38568=DIRECTION ( 'NONE',  ( 0.000000000000000000, 0.000000000000000000, 1.000000000000000000 ) ) ;
#38576=EDGE_LOOP ( 'NONE', ( #4505, #35835 ) ) ;
#38583=CIRCLE ( 'NONE', #33417, 1.000000000000000000 ) ;
#38586=DIRECTION ( 'NONE',  ( 1.000000000000000000, 0.000000000000000000, 0.000000000000000000 ) ) ;
#38589=EDGE_CURVE ( 'NONE', #25338, #20584, #8569, .T. ) ;
#38591=CIRCLE ( 'NONE', #35377, 1.000000000000000888 ) ;
#38596=CARTESIAN_POINT ( 'NONE',  ( -0.6237384431625470071, 19.56555719779890978, 12.00000000000000000 ) ) ;
#38600=CARTESIAN_POINT ( 'NONE',  ( -5.440836655099179353, 34.39106106163288246, 12.00000000000000000 ) ) ;
#38604=CARTESIAN_POINT ( 'NONE',  ( -3.494943660522439099, 10.76222879119470832, 6.000000000000000000 ) ) ;
#38611=DIRECTION ( 'NONE',  ( 1.000000000000000000, 0.000000000000000000, 0.000000000000000000 ) ) ;
#38613=EDGE_LOOP ( 'NONE', ( #28079, #6513, #31836, #33024 ) ) ;
#38617=CARTESIAN_POINT ( 'NONE',  ( 6.577540944421576441, 33.15743037285414374, 12.00000000000000000 ) ) ;
#38618=FACE_BOUND ( 'NONE', #31478, .T. ) ;
#38621=AXIS2_PLACEMENT_3D ( 'NONE', #35981, #11989, #24381 ) ;
#38631=CARTESIAN_POINT ( 'NONE',  ( 0.6237317017440463518, 25.43444280220171194, 12.00000000000000000 ) ) ;
#38632=ORIENTED_EDGE ( 'NONE', *, *, #7249, .T. ) ;
#38643=ORIENTED_EDGE ( 'NONE', *, *, #30284, .F. ) ;
#38653=LINE ( 'NONE', #34060, #273 ) ;
#38654=DIRECTION ( 'NONE',  ( 0.000000000000000000, 0.000000000000000000, 1.000000000000000000 ) ) ;
#38655=ORIENTED_EDGE ( 'NONE', *, *, #23441, .T. ) ;
#38660=LINE ( 'NONE', #29519, #2322 ) ;
#38671=ORIENTED_EDGE ( 'NONE', *, *, #2271, .T. ) ;
#38676=VERTEX_POINT ( 'NONE', #20898 ) ;
#38681=ORIENTED_EDGE ( 'NONE', *, *, #2425, .T. ) ;
#38687=AXIS2_PLACEMENT_3D ( 'NONE', #8687, #18630, #15176 ) ;
#38692=DIRECTION ( 'NONE',  ( 1.000000000000000000, 0.000000000000000000, 0.000000000000000000 ) ) ;
#38693=CARTESIAN_POINT ( 'NONE',  ( 6.935770203493858865, 22.34671014717335780, 12.00000000000000000 ) ) ;
#38701=DIRECTION ( 'NONE',  ( 1.000000000000000000, 0.000000000000000000, 0.000000000000000000 ) ) ;
#38706=FILL_AREA_STYLE ('',( #10469 ) ) ;
#38714=ORIENTED_EDGE ( 'NONE', *, *, #9410, .F. ) ;
#38734=ORIENTED_EDGE ( 'NONE', *, *, #25648, .F. ) ;
#38740=VECTOR ( 'NONE', #27536, 1000.000000000000000 ) ;
#38742=ORIENTED_EDGE ( 'NONE', *, *, #15425, .F. ) ;
#38744=CYLINDRICAL_SURFACE ( 'NONE', #2650, 1.000000000000000000 ) ;
#38745=CARTESIAN_POINT ( 'NONE',  ( 9.183240348400453001, 28.21559575157615996, 12.00000000000000000 ) ) ;
#38754=DIRECTION ( 'NONE',  ( -0.000000000000000000, -0.000000000000000000, -1.000000000000000000 ) ) ;
#38757=DIRECTION ( 'NONE',  ( 0.000000000000000000, 0.000000000000000000, 1.000000000000000000 ) ) ;
#38758=DIRECTION ( 'NONE',  ( 1.000000000000000000, 0.000000000000000000, 0.000000000000000000 ) ) ;
#38760=CARTESIAN_POINT ( 'NONE',  ( -4.082607396026893376, 23.58034083595207875, 13.00000000000000178 ) ) ;
#38765=AXIS2_PLACEMENT_3D ( 'NONE', #8294, #8495, #11746 ) ;
#38770=FACE_OUTER_BOUND ( 'NONE', #26421, .T. ) ;
#38774=AXIS2_PLACEMENT_3D ( 'NONE', #21008, #32606, #33014 ) ;
#38776=AXIS2_PLACEMENT_3D ( 'NONE', #20855, #23490, #35885 ) ;
#38777=DIRECTION ( 'NONE',  ( 0.000000000000000000, 0.000000000000000000, 1.000000000000000000 ) ) ;
#38781=EDGE_CURVE ( 'NONE', #880, #35978, #14407, .T. ) ;
#38784=EDGE_LOOP ( 'NONE', ( #39383, #21660 ) ) ;
#38787=DIRECTION ( 'NONE',  ( 1.000000000000000000, 0.000000000000000000, 0.000000000000000000 ) ) ;
#38790=DIRECTION ( 'NONE',  ( 1.000000000000000000, 0.000000000000000000, 0.000000000000000000 ) ) ;
#38799=EDGE_CURVE ( 'NONE', #34302, #11394, #34532, .T. ) ;
#38816=ORIENTED_EDGE ( 'NONE', *, *, #38437, .F. ) ;
#38821=AXIS2_PLACEMENT_3D ( 'NONE', #15200, #36536, #21691 ) ;
#38831=CIRCLE ( 'NONE', #31690, 1.000000000000000000 ) ;
#38837=CIRCLE ( 'NONE', #31593, 1.000000000000000888 ) ;
#38839=ORIENTED_EDGE ( 'NONE', *, *, #10616, .F. ) ;
#38842=DIRECTION ( 'NONE',  ( 0.000000000000000000, 0.000000000000000000, 1.000000000000000000 ) ) ;
#38847=DIRECTION ( 'NONE',  ( 0.000000000000000000, 0.000000000000000000, 1.000000000000000000 ) ) ;
#38851=VECTOR ( 'NONE', #13031, 1000.000000000000000 ) ;
#38856=AXIS2_PLACEMENT_3D ( 'NONE', #7955, #8368, #36597 ) ;
#38857=DIRECTION ( 'NONE',  ( 1.000000000000000000, 0.000000000000000000, 0.000000000000000000 ) ) ;
#38858=FACE_OUTER_BOUND ( 'NONE', #27048, .T. ) ;
#38859=ORIENTED_EDGE ( 'NONE', *, *, #18562, .F. ) ;
#38868=EDGE_LOOP ( 'NONE', ( #23142, #17664 ) ) ;
#38870=CARTESIAN_POINT ( 'NONE',  ( -3.118678732975735279, 7.827785988993307242, 13.00000000000000178 ) ) ;
#38879=EDGE_LOOP ( 'NONE', ( #25972, #7745 ) ) ;
#38897=CARTESIAN_POINT ( 'NONE',  ( 12.64210930126479937, 24.20081211342298744, 6.000000000000000000 ) ) ;
#38899=ORIENTED_EDGE ( 'NONE', *, *, #14132, .T. ) ;
#38902=FACE_OUTER_BOUND ( 'NONE', #8029, .T. ) ;
#38904=LINE ( 'NONE', #11081, #16438 ) ;
#38915=DIRECTION ( 'NONE',  ( 1.000000000000000000, 0.000000000000000000, 0.000000000000000000 ) ) ;
#38916=ORIENTED_EDGE ( 'NONE', *, *, #26758, .T. ) ;
#38920=EDGE_CURVE ( 'NONE', #7138, #38453, #23509, .T. ) ;
#38925=ORIENTED_EDGE ( 'NONE', *, *, #5517, .T. ) ;
#38928=CARTESIAN_POINT ( 'NONE',  ( -12.14717575287011719, 32.53695909538323860, 12.00000000000000000 ) ) ;
#38944=CYLINDRICAL_SURFACE ( 'NONE', #9998, 1.000000000000000000 ) ;
#38945=EDGE_CURVE ( 'NONE', #19314, #2033, #2752, .T. ) ;
#38950=DIRECTION ( 'NONE',  ( 0.000000000000000000, 0.000000000000000000, 1.000000000000000000 ) ) ;
#38961=LINE ( 'NONE', #35720, #16620 ) ;
#38977=ORIENTED_EDGE ( 'NONE', *, *, #27527, .T. ) ;
#38978=CARTESIAN_POINT ( 'NONE',  ( 2.494936919103933448, 34.23777120880591696, 13.00000000000000178 ) ) ;
#38979=VERTEX_POINT ( 'NONE', #25831 ) ;
#38980=DIRECTION ( 'NONE',  ( 1.000000000000000000, 0.000000000000000000, 0.000000000000000000 ) ) ;
#38981=DIRECTION ( 'NONE',  ( 0.000000000000000000, 0.000000000000000000, 1.000000000000000000 ) ) ;
#38995=DIRECTION ( 'NONE',  ( 0.000000000000000000, 0.000000000000000000, 1.000000000000000000 ) ) ;
#38996=CARTESIAN_POINT ( 'NONE',  ( 5.440829913680675034, 10.60893893836775348, 13.00000000000000178 ) ) ;
#39017=FACE_BOUND ( 'NONE', #25829, .T. ) ;
#39019=CARTESIAN_POINT ( 'NONE',  ( 0.000000000000000000, 22.50000000000000355, 13.00000000000000178 ) ) ;
#39020=ORIENTED_EDGE ( 'NONE', *, *, #35569, .T. ) ;
#39023=CARTESIAN_POINT ( 'NONE',  ( 11.14716901145161643, 12.46304090461738667, 13.00000000000000178 ) ) ;
#39025=DIRECTION ( 'NONE',  ( 1.000000000000000000, 0.000000000000000000, 0.000000000000000000 ) ) ;
#39026=EDGE_LOOP ( 'NONE', ( #21377, #17516 ) ) ;
#39028=CYLINDRICAL_SURFACE ( 'NONE', #27421, 1.000000000000000888 ) ;
#39035=CARTESIAN_POINT ( 'NONE',  ( 7.935770203493858865, 22.34671014717335780, 12.00000000000000000 ) ) ;
#39039=VERTEX_POINT ( 'NONE', #25626 ) ;
#39042=LINE ( 'NONE', #14459, #17605 ) ;
#39048=EDGE_CURVE ( 'NONE', #19095, #36376, #31910, .T. ) ;
#39050=DIRECTION ( 'NONE',  ( 1.000000000000000000, 0.000000000000000000, 0.000000000000000000 ) ) ;
#39052=DIRECTION ( 'NONE',  ( 0.000000000000000000, 0.000000000000000000, 1.000000000000000000 ) ) ;
#39055=EDGE_LOOP ( 'NONE', ( #29314, #40071, #21839, #90 ) ) ;
#39067=ORIENTED_EDGE ( 'NONE', *, *, #28496, .T. ) ;
#39071=LINE ( 'NONE', #11249, #4722 ) ;
#39091=CARTESIAN_POINT ( 'NONE',  ( 0.2655024426717602637, 36.24516302788250499, 12.00000000000000000 ) ) ;
#39095=CARTESIAN_POINT ( 'NONE',  ( 10.80697542085375140, 31.15003855377755571, 6.000000000000000000 ) ) ;
#39096=DIRECTION ( 'NONE',  ( 0.000000000000000000, 0.000000000000000000, 1.000000000000000000 ) ) ;
#39105=CIRCLE ( 'NONE', #25468, 1.000000000000000000 ) ;
#39106=DIRECTION ( 'NONE',  ( 0.000000000000000000, 0.000000000000000000, 1.000000000000000000 ) ) ;
#39122=CARTESIAN_POINT ( 'NONE',  ( -15.26585111513660209, 17.86474508437623143, 12.00000000000000000 ) ) ;
#39133=AXIS2_PLACEMENT_3D ( 'NONE', #13949, #11513, #14152 ) ;
#39148=LINE ( 'NONE', #11127, #39827 ) ;
#39154=CARTESIAN_POINT ( 'NONE',  ( 0.000000000000000000, 22.50000000000000355, 11.00000000000000178 ) ) ;
#39155=AXIS2_PLACEMENT_3D ( 'NONE', #3709, #31943, #10011 ) ;
#39171=EDGE_CURVE ( 'NONE', #21822, #26584, #20298, .T. ) ;
#39174=AXIS2_PLACEMENT_3D ( 'NONE', #8917, #33715, #33113 ) ;
#39183=CIRCLE ( 'NONE', #11931, 1.000000000000000888 ) ;
#39190=ADVANCED_FACE ( 'NONE', ( #11206 ), #39028, .F. ) ;
#39191=VECTOR ( 'NONE', #21856, 1000.000000000000000 ) ;
#39192=EDGE_CURVE ( 'NONE', #24994, #19934, #39105, .T. ) ;
#39196=CARTESIAN_POINT ( 'NONE',  ( 0.6417673702184640838, 33.31072022568110924, 13.00000000000000178 ) ) ;
#39218=CARTESIAN_POINT ( 'NONE',  ( 3.724371395536106188, 32.23037938972932892, 13.00000000000000178 ) ) ;
#39227=ORIENTED_EDGE ( 'NONE', *, *, #8892, .T. ) ;
#39234=EDGE_LOOP ( 'NONE', ( #25533, #38350 ) ) ;
#39242=FACE_OUTER_BOUND ( 'NONE', #30484, .T. ) ;
#39243=DIRECTION ( 'NONE',  ( 1.000000000000000000, 0.000000000000000000, 0.000000000000000000 ) ) ;
#39254=ORIENTED_EDGE ( 'NONE', *, *, #27474, .F. ) ;
#39272=ORIENTED_EDGE ( 'NONE', *, *, #4583, .T. ) ;
#39278=ORIENTED_EDGE ( 'NONE', *, *, #15364, .T. ) ;
#39284=EDGE_CURVE ( 'NONE', #342, #25818, #16372, .T. ) ;
#39285=VECTOR ( 'NONE', #2145, 1000.000000000000000 ) ;
#39288=AXIS2_PLACEMENT_3D ( 'NONE', #7404, #31994, #25692 ) ;
#39292=CARTESIAN_POINT ( 'NONE',  ( 7.312035131040564906, 19.41226734497195849, 12.00000000000000000 ) ) ;
#39318=AXIS2_PLACEMENT_3D ( 'NONE', #12332, #37120, #37317 ) ;
#39326=ADVANCED_FACE ( 'NONE', ( #36585 ), #15649, .F. ) ;
#39329=CARTESIAN_POINT ( 'NONE',  ( 0.000000000000000000, 22.50000000000000355, 12.00000000000000000 ) ) ;
#39337=CARTESIAN_POINT ( 'NONE',  ( -5.688306800005769048, 28.52217545723006609, 13.00000000000000178 ) ) ;
#39340=CARTESIAN_POINT ( 'NONE',  ( -14.64211604268330902, 20.79918788657763429, 12.00000000000000000 ) ) ;
#39346=AXIS2_PLACEMENT_3D ( 'NONE', #37858, #31563, #12678 ) ;
#39350=DIRECTION ( 'NONE',  ( 1.000000000000000000, 0.000000000000000000, 0.000000000000000000 ) ) ;
#39363=LINE ( 'NONE', #39760, #22426 ) ;
#39380=VERTEX_POINT ( 'NONE', #18896 ) ;
#39383=ORIENTED_EDGE ( 'NONE', *, *, #9410, .T. ) ;
#39387=CARTESIAN_POINT ( 'NONE',  ( -4.211402178667006169, 32.38366924255629442, 6.000000000000000000 ) ) ;
#39397=ORIENTED_EDGE ( 'NONE', *, *, #18809, .T. ) ;
#39399=CARTESIAN_POINT ( 'NONE',  ( 0.3582258883630317636, 11.68927977431952137, 13.00000000000000178 ) ) ;
#39417=EDGE_LOOP ( 'NONE', ( #36027, #3592, #21105, #40054, #22613, #28659 ) ) ;
#39421=CARTESIAN_POINT ( 'NONE',  ( -3.587667106213709101, 35.31811204475769728, 6.000000000000000000 ) ) ;
#39430=ADVANCED_FACE ( 'NONE', ( #6293 ), #24189, .F. ) ;
#39434=AXIS2_PLACEMENT_3D ( 'NONE', #1619, #27002, #38787 ) ;
#39438=CIRCLE ( 'NONE', #38776, 1.000000000000000000 ) ;
#39439=CARTESIAN_POINT ( 'NONE',  ( 8.559505275947156377, 25.28115294937476065, 13.00000000000000178 ) ) ;
#39442=CARTESIAN_POINT ( 'NONE',  ( 11.41267482483262619, 26.20820393249957192, 6.000000000000000000 ) ) ;
#39446=DIRECTION ( 'NONE',  ( 0.000000000000000000, 0.000000000000000000, 1.000000000000000000 ) ) ;
#39450=DIRECTION ( 'NONE',  ( 0.000000000000000000, 0.000000000000000000, 1.000000000000000000 ) ) ;
#39454=CIRCLE ( 'NONE', #21308, 18.00000000000000000 ) ;
#39461=ORIENTED_EDGE ( 'NONE', *, *, #2345, .T. ) ;
#39478=EDGE_CURVE ( 'NONE', #32551, #2390, #827, .T. ) ;
#39486=VERTEX_POINT ( 'NONE', #9756 ) ;
#39488=CARTESIAN_POINT ( 'NONE',  ( 2.118671991557230516, 37.17221401100731981, 12.00000000000000000 ) ) ;
#39490=AXIS2_PLACEMENT_3D ( 'NONE', #31072, #6472, #3831 ) ;
#39491=AXIS2_PLACEMENT_3D ( 'NONE', #26364, #38757, #22307 ) ;
#39493=CARTESIAN_POINT ( 'NONE',  ( -12.14717575287011719, 32.53695909538323860, 13.00000000000000178 ) ) ;
#39494=FACE_BOUND ( 'NONE', #31881, .T. ) ;
#39514=CARTESIAN_POINT ( 'NONE',  ( -11.14717575287011542, 32.53695909538323860, 13.00000000000000178 ) ) ;
#39516=LINE ( 'NONE', #5586, #11461 ) ;
#39526=DIRECTION ( 'NONE',  ( 0.000000000000000000, 0.000000000000000000, 1.000000000000000000 ) ) ;
#39532=DIRECTION ( 'NONE',  ( 1.000000000000000000, 0.000000000000000000, 0.000000000000000000 ) ) ;
#39534=ADVANCED_FACE ( 'NONE', ( #28834 ), #15849, .F. ) ;
#39536=DIRECTION ( 'NONE',  ( 0.000000000000000000, 0.000000000000000000, 1.000000000000000000 ) ) ;
#39540=CIRCLE ( 'NONE', #4516, 1.000000000000000000 ) ;
#39549=CARTESIAN_POINT ( 'NONE',  ( -11.14717575287011542, 32.53695909538323860, 6.000000000000000000 ) ) ;
#39570=FACE_OUTER_BOUND ( 'NONE', #41, .T. ) ;
#39574=AXIS2_PLACEMENT_3D ( 'NONE', #26209, #36364, #32723 ) ;
#39578=ADVANCED_FACE ( 'NONE', ( #31288 ), #31883, .F. ) ;
#39579=CARTESIAN_POINT ( 'NONE',  ( 0.3582258883630317636, 11.68927977431952137, 6.000000000000000000 ) ) ;
#39580=EDGE_CURVE ( 'NONE', #32493, #7288, #26755, .T. ) ;
#39589=CARTESIAN_POINT ( 'NONE',  ( 6.688300058587269170, 16.47782454277055564, 13.00000000000000178 ) ) ;
#39590=AXIS2_PLACEMENT_3D ( 'NONE', #39589, #11962, #5861 ) ;
#39591=CARTESIAN_POINT ( 'NONE',  ( 1.229431105722923023, 20.49260818092372460, 13.00000000000000178 ) ) ;
#39596=DIRECTION ( 'NONE',  ( 0.000000000000000000, 0.000000000000000000, 1.000000000000000000 ) ) ;
#39604=DIRECTION ( 'NONE',  ( 1.000000000000000000, 0.000000000000000000, 0.000000000000000000 ) ) ;
#39606=DIRECTION ( 'NONE',  ( 0.000000000000000000, 0.000000000000000000, 1.000000000000000000 ) ) ;
#39612=EDGE_LOOP ( 'NONE', ( #14158, #10242 ) ) ;
#39615=DIRECTION ( 'NONE',  ( 1.000000000000000000, 0.000000000000000000, 0.000000000000000000 ) ) ;
#39627=DIRECTION ( 'NONE',  ( 0.000000000000000000, 0.000000000000000000, 1.000000000000000000 ) ) ;
#39628=VERTEX_POINT ( 'NONE', #32833 ) ;
#39633=AXIS2_PLACEMENT_3D ( 'NONE', #25005, #3272, #6506 ) ;
#39637=DIRECTION ( 'NONE',  ( 0.000000000000000000, 0.000000000000000000, 1.000000000000000000 ) ) ;
#39640=CARTESIAN_POINT ( 'NONE',  ( 0.000000000000000000, 22.50000000000000355, 11.00000000000000178 ) ) ;
#39643=CIRCLE ( 'NONE', #26009, 1.000000000000000000 ) ;
#39654=ORIENTED_EDGE ( 'NONE', *, *, #1425, .T. ) ;
#39659=CARTESIAN_POINT ( 'NONE',  ( 2.494936919103933448, 34.23777120880591696, 13.00000000000000178 ) ) ;
#39663=EDGE_LOOP ( 'NONE', ( #37475, #8654, #36782, #3393 ) ) ;
#39667=DIRECTION ( 'NONE',  ( 0.000000000000000000, 0.000000000000000000, 1.000000000000000000 ) ) ;
#39668=ORIENTED_EDGE ( 'NONE', *, *, #31238, .T. ) ;
#39671=DIRECTION ( 'NONE',  ( 1.000000000000000000, 0.000000000000000000, 0.000000000000000000 ) ) ;
#39674=FACE_OUTER_BOUND ( 'NONE', #39711, .T. ) ;
#39680=ORIENTED_EDGE ( 'NONE', *, *, #32494, .F. ) ;
#39681=ADVANCED_FACE ( 'NONE', ( #23475 ), #8839, .F. ) ;
#39686=VERTEX_POINT ( 'NONE', #3134 ) ;
#39692=EDGE_CURVE ( 'NONE', #39920, #6629, #2806, .T. ) ;
#39707=CYLINDRICAL_SURFACE ( 'NONE', #1649, 1.000000000000000000 ) ;
#39711=EDGE_LOOP ( 'NONE', ( #13739, #16408, #12599, #35280 ) ) ;
#39716=CARTESIAN_POINT ( 'NONE',  ( 3.494936919103933448, 34.23777120880591696, 6.000000000000000000 ) ) ;
#39723=CARTESIAN_POINT ( 'NONE',  ( 5.953805871968278929, 30.22298757065274444, 6.000000000000000000 ) ) ;
#39735=CIRCLE ( 'NONE', #5347, 1.000000000000000000 ) ;
#39736=ORIENTED_EDGE ( 'NONE', *, *, #16325, .T. ) ;
#39741=CARTESIAN_POINT ( 'NONE',  ( 8.541469607472738090, 17.40487552589537401, 12.00000000000000000 ) ) ;
#39746=DIRECTION ( 'NONE',  ( 0.000000000000000000, 0.000000000000000000, 1.000000000000000000 ) ) ;
#39747=CARTESIAN_POINT ( 'NONE',  ( 0.000000000000000000, 22.50000000000000355, 12.00000000000000000 ) ) ;
#39751=AXIS2_PLACEMENT_3D ( 'NONE', #25228, #3493, #34774 ) ;
#39760=CARTESIAN_POINT ( 'NONE',  ( -9.165211421344535481, 24.66068167190384841, 6.000000000000000000 ) ) ;
#39763=VECTOR ( 'NONE', #2681, 1000.000000000000000 ) ;
#39773=EDGE_LOOP ( 'NONE', ( #23228, #25584, #21587, #12584 ) ) ;
#39774=CARTESIAN_POINT ( 'NONE',  ( 10.16520467992603294, 20.33931832809677331, 6.000000000000000000 ) ) ;
#39775=EDGE_CURVE ( 'NONE', #4988, #21746, #5382, .T. ) ;
#39790=FILL_AREA_STYLE_COLOUR ( '', #18410 ) ;
#39800=EDGE_CURVE ( 'NONE', #30063, #6257, #7992, .T. ) ;
#39801=STYLED_ITEM ( 'NONE', ( #36354 ), #3225 ) ;
#39811=ORIENTED_EDGE ( 'NONE', *, *, #14157, .T. ) ;
#39814=FACE_OUTER_BOUND ( 'NONE', #19166, .T. ) ;
#39815=CIRCLE ( 'NONE', #9977, 1.000000000000000000 ) ;
#39816=DIRECTION ( 'NONE',  ( 0.000000000000000000, 0.000000000000000000, 1.000000000000000000 ) ) ;
#39817=ORIENTED_EDGE ( 'NONE', *, *, #24791, .F. ) ;
#39820=CARTESIAN_POINT ( 'NONE',  ( -13.01838097023000707, 23.73363068877903359, 12.00000000000000000 ) ) ;
#39827=VECTOR ( 'NONE', #23319, 1000.000000000000000 ) ;
#39828=ORIENTED_EDGE ( 'NONE', *, *, #29697, .F. ) ;
#39833=VECTOR ( 'NONE', #17629, 1000.000000000000000 ) ;
#39837=CARTESIAN_POINT ( 'NONE',  ( -1.587667106213708879, 35.31811204475769728, 13.00000000000000178 ) ) ;
#39847=DIRECTION ( 'NONE',  ( 1.000000000000000000, 0.000000000000000000, 0.000000000000000000 ) ) ;
#39849=CIRCLE ( 'NONE', #26865, 1.000000000000000000 ) ;
#39854=DIRECTION ( 'NONE',  ( 0.000000000000000000, 0.000000000000000000, 1.000000000000000000 ) ) ;
#39855=EDGE_LOOP ( 'NONE', ( #17680, #34193, #15542, #5937 ) ) ;
#39856=ORIENTED_EDGE ( 'NONE', *, *, #23154, .F. ) ;
#39861=AXIS2_PLACEMENT_3D ( 'NONE', #2673, #20960, #3269 ) ;
#39865=DIRECTION ( 'NONE',  ( 1.000000000000000000, 0.000000000000000000, 0.000000000000000000 ) ) ;
#39881=DIRECTION ( 'NONE',  ( 1.000000000000000000, 0.000000000000000000, 0.000000000000000000 ) ) ;
#39885=FACE_BOUND ( 'NONE', #7418, .T. ) ;
#39887=EDGE_LOOP ( 'NONE', ( #33513, #5752 ) ) ;
#39890=CARTESIAN_POINT ( 'NONE',  ( 5.082600654608392610, 21.41965916404854298, 12.00000000000000000 ) ) ;
#39894=ADVANCED_FACE ( 'NONE', ( #25067 ), #3529, .F. ) ;
#39904=ORIENTED_EDGE ( 'NONE', *, *, #23908, .T. ) ;
#39908=FACE_OUTER_BOUND ( 'NONE', #32964, .T. ) ;
#39909=AXIS2_PLACEMENT_3D ( 'NONE', #23724, #10732, #11340 ) ;
#39916=DIRECTION ( 'NONE',  ( 0.000000000000000000, 0.000000000000000000, 1.000000000000000000 ) ) ;
#39919=VECTOR ( 'NONE', #30773, 1000.000000000000000 ) ;
#39920=VERTEX_POINT ( 'NONE', #22207 ) ;
#39922=EDGE_CURVE ( 'NONE', #37976, #39686, #26785, .T. ) ;
#39927=ADVANCED_FACE ( 'NONE', ( #2739 ), #12079, .F. ) ;
#39930=DIRECTION ( 'NONE',  ( 0.000000000000000000, 0.000000000000000000, 1.000000000000000000 ) ) ;
#39931=ADVANCED_FACE ( 'NONE', ( #26061 ), #682, .F. ) ;
#39939=DIRECTION ( 'NONE',  ( 0.000000000000000000, 0.000000000000000000, 1.000000000000000000 ) ) ;
#39942=CARTESIAN_POINT ( 'NONE',  ( -11.14717575287011542, 32.53695909538323860, 12.00000000000000000 ) ) ;
#39945=EDGE_CURVE ( 'NONE', #17659, #27275, #17729, .T. ) ;
#39950=CARTESIAN_POINT ( 'NONE',  ( 3.476901250629512941, 26.36149378532653031, 12.00000000000000000 ) ) ;
#39956=DIRECTION ( 'NONE',  ( 0.000000000000000000, 0.000000000000000000, 1.000000000000000000 ) ) ;
#39968=VERTEX_POINT ( 'NONE', #22814 ) ;
#39972=ORIENTED_EDGE ( 'NONE', *, *, #19850, .F. ) ;
#39973=EDGE_CURVE ( 'NONE', #8857, #12667, #37829, .T. ) ;
#39975=CARTESIAN_POINT ( 'NONE',  ( -10.18324708981896087, 16.78440424842446532, 13.00000000000000178 ) ) ;
#39976=AXIS2_PLACEMENT_3D ( 'NONE', #29867, #11392, #38611 ) ;
#39979=AXIS2_PLACEMENT_3D ( 'NONE', #17804, #23678, #29776 ) ;
#39994=ORIENTED_EDGE ( 'NONE', *, *, #4531, .T. ) ;
#39996=CARTESIAN_POINT ( 'NONE',  ( -0.3762682982559537037, 25.43444280220171194, 13.00000000000000178 ) ) ;
#39998=CARTESIAN_POINT ( 'NONE',  ( 0.000000000000000000, 22.50000000000000355, 12.00000000000000000 ) ) ;
#40001=AXIS2_PLACEMENT_3D ( 'NONE', #36977, #24978, #39615 ) ;
#40003=AXIS2_PLACEMENT_3D ( 'NONE', #20392, #17947, #32786 ) ;
#40007=ORIENTED_EDGE ( 'NONE', *, *, #19053, .T. ) ;
#40011=CARTESIAN_POINT ( 'NONE',  ( 8.917734535019441466, 14.47043272369397116, 13.00000000000000178 ) ) ;
#40022=ORIENTED_EDGE ( 'NONE', *, *, #25689, .F. ) ;
#40028=AXIS2_PLACEMENT_3D ( 'NONE', #3297, #37028, #3497 ) ;
#40032=( NAMED_UNIT ( * ) PLANE_ANGLE_UNIT ( ) SI_UNIT ( $, .RADIAN. ) );
#40036=CARTESIAN_POINT ( 'NONE',  ( 7.953805871968279817, 30.22298757065274444, 13.00000000000000178 ) ) ;
#40040=EDGE_CURVE ( 'NONE', #29140, #634, #196, .T. ) ;
#40044=DIRECTION ( 'NONE',  ( 0.000000000000000000, 0.000000000000000000, 1.000000000000000000 ) ) ;
#40045=CYLINDRICAL_SURFACE ( 'NONE', #32398, 1.000000000000000888 ) ;
#40046=VERTEX_POINT ( 'NONE', #29118 ) ;
#40051=LINE ( 'NONE', #5930, #12689 ) ;
#40052=ADVANCED_FACE ( 'NONE', ( #19775 ), #32169, .F. ) ;
#40053=VERTEX_POINT ( 'NONE', #23016 ) ;
#40054=ORIENTED_EDGE ( 'NONE', *, *, #21441, .T. ) ;
#40059=CIRCLE ( 'NONE', #12172, 1.000000000000000000 ) ;
#40064=EDGE_LOOP ( 'NONE', ( #34016, #22826, #10510, #2691 ) ) ;
#40069=ORIENTED_EDGE ( 'NONE', *, *, #15466, .T. ) ;
#40071=ORIENTED_EDGE ( 'NONE', *, *, #665, .F. ) ;
#40073=AXIS2_PLACEMENT_3D ( 'NONE', #3152, #15740, #27932 ) ;
#40077=VERTEX_POINT ( 'NONE', #3723 ) ;
#40085=AXIS2_PLACEMENT_3D ( 'NONE', #4296, #4501, #16696 ) ;
#40091=DIRECTION ( 'NONE',  ( 1.000000000000000000, 0.000000000000000000, 0.000000000000000000 ) ) ;
#40095=CARTESIAN_POINT ( 'NONE',  ( 1.587660364795204782, 9.681887955242936883, 13.00000000000000178 ) ) ;
#40101=CARTESIAN_POINT ( 'NONE',  ( -5.688306800005769048, 28.52217545723006609, 6.000000000000000000 ) ) ;
#40109=DIRECTION ( 'NONE',  ( 0.000000000000000000, 0.000000000000000000, 1.000000000000000000 ) ) ;
#40117=DIRECTION ( 'NONE',  ( 0.000000000000000000, 0.000000000000000000, 1.000000000000000000 ) ) ;
#40121=CIRCLE ( 'NONE', #22593, 1.000000000000000888 ) ;
#40123=CIRCLE ( 'NONE', #25844, 1.000000000000000000 ) ;
#40127=EDGE_CURVE ( 'NONE', #18785, #12475, #3067, .T. ) ;
#40132=CIRCLE ( 'NONE', #555, 1.000000000000000888 ) ;
#40137=LINE ( 'NONE', #24501, #15152 ) ;
#40144=EDGE_CURVE ( 'NONE', #2500, #7051, #28086, .T. ) ;
#40147=CARTESIAN_POINT ( 'NONE',  ( -2.853172919594720192, 21.57294901687549427, 12.00000000000000000 ) ) ;
#40152=LINE ( 'NONE', #3185, #2364 ) ;
#40159=ORIENTED_EDGE ( 'NONE', *, *, #29866, .T. ) ;
#40168=DIRECTION ( 'NONE',  ( -1.000000000000000000, 0.000000000000000000, 0.000000000000000000 ) ) ;
#40173=EDGE_LOOP ( 'NONE', ( #32699, #29400 ) ) ;
#40180=EDGE_CURVE ( 'NONE', #9757, #32909, #28249, .T. ) ;
#40181=ORIENTED_EDGE ( 'NONE', *, *, #33465, .T. ) ;
#40190=CARTESIAN_POINT ( 'NONE',  ( 0.3582258883630317636, 11.68927977431952137, 12.00000000000000000 ) ) ;
#40192=CARTESIAN_POINT ( 'NONE',  ( -11.16521142134453726, 24.66068167190384841, 6.000000000000000000 ) ) ;
ENDSEC;
END-ISO-10303-21;
